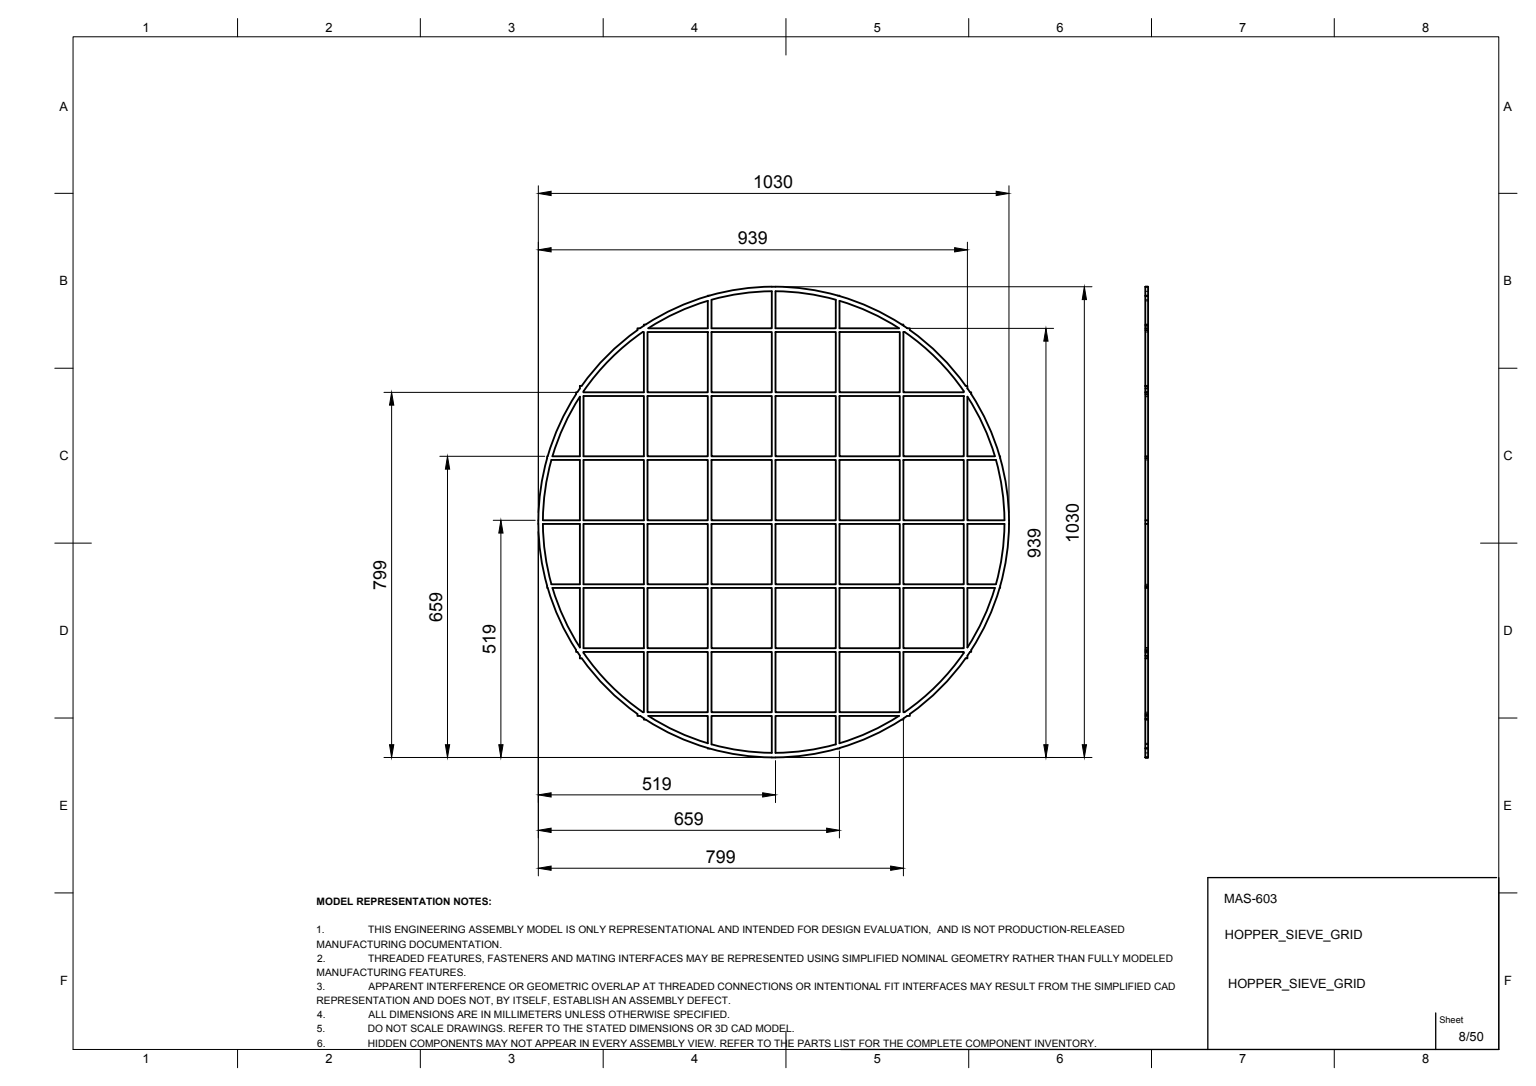
ISO-10303-21;
HEADER;
FILE_DESCRIPTION((''),'2;1');
FILE_NAME('HOPPER_SIEVE_GRID.step','2026-10-01T22:06:14-07:00',(''),(''),'','','');
FILE_SCHEMA (('AUTOMOTIVE_DESIGN { 1 0 10303 214 3 1 1 }'));
ENDSEC;
DATA;
#10=MECHANICAL_DESIGN_GEOMETRIC_PRESENTATION_REPRESENTATION('',(#984),#50440);
#894=SHAPE_REPRESENTATION_RELATIONSHIP('SRR','None',#50624,#939) ;
#939=ADVANCED_BREP_SHAPE_REPRESENTATION('',(#1040),#50393) ;
#984=STYLED_ITEM('',(#50885),#1040) ;
#1040=MANIFOLD_SOLID_BREP('HOPPER_SIEVE_GRID',#28632) ;
#1130=FACE_BOUND('',#4023,.T.) ;
#1131=FACE_BOUND('',#4024,.T.) ;
#1132=FACE_BOUND('',#4025,.T.) ;
#1133=FACE_BOUND('',#4026,.T.) ;
#1134=FACE_BOUND('',#4027,.T.) ;
#1135=FACE_BOUND('',#4028,.T.) ;
#1136=FACE_BOUND('',#4029,.T.) ;
#1137=FACE_BOUND('',#4030,.T.) ;
#1138=FACE_BOUND('',#4031,.T.) ;
#1139=FACE_BOUND('',#4032,.T.) ;
#1140=FACE_BOUND('',#4033,.T.) ;
#1141=FACE_BOUND('',#4034,.T.) ;
#1142=FACE_BOUND('',#4035,.T.) ;
#1143=FACE_BOUND('',#4036,.T.) ;
#1144=FACE_BOUND('',#4037,.T.) ;
#1145=FACE_BOUND('',#4038,.T.) ;
#1146=FACE_BOUND('',#4039,.T.) ;
#1147=FACE_BOUND('',#4040,.T.) ;
#1148=FACE_BOUND('',#4041,.T.) ;
#1149=FACE_BOUND('',#4042,.T.) ;
#1150=FACE_BOUND('',#4043,.T.) ;
#1151=FACE_BOUND('',#4044,.T.) ;
#1152=FACE_BOUND('',#4045,.T.) ;
#1153=FACE_BOUND('',#4046,.T.) ;
#1154=FACE_BOUND('',#4047,.T.) ;
#1155=FACE_BOUND('',#4048,.T.) ;
#1156=FACE_BOUND('',#4049,.T.) ;
#1157=FACE_BOUND('',#4050,.T.) ;
#1158=FACE_BOUND('',#4051,.T.) ;
#1159=FACE_BOUND('',#4052,.T.) ;
#1160=FACE_BOUND('',#4053,.T.) ;
#1161=FACE_BOUND('',#4054,.T.) ;
#1162=FACE_BOUND('',#4055,.T.) ;
#1163=FACE_BOUND('',#4056,.T.) ;
#1164=FACE_BOUND('',#4057,.T.) ;
#1165=FACE_BOUND('',#4058,.T.) ;
#1166=FACE_BOUND('',#4059,.T.) ;
#1167=FACE_BOUND('',#4060,.T.) ;
#1168=FACE_BOUND('',#4061,.T.) ;
#1169=FACE_BOUND('',#4062,.T.) ;
#1170=FACE_BOUND('',#4063,.T.) ;
#1171=FACE_BOUND('',#4064,.T.) ;
#1172=FACE_BOUND('',#4065,.T.) ;
#1173=FACE_BOUND('',#4066,.T.) ;
#1174=FACE_BOUND('',#4067,.T.) ;
#1175=FACE_BOUND('',#4068,.T.) ;
#1176=FACE_BOUND('',#4069,.T.) ;
#1177=FACE_BOUND('',#4070,.T.) ;
#1178=FACE_BOUND('',#4071,.T.) ;
#1179=FACE_BOUND('',#4072,.T.) ;
#1180=FACE_BOUND('',#4073,.T.) ;
#1181=FACE_BOUND('',#4074,.T.) ;
#1182=FACE_BOUND('',#4077,.T.) ;
#1183=FACE_BOUND('',#4078,.T.) ;
#1184=FACE_BOUND('',#4079,.T.) ;
#1185=FACE_BOUND('',#4080,.T.) ;
#1186=FACE_BOUND('',#4081,.T.) ;
#1187=FACE_BOUND('',#4082,.T.) ;
#1188=FACE_BOUND('',#4083,.T.) ;
#1189=FACE_BOUND('',#4084,.T.) ;
#1190=FACE_BOUND('',#4085,.T.) ;
#1191=FACE_BOUND('',#4086,.T.) ;
#1192=FACE_BOUND('',#4087,.T.) ;
#1193=FACE_BOUND('',#4088,.T.) ;
#1194=FACE_BOUND('',#4089,.T.) ;
#1195=FACE_BOUND('',#4090,.T.) ;
#1196=FACE_BOUND('',#4091,.T.) ;
#1197=FACE_BOUND('',#4092,.T.) ;
#1198=FACE_BOUND('',#4093,.T.) ;
#1199=FACE_BOUND('',#4094,.T.) ;
#1200=FACE_BOUND('',#4095,.T.) ;
#1201=FACE_BOUND('',#4096,.T.) ;
#1202=FACE_BOUND('',#4097,.T.) ;
#1203=FACE_BOUND('',#4098,.T.) ;
#1204=FACE_BOUND('',#4099,.T.) ;
#1205=FACE_BOUND('',#4100,.T.) ;
#1206=FACE_BOUND('',#4101,.T.) ;
#1207=FACE_BOUND('',#4102,.T.) ;
#1208=FACE_BOUND('',#4103,.T.) ;
#1209=FACE_BOUND('',#4104,.T.) ;
#1210=FACE_BOUND('',#4105,.T.) ;
#1211=FACE_BOUND('',#4106,.T.) ;
#1212=FACE_BOUND('',#4107,.T.) ;
#1213=FACE_BOUND('',#4108,.T.) ;
#1214=FACE_BOUND('',#4109,.T.) ;
#1215=FACE_BOUND('',#4110,.T.) ;
#1216=FACE_BOUND('',#4111,.T.) ;
#1217=FACE_BOUND('',#4112,.T.) ;
#1218=FACE_BOUND('',#4113,.T.) ;
#1219=FACE_BOUND('',#4114,.T.) ;
#1220=FACE_BOUND('',#4115,.T.) ;
#1221=FACE_BOUND('',#4116,.T.) ;
#1222=FACE_BOUND('',#4117,.T.) ;
#1223=FACE_BOUND('',#4118,.T.) ;
#1224=FACE_BOUND('',#4119,.T.) ;
#1225=FACE_BOUND('',#4120,.T.) ;
#1226=FACE_BOUND('',#4121,.T.) ;
#1227=FACE_BOUND('',#4122,.T.) ;
#1228=FACE_BOUND('',#4123,.T.) ;
#1229=FACE_BOUND('',#4124,.T.) ;
#1230=FACE_BOUND('',#4125,.T.) ;
#1231=FACE_BOUND('',#4126,.T.) ;
#1232=FACE_BOUND('',#4127,.T.) ;
#1233=FACE_BOUND('',#4128,.T.) ;
#1483=PLANE('',#29340) ;
#1484=PLANE('',#29341) ;
#1485=PLANE('',#29342) ;
#1486=PLANE('',#29343) ;
#1487=PLANE('',#29344) ;
#1488=PLANE('',#29345) ;
#1489=PLANE('',#29346) ;
#1490=PLANE('',#29347) ;
#1491=PLANE('',#29348) ;
#1492=PLANE('',#29349) ;
#1493=PLANE('',#29350) ;
#1494=PLANE('',#29351) ;
#1495=PLANE('',#29352) ;
#1496=PLANE('',#29353) ;
#1497=PLANE('',#29363) ;
#1498=PLANE('',#29364) ;
#1499=PLANE('',#29365) ;
#1500=PLANE('',#29366) ;
#1501=PLANE('',#29367) ;
#1502=PLANE('',#29368) ;
#1503=PLANE('',#29369) ;
#1504=PLANE('',#29370) ;
#1505=PLANE('',#29371) ;
#1506=PLANE('',#29419) ;
#1507=PLANE('',#29466) ;
#1508=PLANE('',#29467) ;
#1509=PLANE('',#29468) ;
#1510=PLANE('',#29469) ;
#1511=PLANE('',#29470) ;
#1512=PLANE('',#29471) ;
#1513=PLANE('',#29472) ;
#1514=PLANE('',#29473) ;
#1515=PLANE('',#29474) ;
#1516=PLANE('',#29475) ;
#1517=PLANE('',#29476) ;
#1518=PLANE('',#29477) ;
#1519=PLANE('',#29478) ;
#1520=PLANE('',#29479) ;
#1521=PLANE('',#29480) ;
#1522=PLANE('',#29481) ;
#1523=PLANE('',#29482) ;
#1524=PLANE('',#29485) ;
#1525=PLANE('',#29486) ;
#1526=PLANE('',#29487) ;
#1527=PLANE('',#29488) ;
#1528=PLANE('',#29489) ;
#1529=PLANE('',#29493) ;
#1530=PLANE('',#29494) ;
#1531=PLANE('',#29495) ;
#1532=PLANE('',#29496) ;
#1533=PLANE('',#29497) ;
#1534=PLANE('',#29498) ;
#1535=PLANE('',#29499) ;
#1536=PLANE('',#29500) ;
#1537=PLANE('',#29501) ;
#1538=PLANE('',#29502) ;
#1539=PLANE('',#29503) ;
#1540=PLANE('',#29504) ;
#1541=PLANE('',#29505) ;
#1542=PLANE('',#29506) ;
#1543=PLANE('',#29507) ;
#1544=PLANE('',#29508) ;
#1545=PLANE('',#29509) ;
#1546=PLANE('',#29511) ;
#1547=PLANE('',#29512) ;
#1548=PLANE('',#29513) ;
#1549=PLANE('',#29514) ;
#1550=PLANE('',#29515) ;
#1551=PLANE('',#29516) ;
#1552=PLANE('',#29517) ;
#1553=PLANE('',#29518) ;
#1554=PLANE('',#29520) ;
#1555=PLANE('',#29521) ;
#1556=PLANE('',#29522) ;
#1557=PLANE('',#29523) ;
#1558=PLANE('',#29524) ;
#1559=PLANE('',#29525) ;
#1560=PLANE('',#29526) ;
#1561=PLANE('',#29527) ;
#1562=PLANE('',#29528) ;
#1563=PLANE('',#29529) ;
#1564=PLANE('',#29530) ;
#1565=PLANE('',#29531) ;
#1566=PLANE('',#29532) ;
#1567=PLANE('',#29533) ;
#1568=PLANE('',#29534) ;
#1569=PLANE('',#29535) ;
#1570=PLANE('',#29536) ;
#1571=PLANE('',#29537) ;
#1572=PLANE('',#29538) ;
#1573=PLANE('',#29541) ;
#1574=PLANE('',#29544) ;
#1575=PLANE('',#29545) ;
#1576=PLANE('',#29546) ;
#1577=PLANE('',#29547) ;
#1578=PLANE('',#29548) ;
#1579=PLANE('',#29549) ;
#1580=PLANE('',#29550) ;
#1581=PLANE('',#29551) ;
#1582=PLANE('',#29552) ;
#1583=PLANE('',#29553) ;
#1584=PLANE('',#29554) ;
#1585=PLANE('',#29555) ;
#1586=PLANE('',#29556) ;
#1587=PLANE('',#29557) ;
#1588=PLANE('',#29558) ;
#1589=PLANE('',#29559) ;
#1590=PLANE('',#29560) ;
#1591=PLANE('',#29561) ;
#1592=PLANE('',#29562) ;
#1593=PLANE('',#29563) ;
#1594=PLANE('',#29564) ;
#1595=PLANE('',#29565) ;
#1596=PLANE('',#29570) ;
#1597=PLANE('',#29571) ;
#1598=PLANE('',#29572) ;
#1599=PLANE('',#29573) ;
#1600=PLANE('',#29574) ;
#1601=PLANE('',#29575) ;
#1602=PLANE('',#29576) ;
#1603=PLANE('',#29577) ;
#1604=PLANE('',#29578) ;
#1605=PLANE('',#29579) ;
#1606=PLANE('',#29580) ;
#1607=PLANE('',#29581) ;
#1608=PLANE('',#29582) ;
#1609=PLANE('',#29583) ;
#1610=PLANE('',#29584) ;
#1611=PLANE('',#29585) ;
#1612=PLANE('',#29586) ;
#1613=PLANE('',#29587) ;
#1614=PLANE('',#29588) ;
#1615=PLANE('',#29589) ;
#1616=PLANE('',#29590) ;
#1617=PLANE('',#29591) ;
#1618=PLANE('',#29592) ;
#1619=PLANE('',#29593) ;
#1620=PLANE('',#29597) ;
#1621=PLANE('',#29598) ;
#1622=PLANE('',#29599) ;
#1623=PLANE('',#29600) ;
#1624=PLANE('',#29601) ;
#1625=PLANE('',#29602) ;
#1626=PLANE('',#29605) ;
#1627=PLANE('',#29606) ;
#1628=PLANE('',#29607) ;
#1629=PLANE('',#29608) ;
#1630=PLANE('',#29609) ;
#1631=PLANE('',#29610) ;
#1632=PLANE('',#29611) ;
#1633=PLANE('',#29612) ;
#1634=PLANE('',#29613) ;
#1635=PLANE('',#29614) ;
#1636=PLANE('',#29615) ;
#1637=PLANE('',#29616) ;
#1638=PLANE('',#29617) ;
#1639=PLANE('',#29618) ;
#1640=PLANE('',#29619) ;
#1641=PLANE('',#29620) ;
#1642=PLANE('',#29621) ;
#1643=PLANE('',#29622) ;
#1644=PLANE('',#29625) ;
#1645=PLANE('',#29626) ;
#1646=PLANE('',#29630) ;
#1647=PLANE('',#29631) ;
#1648=PLANE('',#29632) ;
#1649=PLANE('',#29633) ;
#1650=PLANE('',#29634) ;
#1651=PLANE('',#29635) ;
#1652=PLANE('',#29636) ;
#1653=PLANE('',#29637) ;
#1654=PLANE('',#29638) ;
#1655=PLANE('',#29639) ;
#1656=PLANE('',#29640) ;
#1657=PLANE('',#29641) ;
#1658=PLANE('',#29642) ;
#1659=PLANE('',#29643) ;
#1660=PLANE('',#29644) ;
#1661=PLANE('',#29645) ;
#1662=PLANE('',#29646) ;
#1663=PLANE('',#29647) ;
#1664=PLANE('',#29648) ;
#1665=PLANE('',#29649) ;
#1666=PLANE('',#29650) ;
#1667=PLANE('',#29651) ;
#1668=PLANE('',#29653) ;
#1669=PLANE('',#29654) ;
#1670=PLANE('',#29658) ;
#1671=PLANE('',#29659) ;
#1672=PLANE('',#29660) ;
#1673=PLANE('',#29661) ;
#1674=PLANE('',#29662) ;
#1675=PLANE('',#29663) ;
#1676=PLANE('',#29664) ;
#1677=PLANE('',#29665) ;
#1678=PLANE('',#29666) ;
#1679=PLANE('',#29667) ;
#1680=PLANE('',#29668) ;
#1681=PLANE('',#29669) ;
#1682=PLANE('',#29670) ;
#1683=PLANE('',#29671) ;
#1684=PLANE('',#29672) ;
#1685=PLANE('',#29673) ;
#1686=PLANE('',#29675) ;
#1687=PLANE('',#29676) ;
#1688=PLANE('',#29679) ;
#1689=PLANE('',#29680) ;
#1690=PLANE('',#29681) ;
#1691=PLANE('',#29682) ;
#1692=PLANE('',#29683) ;
#1693=PLANE('',#29684) ;
#1694=PLANE('',#29685) ;
#1695=PLANE('',#29686) ;
#1696=PLANE('',#29687) ;
#1697=PLANE('',#29688) ;
#1698=PLANE('',#29689) ;
#1699=PLANE('',#29693) ;
#1700=PLANE('',#29694) ;
#1701=PLANE('',#29697) ;
#1702=PLANE('',#29698) ;
#1703=PLANE('',#29699) ;
#1704=PLANE('',#29700) ;
#1705=PLANE('',#29701) ;
#1706=PLANE('',#29702) ;
#1707=PLANE('',#29703) ;
#1708=PLANE('',#29704) ;
#1709=PLANE('',#29705) ;
#1710=PLANE('',#29707) ;
#1711=PLANE('',#29709) ;
#1712=PLANE('',#29710) ;
#1713=PLANE('',#29711) ;
#1714=PLANE('',#29712) ;
#1715=PLANE('',#29713) ;
#1716=PLANE('',#29714) ;
#1717=PLANE('',#29715) ;
#1718=PLANE('',#29717) ;
#1719=PLANE('',#29718) ;
#1720=PLANE('',#29719) ;
#1721=PLANE('',#29720) ;
#1722=PLANE('',#29721) ;
#1723=PLANE('',#29724) ;
#1724=PLANE('',#29725) ;
#1725=PLANE('',#29726) ;
#1726=PLANE('',#29727) ;
#1727=PLANE('',#29728) ;
#1728=PLANE('',#29729) ;
#2425=FACE_OUTER_BOUND('',#3997,.T.) ;
#2426=FACE_OUTER_BOUND('',#3998,.T.) ;
#2427=FACE_OUTER_BOUND('',#3999,.T.) ;
#2428=FACE_OUTER_BOUND('',#4000,.T.) ;
#2429=FACE_OUTER_BOUND('',#4001,.T.) ;
#2430=FACE_OUTER_BOUND('',#4002,.T.) ;
#2431=FACE_OUTER_BOUND('',#4003,.T.) ;
#2432=FACE_OUTER_BOUND('',#4004,.T.) ;
#2433=FACE_OUTER_BOUND('',#4005,.T.) ;
#2434=FACE_OUTER_BOUND('',#4006,.T.) ;
#2435=FACE_OUTER_BOUND('',#4007,.T.) ;
#2436=FACE_OUTER_BOUND('',#4008,.T.) ;
#2437=FACE_OUTER_BOUND('',#4009,.T.) ;
#2438=FACE_OUTER_BOUND('',#4010,.T.) ;
#2439=FACE_OUTER_BOUND('',#4011,.T.) ;
#2440=FACE_OUTER_BOUND('',#4012,.T.) ;
#2441=FACE_OUTER_BOUND('',#4013,.T.) ;
#2442=FACE_OUTER_BOUND('',#4014,.T.) ;
#2443=FACE_OUTER_BOUND('',#4015,.T.) ;
#2444=FACE_OUTER_BOUND('',#4016,.T.) ;
#2445=FACE_OUTER_BOUND('',#4017,.T.) ;
#2446=FACE_OUTER_BOUND('',#4018,.T.) ;
#2447=FACE_OUTER_BOUND('',#4019,.T.) ;
#2448=FACE_OUTER_BOUND('',#4020,.T.) ;
#2449=FACE_OUTER_BOUND('',#4021,.T.) ;
#2450=FACE_OUTER_BOUND('',#4022,.T.) ;
#2451=FACE_OUTER_BOUND('',#4075,.T.) ;
#2452=FACE_OUTER_BOUND('',#4076,.T.) ;
#2453=FACE_OUTER_BOUND('',#4129,.T.) ;
#2454=FACE_OUTER_BOUND('',#4130,.T.) ;
#2455=FACE_OUTER_BOUND('',#4131,.T.) ;
#2456=FACE_OUTER_BOUND('',#4132,.T.) ;
#2457=FACE_OUTER_BOUND('',#4133,.T.) ;
#2458=FACE_OUTER_BOUND('',#4134,.T.) ;
#2459=FACE_OUTER_BOUND('',#4135,.T.) ;
#2460=FACE_OUTER_BOUND('',#4136,.T.) ;
#2461=FACE_OUTER_BOUND('',#4137,.T.) ;
#2462=FACE_OUTER_BOUND('',#4138,.T.) ;
#2463=FACE_OUTER_BOUND('',#4139,.T.) ;
#2464=FACE_OUTER_BOUND('',#4140,.T.) ;
#2465=FACE_OUTER_BOUND('',#4141,.T.) ;
#2466=FACE_OUTER_BOUND('',#4142,.T.) ;
#2467=FACE_OUTER_BOUND('',#4143,.T.) ;
#2468=FACE_OUTER_BOUND('',#4144,.T.) ;
#2469=FACE_OUTER_BOUND('',#4145,.T.) ;
#2470=FACE_OUTER_BOUND('',#4146,.T.) ;
#2471=FACE_OUTER_BOUND('',#4147,.T.) ;
#2472=FACE_OUTER_BOUND('',#4148,.T.) ;
#2473=FACE_OUTER_BOUND('',#4149,.T.) ;
#2474=FACE_OUTER_BOUND('',#4150,.T.) ;
#2475=FACE_OUTER_BOUND('',#4151,.T.) ;
#2476=FACE_OUTER_BOUND('',#4152,.T.) ;
#2477=FACE_OUTER_BOUND('',#4153,.T.) ;
#2478=FACE_OUTER_BOUND('',#4154,.T.) ;
#2479=FACE_OUTER_BOUND('',#4155,.T.) ;
#2480=FACE_OUTER_BOUND('',#4156,.T.) ;
#2481=FACE_OUTER_BOUND('',#4157,.T.) ;
#2482=FACE_OUTER_BOUND('',#4158,.T.) ;
#2483=FACE_OUTER_BOUND('',#4159,.T.) ;
#2484=FACE_OUTER_BOUND('',#4160,.T.) ;
#2485=FACE_OUTER_BOUND('',#4161,.T.) ;
#2486=FACE_OUTER_BOUND('',#4162,.T.) ;
#2487=FACE_OUTER_BOUND('',#4163,.T.) ;
#2488=FACE_OUTER_BOUND('',#4164,.T.) ;
#2489=FACE_OUTER_BOUND('',#4165,.T.) ;
#2490=FACE_OUTER_BOUND('',#4166,.T.) ;
#2491=FACE_OUTER_BOUND('',#4167,.T.) ;
#2492=FACE_OUTER_BOUND('',#4168,.T.) ;
#2493=FACE_OUTER_BOUND('',#4169,.T.) ;
#2494=FACE_OUTER_BOUND('',#4170,.T.) ;
#2495=FACE_OUTER_BOUND('',#4171,.T.) ;
#2496=FACE_OUTER_BOUND('',#4172,.T.) ;
#2497=FACE_OUTER_BOUND('',#4173,.T.) ;
#2498=FACE_OUTER_BOUND('',#4174,.T.) ;
#2499=FACE_OUTER_BOUND('',#4175,.T.) ;
#2500=FACE_OUTER_BOUND('',#4176,.T.) ;
#2501=FACE_OUTER_BOUND('',#4177,.T.) ;
#2502=FACE_OUTER_BOUND('',#4178,.T.) ;
#2503=FACE_OUTER_BOUND('',#4179,.T.) ;
#2504=FACE_OUTER_BOUND('',#4180,.T.) ;
#2505=FACE_OUTER_BOUND('',#4181,.T.) ;
#2506=FACE_OUTER_BOUND('',#4182,.T.) ;
#2507=FACE_OUTER_BOUND('',#4183,.T.) ;
#2508=FACE_OUTER_BOUND('',#4184,.T.) ;
#2509=FACE_OUTER_BOUND('',#4185,.T.) ;
#2510=FACE_OUTER_BOUND('',#4186,.T.) ;
#2511=FACE_OUTER_BOUND('',#4187,.T.) ;
#2512=FACE_OUTER_BOUND('',#4188,.T.) ;
#2513=FACE_OUTER_BOUND('',#4189,.T.) ;
#2514=FACE_OUTER_BOUND('',#4190,.T.) ;
#2515=FACE_OUTER_BOUND('',#4191,.T.) ;
#2516=FACE_OUTER_BOUND('',#4192,.T.) ;
#2517=FACE_OUTER_BOUND('',#4193,.T.) ;
#2518=FACE_OUTER_BOUND('',#4194,.T.) ;
#2519=FACE_OUTER_BOUND('',#4195,.T.) ;
#2520=FACE_OUTER_BOUND('',#4196,.T.) ;
#2521=FACE_OUTER_BOUND('',#4197,.T.) ;
#2522=FACE_OUTER_BOUND('',#4198,.T.) ;
#2523=FACE_OUTER_BOUND('',#4199,.T.) ;
#2524=FACE_OUTER_BOUND('',#4200,.T.) ;
#2525=FACE_OUTER_BOUND('',#4201,.T.) ;
#2526=FACE_OUTER_BOUND('',#4202,.T.) ;
#2527=FACE_OUTER_BOUND('',#4203,.T.) ;
#2528=FACE_OUTER_BOUND('',#4204,.T.) ;
#2529=FACE_OUTER_BOUND('',#4205,.T.) ;
#2530=FACE_OUTER_BOUND('',#4206,.T.) ;
#2531=FACE_OUTER_BOUND('',#4207,.T.) ;
#2532=FACE_OUTER_BOUND('',#4208,.T.) ;
#2533=FACE_OUTER_BOUND('',#4209,.T.) ;
#2534=FACE_OUTER_BOUND('',#4210,.T.) ;
#2535=FACE_OUTER_BOUND('',#4211,.T.) ;
#2536=FACE_OUTER_BOUND('',#4212,.T.) ;
#2537=FACE_OUTER_BOUND('',#4213,.T.) ;
#2538=FACE_OUTER_BOUND('',#4214,.T.) ;
#2539=FACE_OUTER_BOUND('',#4215,.T.) ;
#2540=FACE_OUTER_BOUND('',#4216,.T.) ;
#2541=FACE_OUTER_BOUND('',#4217,.T.) ;
#2542=FACE_OUTER_BOUND('',#4218,.T.) ;
#2543=FACE_OUTER_BOUND('',#4219,.T.) ;
#2544=FACE_OUTER_BOUND('',#4220,.T.) ;
#2545=FACE_OUTER_BOUND('',#4221,.T.) ;
#2546=FACE_OUTER_BOUND('',#4222,.T.) ;
#2547=FACE_OUTER_BOUND('',#4223,.T.) ;
#2548=FACE_OUTER_BOUND('',#4224,.T.) ;
#2549=FACE_OUTER_BOUND('',#4225,.T.) ;
#2550=FACE_OUTER_BOUND('',#4226,.T.) ;
#2551=FACE_OUTER_BOUND('',#4227,.T.) ;
#2552=FACE_OUTER_BOUND('',#4228,.T.) ;
#2553=FACE_OUTER_BOUND('',#4229,.T.) ;
#2554=FACE_OUTER_BOUND('',#4230,.T.) ;
#2555=FACE_OUTER_BOUND('',#4231,.T.) ;
#2556=FACE_OUTER_BOUND('',#4232,.T.) ;
#2557=FACE_OUTER_BOUND('',#4233,.T.) ;
#2558=FACE_OUTER_BOUND('',#4234,.T.) ;
#2559=FACE_OUTER_BOUND('',#4235,.T.) ;
#2560=FACE_OUTER_BOUND('',#4236,.T.) ;
#2561=FACE_OUTER_BOUND('',#4237,.T.) ;
#2562=FACE_OUTER_BOUND('',#4238,.T.) ;
#2563=FACE_OUTER_BOUND('',#4239,.T.) ;
#2564=FACE_OUTER_BOUND('',#4240,.T.) ;
#2565=FACE_OUTER_BOUND('',#4241,.T.) ;
#2566=FACE_OUTER_BOUND('',#4242,.T.) ;
#2567=FACE_OUTER_BOUND('',#4243,.T.) ;
#2568=FACE_OUTER_BOUND('',#4244,.T.) ;
#2569=FACE_OUTER_BOUND('',#4245,.T.) ;
#2570=FACE_OUTER_BOUND('',#4246,.T.) ;
#2571=FACE_OUTER_BOUND('',#4247,.T.) ;
#2572=FACE_OUTER_BOUND('',#4248,.T.) ;
#2573=FACE_OUTER_BOUND('',#4249,.T.) ;
#2574=FACE_OUTER_BOUND('',#4250,.T.) ;
#2575=FACE_OUTER_BOUND('',#4251,.T.) ;
#2576=FACE_OUTER_BOUND('',#4252,.T.) ;
#2577=FACE_OUTER_BOUND('',#4253,.T.) ;
#2578=FACE_OUTER_BOUND('',#4254,.T.) ;
#2579=FACE_OUTER_BOUND('',#4255,.T.) ;
#2580=FACE_OUTER_BOUND('',#4256,.T.) ;
#2581=FACE_OUTER_BOUND('',#4257,.T.) ;
#2582=FACE_OUTER_BOUND('',#4258,.T.) ;
#2583=FACE_OUTER_BOUND('',#4259,.T.) ;
#2584=FACE_OUTER_BOUND('',#4260,.T.) ;
#2585=FACE_OUTER_BOUND('',#4261,.T.) ;
#2586=FACE_OUTER_BOUND('',#4262,.T.) ;
#2587=FACE_OUTER_BOUND('',#4263,.T.) ;
#2588=FACE_OUTER_BOUND('',#4264,.T.) ;
#2589=FACE_OUTER_BOUND('',#4265,.T.) ;
#2590=FACE_OUTER_BOUND('',#4266,.T.) ;
#2591=FACE_OUTER_BOUND('',#4267,.T.) ;
#2592=FACE_OUTER_BOUND('',#4268,.T.) ;
#2593=FACE_OUTER_BOUND('',#4269,.T.) ;
#2594=FACE_OUTER_BOUND('',#4270,.T.) ;
#2595=FACE_OUTER_BOUND('',#4271,.T.) ;
#2596=FACE_OUTER_BOUND('',#4272,.T.) ;
#2597=FACE_OUTER_BOUND('',#4273,.T.) ;
#2598=FACE_OUTER_BOUND('',#4274,.T.) ;
#2599=FACE_OUTER_BOUND('',#4275,.T.) ;
#2600=FACE_OUTER_BOUND('',#4276,.T.) ;
#2601=FACE_OUTER_BOUND('',#4277,.T.) ;
#2602=FACE_OUTER_BOUND('',#4278,.T.) ;
#2603=FACE_OUTER_BOUND('',#4279,.T.) ;
#2604=FACE_OUTER_BOUND('',#4280,.T.) ;
#2605=FACE_OUTER_BOUND('',#4281,.T.) ;
#2606=FACE_OUTER_BOUND('',#4282,.T.) ;
#2607=FACE_OUTER_BOUND('',#4283,.T.) ;
#2608=FACE_OUTER_BOUND('',#4284,.T.) ;
#2609=FACE_OUTER_BOUND('',#4285,.T.) ;
#2610=FACE_OUTER_BOUND('',#4286,.T.) ;
#2611=FACE_OUTER_BOUND('',#4287,.T.) ;
#2612=FACE_OUTER_BOUND('',#4288,.T.) ;
#2613=FACE_OUTER_BOUND('',#4289,.T.) ;
#2614=FACE_OUTER_BOUND('',#4290,.T.) ;
#2615=FACE_OUTER_BOUND('',#4291,.T.) ;
#2616=FACE_OUTER_BOUND('',#4292,.T.) ;
#2617=FACE_OUTER_BOUND('',#4293,.T.) ;
#2618=FACE_OUTER_BOUND('',#4294,.T.) ;
#2619=FACE_OUTER_BOUND('',#4295,.T.) ;
#2620=FACE_OUTER_BOUND('',#4296,.T.) ;
#2621=FACE_OUTER_BOUND('',#4297,.T.) ;
#2622=FACE_OUTER_BOUND('',#4298,.T.) ;
#2623=FACE_OUTER_BOUND('',#4299,.T.) ;
#2624=FACE_OUTER_BOUND('',#4300,.T.) ;
#2625=FACE_OUTER_BOUND('',#4301,.T.) ;
#2626=FACE_OUTER_BOUND('',#4302,.T.) ;
#2627=FACE_OUTER_BOUND('',#4303,.T.) ;
#2628=FACE_OUTER_BOUND('',#4304,.T.) ;
#2629=FACE_OUTER_BOUND('',#4305,.T.) ;
#2630=FACE_OUTER_BOUND('',#4306,.T.) ;
#2631=FACE_OUTER_BOUND('',#4307,.T.) ;
#2632=FACE_OUTER_BOUND('',#4308,.T.) ;
#2633=FACE_OUTER_BOUND('',#4309,.T.) ;
#2634=FACE_OUTER_BOUND('',#4310,.T.) ;
#2635=FACE_OUTER_BOUND('',#4311,.T.) ;
#2636=FACE_OUTER_BOUND('',#4312,.T.) ;
#2637=FACE_OUTER_BOUND('',#4313,.T.) ;
#2638=FACE_OUTER_BOUND('',#4314,.T.) ;
#2639=FACE_OUTER_BOUND('',#4315,.T.) ;
#2640=FACE_OUTER_BOUND('',#4316,.T.) ;
#2641=FACE_OUTER_BOUND('',#4317,.T.) ;
#2642=FACE_OUTER_BOUND('',#4318,.T.) ;
#2643=FACE_OUTER_BOUND('',#4319,.T.) ;
#2644=FACE_OUTER_BOUND('',#4320,.T.) ;
#2645=FACE_OUTER_BOUND('',#4321,.T.) ;
#2646=FACE_OUTER_BOUND('',#4322,.T.) ;
#2647=FACE_OUTER_BOUND('',#4323,.T.) ;
#2648=FACE_OUTER_BOUND('',#4324,.T.) ;
#2649=FACE_OUTER_BOUND('',#4325,.T.) ;
#2650=FACE_OUTER_BOUND('',#4326,.T.) ;
#2651=FACE_OUTER_BOUND('',#4327,.T.) ;
#2652=FACE_OUTER_BOUND('',#4328,.T.) ;
#2653=FACE_OUTER_BOUND('',#4329,.T.) ;
#2654=FACE_OUTER_BOUND('',#4330,.T.) ;
#2655=FACE_OUTER_BOUND('',#4331,.T.) ;
#2656=FACE_OUTER_BOUND('',#4332,.T.) ;
#2657=FACE_OUTER_BOUND('',#4333,.T.) ;
#2658=FACE_OUTER_BOUND('',#4334,.T.) ;
#2659=FACE_OUTER_BOUND('',#4335,.T.) ;
#2660=FACE_OUTER_BOUND('',#4336,.T.) ;
#2661=FACE_OUTER_BOUND('',#4337,.T.) ;
#2662=FACE_OUTER_BOUND('',#4338,.T.) ;
#2663=FACE_OUTER_BOUND('',#4339,.T.) ;
#2664=FACE_OUTER_BOUND('',#4340,.T.) ;
#2665=FACE_OUTER_BOUND('',#4341,.T.) ;
#2666=FACE_OUTER_BOUND('',#4342,.T.) ;
#2667=FACE_OUTER_BOUND('',#4343,.T.) ;
#2668=FACE_OUTER_BOUND('',#4344,.T.) ;
#2669=FACE_OUTER_BOUND('',#4345,.T.) ;
#2670=FACE_OUTER_BOUND('',#4346,.T.) ;
#2671=FACE_OUTER_BOUND('',#4347,.T.) ;
#2672=FACE_OUTER_BOUND('',#4348,.T.) ;
#2673=FACE_OUTER_BOUND('',#4349,.T.) ;
#2674=FACE_OUTER_BOUND('',#4350,.T.) ;
#2675=FACE_OUTER_BOUND('',#4351,.T.) ;
#2676=FACE_OUTER_BOUND('',#4352,.T.) ;
#2677=FACE_OUTER_BOUND('',#4353,.T.) ;
#2678=FACE_OUTER_BOUND('',#4354,.T.) ;
#2679=FACE_OUTER_BOUND('',#4355,.T.) ;
#2680=FACE_OUTER_BOUND('',#4356,.T.) ;
#2681=FACE_OUTER_BOUND('',#4357,.T.) ;
#2682=FACE_OUTER_BOUND('',#4358,.T.) ;
#2683=FACE_OUTER_BOUND('',#4359,.T.) ;
#2684=FACE_OUTER_BOUND('',#4360,.T.) ;
#2685=FACE_OUTER_BOUND('',#4361,.T.) ;
#2686=FACE_OUTER_BOUND('',#4362,.T.) ;
#2687=FACE_OUTER_BOUND('',#4363,.T.) ;
#2688=FACE_OUTER_BOUND('',#4364,.T.) ;
#2689=FACE_OUTER_BOUND('',#4365,.T.) ;
#2690=FACE_OUTER_BOUND('',#4366,.T.) ;
#2691=FACE_OUTER_BOUND('',#4367,.T.) ;
#2692=FACE_OUTER_BOUND('',#4368,.T.) ;
#2693=FACE_OUTER_BOUND('',#4369,.T.) ;
#2694=FACE_OUTER_BOUND('',#4370,.T.) ;
#2695=FACE_OUTER_BOUND('',#4371,.T.) ;
#2696=FACE_OUTER_BOUND('',#4372,.T.) ;
#2697=FACE_OUTER_BOUND('',#4373,.T.) ;
#2698=FACE_OUTER_BOUND('',#4374,.T.) ;
#2699=FACE_OUTER_BOUND('',#4375,.T.) ;
#2700=FACE_OUTER_BOUND('',#4376,.T.) ;
#2701=FACE_OUTER_BOUND('',#4377,.T.) ;
#2702=FACE_OUTER_BOUND('',#4378,.T.) ;
#2703=FACE_OUTER_BOUND('',#4379,.T.) ;
#2704=FACE_OUTER_BOUND('',#4380,.T.) ;
#2705=FACE_OUTER_BOUND('',#4381,.T.) ;
#2706=FACE_OUTER_BOUND('',#4382,.T.) ;
#2707=FACE_OUTER_BOUND('',#4383,.T.) ;
#2708=FACE_OUTER_BOUND('',#4384,.T.) ;
#2709=FACE_OUTER_BOUND('',#4385,.T.) ;
#2710=FACE_OUTER_BOUND('',#4386,.T.) ;
#2711=FACE_OUTER_BOUND('',#4387,.T.) ;
#2712=FACE_OUTER_BOUND('',#4388,.T.) ;
#2713=FACE_OUTER_BOUND('',#4389,.T.) ;
#2714=FACE_OUTER_BOUND('',#4390,.T.) ;
#2715=FACE_OUTER_BOUND('',#4391,.T.) ;
#2716=FACE_OUTER_BOUND('',#4392,.T.) ;
#2717=FACE_OUTER_BOUND('',#4393,.T.) ;
#2718=FACE_OUTER_BOUND('',#4394,.T.) ;
#3997=EDGE_LOOP('',(#19001,#19002,#19003,#19004)) ;
#3998=EDGE_LOOP('',(#19005,#19006,#19007,#19008)) ;
#3999=EDGE_LOOP('',(#19009,#19010,#19011,#19012)) ;
#4000=EDGE_LOOP('',(#19013,#19014,#19015,#19016)) ;
#4001=EDGE_LOOP('',(#19017,#19018,#19019,#19020)) ;
#4002=EDGE_LOOP('',(#19021,#19022,#19023,#19024)) ;
#4003=EDGE_LOOP('',(#19025,#19026,#19027,#19028)) ;
#4004=EDGE_LOOP('',(#19029,#19030,#19031,#19032)) ;
#4005=EDGE_LOOP('',(#19033,#19034,#19035,#19036)) ;
#4006=EDGE_LOOP('',(#19037,#19038,#19039,#19040)) ;
#4007=EDGE_LOOP('',(#19041,#19042,#19043,#19044)) ;
#4008=EDGE_LOOP('',(#19045,#19046,#19047,#19048)) ;
#4009=EDGE_LOOP('',(#19049,#19050,#19051,#19052)) ;
#4010=EDGE_LOOP('',(#19053,#19054,#19055,#19056)) ;
#4011=EDGE_LOOP('',(#19057,#19058,#19059,#19060)) ;
#4012=EDGE_LOOP('',(#19061,#19062,#19063,#19064)) ;
#4013=EDGE_LOOP('',(#19065,#19066,#19067,#19068)) ;
#4014=EDGE_LOOP('',(#19069,#19070,#19071,#19072)) ;
#4015=EDGE_LOOP('',(#19073,#19074,#19075,#19076)) ;
#4016=EDGE_LOOP('',(#19077,#19078,#19079,#19080)) ;
#4017=EDGE_LOOP('',(#19081,#19082,#19083,#19084)) ;
#4018=EDGE_LOOP('',(#19085,#19086,#19087,#19088)) ;
#4019=EDGE_LOOP('',(#19089,#19090,#19091,#19092)) ;
#4020=EDGE_LOOP('',(#19093,#19094,#19095,#19096)) ;
#4021=EDGE_LOOP('',(#19097,#19098,#19099,#19100)) ;
#4022=EDGE_LOOP('',(#19101,#19102,#19103,#19104,#19105,#19106,#19107,#19108,
#19109,#19110,#19111,#19112,#19113,#19114,#19115,#19116,#19117,#19118,#19119,
#19120,#19121,#19122,#19123,#19124,#19125,#19126,#19127,#19128,#19129,#19130,
#19131,#19132,#19133,#19134,#19135,#19136,#19137,#19138,#19139,#19140,#19141,
#19142,#19143,#19144,#19145,#19146,#19147,#19148,#19149,#19150,#19151,#19152,
#19153,#19154,#19155,#19156,#19157,#19158,#19159,#19160,#19161,#19162,#19163,
#19164,#19165,#19166,#19167,#19168,#19169,#19170,#19171,#19172,#19173,#19174,
#19175,#19176,#19177,#19178,#19179,#19180,#19181,#19182,#19183,#19184,#19185,
#19186,#19187,#19188)) ;
#4023=EDGE_LOOP('',(#19189,#19190,#19191)) ;
#4024=EDGE_LOOP('',(#19192,#19193,#19194,#19195)) ;
#4025=EDGE_LOOP('',(#19196,#19197,#19198,#19199)) ;
#4026=EDGE_LOOP('',(#19200,#19201,#19202)) ;
#4027=EDGE_LOOP('',(#19203,#19204,#19205,#19206)) ;
#4028=EDGE_LOOP('',(#19207,#19208,#19209,#19210)) ;
#4029=EDGE_LOOP('',(#19211,#19212,#19213,#19214)) ;
#4030=EDGE_LOOP('',(#19215,#19216,#19217,#19218)) ;
#4031=EDGE_LOOP('',(#19219,#19220,#19221,#19222,#19223)) ;
#4032=EDGE_LOOP('',(#19224,#19225,#19226)) ;
#4033=EDGE_LOOP('',(#19227,#19228,#19229,#19230)) ;
#4034=EDGE_LOOP('',(#19231,#19232,#19233,#19234)) ;
#4035=EDGE_LOOP('',(#19235,#19236,#19237,#19238)) ;
#4036=EDGE_LOOP('',(#19239,#19240,#19241,#19242)) ;
#4037=EDGE_LOOP('',(#19243,#19244,#19245,#19246)) ;
#4038=EDGE_LOOP('',(#19247,#19248,#19249,#19250)) ;
#4039=EDGE_LOOP('',(#19251,#19252,#19253,#19254,#19255)) ;
#4040=EDGE_LOOP('',(#19256,#19257,#19258)) ;
#4041=EDGE_LOOP('',(#19259,#19260,#19261,#19262)) ;
#4042=EDGE_LOOP('',(#19263,#19264,#19265,#19266)) ;
#4043=EDGE_LOOP('',(#19267,#19268,#19269,#19270)) ;
#4044=EDGE_LOOP('',(#19271,#19272,#19273,#19274)) ;
#4045=EDGE_LOOP('',(#19275,#19276,#19277,#19278)) ;
#4046=EDGE_LOOP('',(#19279,#19280,#19281,#19282)) ;
#4047=EDGE_LOOP('',(#19283,#19284,#19285,#19286)) ;
#4048=EDGE_LOOP('',(#19287,#19288,#19289,#19290)) ;
#4049=EDGE_LOOP('',(#19291,#19292,#19293,#19294)) ;
#4050=EDGE_LOOP('',(#19295,#19296,#19297)) ;
#4051=EDGE_LOOP('',(#19298,#19299,#19300,#19301,#19302)) ;
#4052=EDGE_LOOP('',(#19303,#19304,#19305)) ;
#4053=EDGE_LOOP('',(#19306,#19307,#19308,#19309)) ;
#4054=EDGE_LOOP('',(#19310,#19311,#19312)) ;
#4055=EDGE_LOOP('',(#19313,#19314,#19315,#19316)) ;
#4056=EDGE_LOOP('',(#19317,#19318,#19319,#19320)) ;
#4057=EDGE_LOOP('',(#19321,#19322,#19323,#19324)) ;
#4058=EDGE_LOOP('',(#19325,#19326,#19327,#19328)) ;
#4059=EDGE_LOOP('',(#19329,#19330,#19331,#19332)) ;
#4060=EDGE_LOOP('',(#19333,#19334,#19335,#19336)) ;
#4061=EDGE_LOOP('',(#19337,#19338,#19339,#19340)) ;
#4062=EDGE_LOOP('',(#19341,#19342,#19343)) ;
#4063=EDGE_LOOP('',(#19344,#19345,#19346,#19347)) ;
#4064=EDGE_LOOP('',(#19348,#19349,#19350,#19351)) ;
#4065=EDGE_LOOP('',(#19352,#19353,#19354,#19355)) ;
#4066=EDGE_LOOP('',(#19356,#19357,#19358,#19359)) ;
#4067=EDGE_LOOP('',(#19360,#19361,#19362,#19363)) ;
#4068=EDGE_LOOP('',(#19364,#19365,#19366,#19367)) ;
#4069=EDGE_LOOP('',(#19368,#19369,#19370,#19371)) ;
#4070=EDGE_LOOP('',(#19372,#19373,#19374,#19375)) ;
#4071=EDGE_LOOP('',(#19376,#19377,#19378,#19379)) ;
#4072=EDGE_LOOP('',(#19380,#19381,#19382,#19383)) ;
#4073=EDGE_LOOP('',(#19384,#19385,#19386,#19387)) ;
#4074=EDGE_LOOP('',(#19388,#19389,#19390,#19391,#19392)) ;
#4075=EDGE_LOOP('',(#19393,#19394,#19395,#19396)) ;
#4076=EDGE_LOOP('',(#19397,#19398,#19399,#19400,#19401,#19402,#19403,#19404,
#19405,#19406,#19407,#19408,#19409,#19410,#19411,#19412,#19413,#19414,#19415,
#19416,#19417,#19418,#19419,#19420,#19421,#19422,#19423,#19424,#19425,#19426,
#19427,#19428,#19429,#19430,#19431,#19432,#19433,#19434,#19435,#19436,#19437,
#19438,#19439,#19440,#19441,#19442,#19443,#19444,#19445,#19446,#19447,#19448,
#19449,#19450,#19451,#19452,#19453,#19454,#19455,#19456,#19457,#19458,#19459,
#19460,#19461,#19462,#19463,#19464,#19465,#19466,#19467,#19468,#19469,#19470,
#19471,#19472,#19473,#19474,#19475,#19476,#19477,#19478,#19479,#19480,#19481,
#19482,#19483,#19484)) ;
#4077=EDGE_LOOP('',(#19485,#19486,#19487,#19488)) ;
#4078=EDGE_LOOP('',(#19489,#19490,#19491,#19492)) ;
#4079=EDGE_LOOP('',(#19493,#19494,#19495,#19496)) ;
#4080=EDGE_LOOP('',(#19497,#19498,#19499,#19500)) ;
#4081=EDGE_LOOP('',(#19501,#19502,#19503,#19504,#19505)) ;
#4082=EDGE_LOOP('',(#19506,#19507,#19508,#19509)) ;
#4083=EDGE_LOOP('',(#19510,#19511,#19512,#19513)) ;
#4084=EDGE_LOOP('',(#19514,#19515,#19516)) ;
#4085=EDGE_LOOP('',(#19517,#19518,#19519,#19520,#19521)) ;
#4086=EDGE_LOOP('',(#19522,#19523,#19524)) ;
#4087=EDGE_LOOP('',(#19525,#19526,#19527,#19528,#19529)) ;
#4088=EDGE_LOOP('',(#19530,#19531,#19532,#19533)) ;
#4089=EDGE_LOOP('',(#19534,#19535,#19536,#19537)) ;
#4090=EDGE_LOOP('',(#19538,#19539,#19540,#19541)) ;
#4091=EDGE_LOOP('',(#19542,#19543,#19544,#19545)) ;
#4092=EDGE_LOOP('',(#19546,#19547,#19548)) ;
#4093=EDGE_LOOP('',(#19549,#19550,#19551,#19552)) ;
#4094=EDGE_LOOP('',(#19553,#19554,#19555,#19556)) ;
#4095=EDGE_LOOP('',(#19557,#19558,#19559,#19560)) ;
#4096=EDGE_LOOP('',(#19561,#19562,#19563,#19564)) ;
#4097=EDGE_LOOP('',(#19565,#19566,#19567,#19568)) ;
#4098=EDGE_LOOP('',(#19569,#19570,#19571,#19572)) ;
#4099=EDGE_LOOP('',(#19573,#19574,#19575,#19576)) ;
#4100=EDGE_LOOP('',(#19577,#19578,#19579,#19580)) ;
#4101=EDGE_LOOP('',(#19581,#19582,#19583,#19584,#19585)) ;
#4102=EDGE_LOOP('',(#19586,#19587,#19588)) ;
#4103=EDGE_LOOP('',(#19589,#19590,#19591,#19592)) ;
#4104=EDGE_LOOP('',(#19593,#19594,#19595)) ;
#4105=EDGE_LOOP('',(#19596,#19597,#19598,#19599)) ;
#4106=EDGE_LOOP('',(#19600,#19601,#19602,#19603)) ;
#4107=EDGE_LOOP('',(#19604,#19605,#19606,#19607)) ;
#4108=EDGE_LOOP('',(#19608,#19609,#19610,#19611)) ;
#4109=EDGE_LOOP('',(#19612,#19613,#19614,#19615)) ;
#4110=EDGE_LOOP('',(#19616,#19617,#19618,#19619)) ;
#4111=EDGE_LOOP('',(#19620,#19621,#19622,#19623)) ;
#4112=EDGE_LOOP('',(#19624,#19625,#19626,#19627)) ;
#4113=EDGE_LOOP('',(#19628,#19629,#19630,#19631)) ;
#4114=EDGE_LOOP('',(#19632,#19633,#19634)) ;
#4115=EDGE_LOOP('',(#19635,#19636,#19637,#19638)) ;
#4116=EDGE_LOOP('',(#19639,#19640,#19641,#19642)) ;
#4117=EDGE_LOOP('',(#19643,#19644,#19645,#19646)) ;
#4118=EDGE_LOOP('',(#19647,#19648,#19649,#19650)) ;
#4119=EDGE_LOOP('',(#19651,#19652,#19653,#19654)) ;
#4120=EDGE_LOOP('',(#19655,#19656,#19657,#19658)) ;
#4121=EDGE_LOOP('',(#19659,#19660,#19661,#19662)) ;
#4122=EDGE_LOOP('',(#19663,#19664,#19665,#19666)) ;
#4123=EDGE_LOOP('',(#19667,#19668,#19669,#19670)) ;
#4124=EDGE_LOOP('',(#19671,#19672,#19673)) ;
#4125=EDGE_LOOP('',(#19674,#19675,#19676)) ;
#4126=EDGE_LOOP('',(#19677,#19678,#19679,#19680)) ;
#4127=EDGE_LOOP('',(#19681,#19682,#19683,#19684)) ;
#4128=EDGE_LOOP('',(#19685,#19686,#19687,#19688)) ;
#4129=EDGE_LOOP('',(#19689,#19690,#19691,#19692)) ;
#4130=EDGE_LOOP('',(#19693,#19694,#19695,#19696)) ;
#4131=EDGE_LOOP('',(#19697,#19698,#19699,#19700)) ;
#4132=EDGE_LOOP('',(#19701,#19702,#19703,#19704)) ;
#4133=EDGE_LOOP('',(#19705,#19706,#19707,#19708)) ;
#4134=EDGE_LOOP('',(#19709,#19710,#19711,#19712)) ;
#4135=EDGE_LOOP('',(#19713,#19714,#19715,#19716)) ;
#4136=EDGE_LOOP('',(#19717,#19718,#19719,#19720)) ;
#4137=EDGE_LOOP('',(#19721,#19722,#19723,#19724)) ;
#4138=EDGE_LOOP('',(#19725,#19726,#19727,#19728)) ;
#4139=EDGE_LOOP('',(#19729,#19730,#19731,#19732)) ;
#4140=EDGE_LOOP('',(#19733,#19734,#19735,#19736)) ;
#4141=EDGE_LOOP('',(#19737,#19738,#19739,#19740)) ;
#4142=EDGE_LOOP('',(#19741,#19742,#19743,#19744)) ;
#4143=EDGE_LOOP('',(#19745,#19746,#19747,#19748)) ;
#4144=EDGE_LOOP('',(#19749,#19750,#19751,#19752)) ;
#4145=EDGE_LOOP('',(#19753,#19754,#19755,#19756)) ;
#4146=EDGE_LOOP('',(#19757,#19758,#19759,#19760)) ;
#4147=EDGE_LOOP('',(#19761,#19762,#19763,#19764)) ;
#4148=EDGE_LOOP('',(#19765,#19766,#19767,#19768)) ;
#4149=EDGE_LOOP('',(#19769,#19770,#19771,#19772)) ;
#4150=EDGE_LOOP('',(#19773,#19774,#19775,#19776)) ;
#4151=EDGE_LOOP('',(#19777,#19778,#19779,#19780)) ;
#4152=EDGE_LOOP('',(#19781,#19782,#19783,#19784)) ;
#4153=EDGE_LOOP('',(#19785,#19786,#19787,#19788)) ;
#4154=EDGE_LOOP('',(#19789,#19790,#19791,#19792)) ;
#4155=EDGE_LOOP('',(#19793,#19794,#19795,#19796)) ;
#4156=EDGE_LOOP('',(#19797,#19798,#19799,#19800)) ;
#4157=EDGE_LOOP('',(#19801,#19802,#19803,#19804)) ;
#4158=EDGE_LOOP('',(#19805,#19806,#19807,#19808)) ;
#4159=EDGE_LOOP('',(#19809,#19810,#19811,#19812)) ;
#4160=EDGE_LOOP('',(#19813,#19814,#19815,#19816)) ;
#4161=EDGE_LOOP('',(#19817,#19818,#19819,#19820)) ;
#4162=EDGE_LOOP('',(#19821,#19822,#19823,#19824)) ;
#4163=EDGE_LOOP('',(#19825,#19826,#19827,#19828)) ;
#4164=EDGE_LOOP('',(#19829,#19830,#19831,#19832)) ;
#4165=EDGE_LOOP('',(#19833,#19834,#19835,#19836)) ;
#4166=EDGE_LOOP('',(#19837,#19838,#19839,#19840)) ;
#4167=EDGE_LOOP('',(#19841,#19842,#19843,#19844)) ;
#4168=EDGE_LOOP('',(#19845,#19846,#19847,#19848)) ;
#4169=EDGE_LOOP('',(#19849,#19850,#19851,#19852)) ;
#4170=EDGE_LOOP('',(#19853,#19854,#19855,#19856)) ;
#4171=EDGE_LOOP('',(#19857,#19858,#19859,#19860)) ;
#4172=EDGE_LOOP('',(#19861,#19862,#19863,#19864)) ;
#4173=EDGE_LOOP('',(#19865,#19866,#19867,#19868)) ;
#4174=EDGE_LOOP('',(#19869,#19870,#19871,#19872)) ;
#4175=EDGE_LOOP('',(#19873,#19874,#19875,#19876)) ;
#4176=EDGE_LOOP('',(#19877,#19878,#19879,#19880)) ;
#4177=EDGE_LOOP('',(#19881,#19882,#19883,#19884)) ;
#4178=EDGE_LOOP('',(#19885,#19886,#19887,#19888)) ;
#4179=EDGE_LOOP('',(#19889,#19890,#19891,#19892)) ;
#4180=EDGE_LOOP('',(#19893,#19894,#19895,#19896)) ;
#4181=EDGE_LOOP('',(#19897,#19898,#19899,#19900)) ;
#4182=EDGE_LOOP('',(#19901,#19902,#19903,#19904)) ;
#4183=EDGE_LOOP('',(#19905,#19906,#19907,#19908)) ;
#4184=EDGE_LOOP('',(#19909,#19910,#19911,#19912)) ;
#4185=EDGE_LOOP('',(#19913,#19914,#19915,#19916)) ;
#4186=EDGE_LOOP('',(#19917,#19918,#19919,#19920)) ;
#4187=EDGE_LOOP('',(#19921,#19922,#19923,#19924)) ;
#4188=EDGE_LOOP('',(#19925,#19926,#19927,#19928)) ;
#4189=EDGE_LOOP('',(#19929,#19930,#19931,#19932)) ;
#4190=EDGE_LOOP('',(#19933,#19934,#19935,#19936)) ;
#4191=EDGE_LOOP('',(#19937,#19938,#19939,#19940)) ;
#4192=EDGE_LOOP('',(#19941,#19942,#19943,#19944)) ;
#4193=EDGE_LOOP('',(#19945,#19946,#19947,#19948)) ;
#4194=EDGE_LOOP('',(#19949,#19950,#19951,#19952)) ;
#4195=EDGE_LOOP('',(#19953,#19954,#19955,#19956)) ;
#4196=EDGE_LOOP('',(#19957,#19958,#19959,#19960)) ;
#4197=EDGE_LOOP('',(#19961,#19962,#19963,#19964)) ;
#4198=EDGE_LOOP('',(#19965,#19966,#19967,#19968)) ;
#4199=EDGE_LOOP('',(#19969,#19970,#19971,#19972)) ;
#4200=EDGE_LOOP('',(#19973,#19974,#19975,#19976)) ;
#4201=EDGE_LOOP('',(#19977,#19978,#19979,#19980)) ;
#4202=EDGE_LOOP('',(#19981,#19982,#19983,#19984)) ;
#4203=EDGE_LOOP('',(#19985,#19986,#19987,#19988)) ;
#4204=EDGE_LOOP('',(#19989,#19990,#19991,#19992)) ;
#4205=EDGE_LOOP('',(#19993,#19994,#19995,#19996)) ;
#4206=EDGE_LOOP('',(#19997,#19998,#19999,#20000)) ;
#4207=EDGE_LOOP('',(#20001,#20002,#20003,#20004)) ;
#4208=EDGE_LOOP('',(#20005,#20006,#20007,#20008)) ;
#4209=EDGE_LOOP('',(#20009,#20010,#20011,#20012)) ;
#4210=EDGE_LOOP('',(#20013,#20014,#20015,#20016)) ;
#4211=EDGE_LOOP('',(#20017,#20018,#20019,#20020)) ;
#4212=EDGE_LOOP('',(#20021,#20022,#20023,#20024)) ;
#4213=EDGE_LOOP('',(#20025,#20026,#20027,#20028)) ;
#4214=EDGE_LOOP('',(#20029,#20030,#20031,#20032)) ;
#4215=EDGE_LOOP('',(#20033,#20034,#20035,#20036)) ;
#4216=EDGE_LOOP('',(#20037,#20038,#20039,#20040)) ;
#4217=EDGE_LOOP('',(#20041,#20042,#20043,#20044)) ;
#4218=EDGE_LOOP('',(#20045,#20046,#20047,#20048)) ;
#4219=EDGE_LOOP('',(#20049,#20050,#20051,#20052)) ;
#4220=EDGE_LOOP('',(#20053,#20054,#20055,#20056)) ;
#4221=EDGE_LOOP('',(#20057,#20058,#20059,#20060)) ;
#4222=EDGE_LOOP('',(#20061,#20062,#20063,#20064)) ;
#4223=EDGE_LOOP('',(#20065,#20066,#20067,#20068)) ;
#4224=EDGE_LOOP('',(#20069,#20070,#20071,#20072)) ;
#4225=EDGE_LOOP('',(#20073,#20074,#20075,#20076)) ;
#4226=EDGE_LOOP('',(#20077,#20078,#20079,#20080)) ;
#4227=EDGE_LOOP('',(#20081,#20082,#20083,#20084)) ;
#4228=EDGE_LOOP('',(#20085,#20086,#20087,#20088)) ;
#4229=EDGE_LOOP('',(#20089,#20090,#20091,#20092)) ;
#4230=EDGE_LOOP('',(#20093,#20094,#20095,#20096)) ;
#4231=EDGE_LOOP('',(#20097,#20098,#20099,#20100)) ;
#4232=EDGE_LOOP('',(#20101,#20102,#20103,#20104)) ;
#4233=EDGE_LOOP('',(#20105,#20106,#20107,#20108)) ;
#4234=EDGE_LOOP('',(#20109,#20110,#20111,#20112)) ;
#4235=EDGE_LOOP('',(#20113,#20114,#20115,#20116)) ;
#4236=EDGE_LOOP('',(#20117,#20118,#20119,#20120)) ;
#4237=EDGE_LOOP('',(#20121,#20122,#20123,#20124)) ;
#4238=EDGE_LOOP('',(#20125,#20126,#20127,#20128)) ;
#4239=EDGE_LOOP('',(#20129,#20130,#20131,#20132)) ;
#4240=EDGE_LOOP('',(#20133,#20134,#20135,#20136)) ;
#4241=EDGE_LOOP('',(#20137,#20138,#20139,#20140)) ;
#4242=EDGE_LOOP('',(#20141,#20142,#20143,#20144)) ;
#4243=EDGE_LOOP('',(#20145,#20146,#20147,#20148)) ;
#4244=EDGE_LOOP('',(#20149,#20150,#20151,#20152)) ;
#4245=EDGE_LOOP('',(#20153,#20154,#20155,#20156)) ;
#4246=EDGE_LOOP('',(#20157,#20158,#20159,#20160)) ;
#4247=EDGE_LOOP('',(#20161,#20162,#20163,#20164)) ;
#4248=EDGE_LOOP('',(#20165,#20166,#20167,#20168)) ;
#4249=EDGE_LOOP('',(#20169,#20170,#20171,#20172)) ;
#4250=EDGE_LOOP('',(#20173,#20174,#20175,#20176)) ;
#4251=EDGE_LOOP('',(#20177,#20178,#20179,#20180)) ;
#4252=EDGE_LOOP('',(#20181,#20182,#20183,#20184)) ;
#4253=EDGE_LOOP('',(#20185,#20186,#20187,#20188)) ;
#4254=EDGE_LOOP('',(#20189,#20190,#20191,#20192)) ;
#4255=EDGE_LOOP('',(#20193,#20194,#20195,#20196)) ;
#4256=EDGE_LOOP('',(#20197,#20198,#20199,#20200)) ;
#4257=EDGE_LOOP('',(#20201,#20202,#20203,#20204)) ;
#4258=EDGE_LOOP('',(#20205,#20206,#20207,#20208)) ;
#4259=EDGE_LOOP('',(#20209,#20210,#20211,#20212)) ;
#4260=EDGE_LOOP('',(#20213,#20214,#20215,#20216)) ;
#4261=EDGE_LOOP('',(#20217,#20218,#20219,#20220)) ;
#4262=EDGE_LOOP('',(#20221,#20222,#20223,#20224)) ;
#4263=EDGE_LOOP('',(#20225,#20226,#20227,#20228)) ;
#4264=EDGE_LOOP('',(#20229,#20230,#20231,#20232)) ;
#4265=EDGE_LOOP('',(#20233,#20234,#20235,#20236)) ;
#4266=EDGE_LOOP('',(#20237,#20238,#20239,#20240)) ;
#4267=EDGE_LOOP('',(#20241,#20242,#20243,#20244)) ;
#4268=EDGE_LOOP('',(#20245,#20246,#20247,#20248)) ;
#4269=EDGE_LOOP('',(#20249,#20250,#20251,#20252)) ;
#4270=EDGE_LOOP('',(#20253,#20254,#20255,#20256)) ;
#4271=EDGE_LOOP('',(#20257,#20258,#20259,#20260)) ;
#4272=EDGE_LOOP('',(#20261,#20262,#20263,#20264)) ;
#4273=EDGE_LOOP('',(#20265,#20266,#20267,#20268)) ;
#4274=EDGE_LOOP('',(#20269,#20270,#20271,#20272)) ;
#4275=EDGE_LOOP('',(#20273,#20274,#20275,#20276)) ;
#4276=EDGE_LOOP('',(#20277,#20278,#20279,#20280)) ;
#4277=EDGE_LOOP('',(#20281,#20282,#20283,#20284)) ;
#4278=EDGE_LOOP('',(#20285,#20286,#20287,#20288)) ;
#4279=EDGE_LOOP('',(#20289,#20290,#20291,#20292)) ;
#4280=EDGE_LOOP('',(#20293,#20294,#20295,#20296)) ;
#4281=EDGE_LOOP('',(#20297,#20298,#20299,#20300)) ;
#4282=EDGE_LOOP('',(#20301,#20302,#20303,#20304)) ;
#4283=EDGE_LOOP('',(#20305,#20306,#20307,#20308)) ;
#4284=EDGE_LOOP('',(#20309,#20310,#20311,#20312)) ;
#4285=EDGE_LOOP('',(#20313,#20314,#20315,#20316)) ;
#4286=EDGE_LOOP('',(#20317,#20318,#20319,#20320)) ;
#4287=EDGE_LOOP('',(#20321,#20322,#20323,#20324)) ;
#4288=EDGE_LOOP('',(#20325,#20326,#20327,#20328)) ;
#4289=EDGE_LOOP('',(#20329,#20330,#20331,#20332)) ;
#4290=EDGE_LOOP('',(#20333,#20334,#20335,#20336)) ;
#4291=EDGE_LOOP('',(#20337,#20338,#20339,#20340)) ;
#4292=EDGE_LOOP('',(#20341,#20342,#20343,#20344)) ;
#4293=EDGE_LOOP('',(#20345,#20346,#20347,#20348)) ;
#4294=EDGE_LOOP('',(#20349,#20350,#20351,#20352)) ;
#4295=EDGE_LOOP('',(#20353,#20354,#20355,#20356)) ;
#4296=EDGE_LOOP('',(#20357,#20358,#20359,#20360)) ;
#4297=EDGE_LOOP('',(#20361,#20362,#20363,#20364)) ;
#4298=EDGE_LOOP('',(#20365,#20366,#20367,#20368)) ;
#4299=EDGE_LOOP('',(#20369,#20370,#20371,#20372)) ;
#4300=EDGE_LOOP('',(#20373,#20374,#20375,#20376)) ;
#4301=EDGE_LOOP('',(#20377,#20378,#20379,#20380)) ;
#4302=EDGE_LOOP('',(#20381,#20382,#20383,#20384)) ;
#4303=EDGE_LOOP('',(#20385,#20386,#20387,#20388)) ;
#4304=EDGE_LOOP('',(#20389,#20390,#20391,#20392)) ;
#4305=EDGE_LOOP('',(#20393,#20394,#20395,#20396)) ;
#4306=EDGE_LOOP('',(#20397,#20398,#20399,#20400)) ;
#4307=EDGE_LOOP('',(#20401,#20402,#20403,#20404)) ;
#4308=EDGE_LOOP('',(#20405,#20406,#20407,#20408)) ;
#4309=EDGE_LOOP('',(#20409,#20410,#20411,#20412)) ;
#4310=EDGE_LOOP('',(#20413,#20414,#20415,#20416)) ;
#4311=EDGE_LOOP('',(#20417,#20418,#20419,#20420)) ;
#4312=EDGE_LOOP('',(#20421,#20422,#20423,#20424)) ;
#4313=EDGE_LOOP('',(#20425,#20426,#20427,#20428)) ;
#4314=EDGE_LOOP('',(#20429,#20430,#20431,#20432)) ;
#4315=EDGE_LOOP('',(#20433,#20434,#20435,#20436)) ;
#4316=EDGE_LOOP('',(#20437,#20438,#20439,#20440)) ;
#4317=EDGE_LOOP('',(#20441,#20442,#20443,#20444)) ;
#4318=EDGE_LOOP('',(#20445,#20446,#20447,#20448)) ;
#4319=EDGE_LOOP('',(#20449,#20450,#20451,#20452)) ;
#4320=EDGE_LOOP('',(#20453,#20454,#20455,#20456)) ;
#4321=EDGE_LOOP('',(#20457,#20458,#20459,#20460)) ;
#4322=EDGE_LOOP('',(#20461,#20462,#20463,#20464)) ;
#4323=EDGE_LOOP('',(#20465,#20466,#20467,#20468)) ;
#4324=EDGE_LOOP('',(#20469,#20470,#20471,#20472)) ;
#4325=EDGE_LOOP('',(#20473,#20474,#20475,#20476)) ;
#4326=EDGE_LOOP('',(#20477,#20478,#20479,#20480)) ;
#4327=EDGE_LOOP('',(#20481,#20482,#20483,#20484)) ;
#4328=EDGE_LOOP('',(#20485,#20486,#20487,#20488)) ;
#4329=EDGE_LOOP('',(#20489,#20490,#20491,#20492)) ;
#4330=EDGE_LOOP('',(#20493,#20494,#20495,#20496)) ;
#4331=EDGE_LOOP('',(#20497,#20498,#20499,#20500)) ;
#4332=EDGE_LOOP('',(#20501,#20502,#20503,#20504)) ;
#4333=EDGE_LOOP('',(#20505,#20506,#20507,#20508)) ;
#4334=EDGE_LOOP('',(#20509,#20510,#20511,#20512)) ;
#4335=EDGE_LOOP('',(#20513,#20514,#20515,#20516)) ;
#4336=EDGE_LOOP('',(#20517,#20518,#20519,#20520)) ;
#4337=EDGE_LOOP('',(#20521,#20522,#20523,#20524)) ;
#4338=EDGE_LOOP('',(#20525,#20526,#20527,#20528)) ;
#4339=EDGE_LOOP('',(#20529,#20530,#20531,#20532)) ;
#4340=EDGE_LOOP('',(#20533,#20534,#20535,#20536)) ;
#4341=EDGE_LOOP('',(#20537,#20538,#20539,#20540)) ;
#4342=EDGE_LOOP('',(#20541,#20542,#20543,#20544)) ;
#4343=EDGE_LOOP('',(#20545,#20546,#20547,#20548)) ;
#4344=EDGE_LOOP('',(#20549,#20550,#20551,#20552)) ;
#4345=EDGE_LOOP('',(#20553,#20554,#20555,#20556)) ;
#4346=EDGE_LOOP('',(#20557,#20558,#20559,#20560)) ;
#4347=EDGE_LOOP('',(#20561,#20562,#20563,#20564)) ;
#4348=EDGE_LOOP('',(#20565,#20566,#20567,#20568)) ;
#4349=EDGE_LOOP('',(#20569,#20570,#20571,#20572)) ;
#4350=EDGE_LOOP('',(#20573,#20574,#20575,#20576)) ;
#4351=EDGE_LOOP('',(#20577,#20578,#20579,#20580)) ;
#4352=EDGE_LOOP('',(#20581,#20582,#20583,#20584)) ;
#4353=EDGE_LOOP('',(#20585,#20586,#20587,#20588)) ;
#4354=EDGE_LOOP('',(#20589,#20590,#20591,#20592)) ;
#4355=EDGE_LOOP('',(#20593,#20594,#20595,#20596)) ;
#4356=EDGE_LOOP('',(#20597,#20598,#20599,#20600)) ;
#4357=EDGE_LOOP('',(#20601,#20602,#20603,#20604)) ;
#4358=EDGE_LOOP('',(#20605,#20606,#20607,#20608)) ;
#4359=EDGE_LOOP('',(#20609,#20610,#20611,#20612)) ;
#4360=EDGE_LOOP('',(#20613,#20614,#20615,#20616)) ;
#4361=EDGE_LOOP('',(#20617,#20618,#20619,#20620)) ;
#4362=EDGE_LOOP('',(#20621,#20622,#20623,#20624)) ;
#4363=EDGE_LOOP('',(#20625,#20626,#20627,#20628)) ;
#4364=EDGE_LOOP('',(#20629,#20630,#20631,#20632)) ;
#4365=EDGE_LOOP('',(#20633,#20634,#20635,#20636)) ;
#4366=EDGE_LOOP('',(#20637,#20638,#20639,#20640)) ;
#4367=EDGE_LOOP('',(#20641,#20642,#20643,#20644)) ;
#4368=EDGE_LOOP('',(#20645,#20646,#20647,#20648)) ;
#4369=EDGE_LOOP('',(#20649,#20650,#20651,#20652)) ;
#4370=EDGE_LOOP('',(#20653,#20654,#20655,#20656)) ;
#4371=EDGE_LOOP('',(#20657,#20658,#20659,#20660)) ;
#4372=EDGE_LOOP('',(#20661,#20662,#20663,#20664)) ;
#4373=EDGE_LOOP('',(#20665,#20666,#20667,#20668)) ;
#4374=EDGE_LOOP('',(#20669,#20670,#20671,#20672)) ;
#4375=EDGE_LOOP('',(#20673,#20674,#20675,#20676)) ;
#4376=EDGE_LOOP('',(#20677,#20678,#20679,#20680)) ;
#4377=EDGE_LOOP('',(#20681,#20682,#20683,#20684)) ;
#4378=EDGE_LOOP('',(#20685,#20686,#20687,#20688)) ;
#4379=EDGE_LOOP('',(#20689,#20690,#20691,#20692)) ;
#4380=EDGE_LOOP('',(#20693,#20694,#20695,#20696)) ;
#4381=EDGE_LOOP('',(#20697,#20698,#20699,#20700)) ;
#4382=EDGE_LOOP('',(#20701,#20702,#20703,#20704)) ;
#4383=EDGE_LOOP('',(#20705,#20706,#20707,#20708)) ;
#4384=EDGE_LOOP('',(#20709,#20710,#20711,#20712)) ;
#4385=EDGE_LOOP('',(#20713,#20714,#20715,#20716)) ;
#4386=EDGE_LOOP('',(#20717,#20718,#20719,#20720)) ;
#4387=EDGE_LOOP('',(#20721,#20722,#20723,#20724)) ;
#4388=EDGE_LOOP('',(#20725,#20726,#20727,#20728)) ;
#4389=EDGE_LOOP('',(#20729,#20730,#20731,#20732)) ;
#4390=EDGE_LOOP('',(#20733,#20734,#20735,#20736)) ;
#4391=EDGE_LOOP('',(#20737,#20738,#20739,#20740)) ;
#4392=EDGE_LOOP('',(#20741,#20742,#20743,#20744)) ;
#4393=EDGE_LOOP('',(#20745,#20746,#20747,#20748)) ;
#4394=EDGE_LOOP('',(#20749,#20750,#20751,#20752)) ;
#5895=LINE('',#41690,#8367) ;
#5896=LINE('',#41692,#8368) ;
#5897=LINE('',#41694,#8369) ;
#5898=LINE('',#41695,#8370) ;
#5899=LINE('',#41699,#8371) ;
#5900=LINE('',#41701,#8372) ;
#5901=LINE('',#41703,#8373) ;
#5902=LINE('',#41704,#8374) ;
#5903=LINE('',#41708,#8375) ;
#5904=LINE('',#41710,#8376) ;
#5905=LINE('',#41712,#8377) ;
#5906=LINE('',#41713,#8378) ;
#5907=LINE('',#41717,#8379) ;
#5908=LINE('',#41719,#8380) ;
#5909=LINE('',#41721,#8381) ;
#5910=LINE('',#41722,#8382) ;
#5911=LINE('',#41726,#8383) ;
#5912=LINE('',#41728,#8384) ;
#5913=LINE('',#41730,#8385) ;
#5914=LINE('',#41731,#8386) ;
#5915=LINE('',#41735,#8387) ;
#5916=LINE('',#41737,#8388) ;
#5917=LINE('',#41739,#8389) ;
#5918=LINE('',#41740,#8390) ;
#5919=LINE('',#41744,#8391) ;
#5920=LINE('',#41746,#8392) ;
#5921=LINE('',#41748,#8393) ;
#5922=LINE('',#41749,#8394) ;
#5923=LINE('',#41753,#8395) ;
#5924=LINE('',#41755,#8396) ;
#5925=LINE('',#41757,#8397) ;
#5926=LINE('',#41758,#8398) ;
#5927=LINE('',#41762,#8399) ;
#5928=LINE('',#41764,#8400) ;
#5929=LINE('',#41766,#8401) ;
#5930=LINE('',#41767,#8402) ;
#5931=LINE('',#41771,#8403) ;
#5932=LINE('',#41773,#8404) ;
#5933=LINE('',#41775,#8405) ;
#5934=LINE('',#41776,#8406) ;
#5935=LINE('',#41780,#8407) ;
#5936=LINE('',#41782,#8408) ;
#5937=LINE('',#41784,#8409) ;
#5938=LINE('',#41785,#8410) ;
#5939=LINE('',#41789,#8411) ;
#5940=LINE('',#41791,#8412) ;
#5941=LINE('',#41793,#8413) ;
#5942=LINE('',#41794,#8414) ;
#5943=LINE('',#41798,#8415) ;
#5944=LINE('',#41799,#8416) ;
#5945=LINE('',#41800,#8417) ;
#5946=LINE('',#41804,#8418) ;
#5947=LINE('',#41805,#8419) ;
#5948=LINE('',#41806,#8420) ;
#5949=LINE('',#41811,#8421) ;
#5950=LINE('',#41817,#8422) ;
#5951=LINE('',#41823,#8423) ;
#5952=LINE('',#41827,#8424) ;
#5953=LINE('',#41829,#8425) ;
#5954=LINE('',#41830,#8426) ;
#5955=LINE('',#41833,#8427) ;
#5956=LINE('',#41835,#8428) ;
#5957=LINE('',#41836,#8429) ;
#5958=LINE('',#41839,#8430) ;
#5959=LINE('',#41841,#8431) ;
#5960=LINE('',#41842,#8432) ;
#5961=LINE('',#41845,#8433) ;
#5962=LINE('',#41847,#8434) ;
#5963=LINE('',#41848,#8435) ;
#5964=LINE('',#41851,#8436) ;
#5965=LINE('',#41853,#8437) ;
#5966=LINE('',#41854,#8438) ;
#5967=LINE('',#41857,#8439) ;
#5968=LINE('',#41859,#8440) ;
#5969=LINE('',#41860,#8441) ;
#5970=LINE('',#41863,#8442) ;
#5971=LINE('',#41865,#8443) ;
#5972=LINE('',#41866,#8444) ;
#5973=LINE('',#41869,#8445) ;
#5974=LINE('',#41871,#8446) ;
#5975=LINE('',#41872,#8447) ;
#5976=LINE('',#41875,#8448) ;
#5977=LINE('',#41877,#8449) ;
#5978=LINE('',#41881,#8450) ;
#5979=LINE('',#41883,#8451) ;
#5980=LINE('',#41887,#8452) ;
#5981=LINE('',#41889,#8453) ;
#5982=LINE('',#41893,#8454) ;
#5983=LINE('',#41895,#8455) ;
#5984=LINE('',#41897,#8456) ;
#5985=LINE('',#41901,#8457) ;
#5986=LINE('',#41903,#8458) ;
#5987=LINE('',#41907,#8459) ;
#5988=LINE('',#41909,#8460) ;
#5989=LINE('',#41913,#8461) ;
#5990=LINE('',#41915,#8462) ;
#5991=LINE('',#41919,#8463) ;
#5992=LINE('',#41921,#8464) ;
#5993=LINE('',#41925,#8465) ;
#5994=LINE('',#41927,#8466) ;
#5995=LINE('',#41931,#8467) ;
#5996=LINE('',#41933,#8468) ;
#5997=LINE('',#41937,#8469) ;
#5998=LINE('',#41939,#8470) ;
#5999=LINE('',#41941,#8471) ;
#6000=LINE('',#41945,#8472) ;
#6001=LINE('',#41947,#8473) ;
#6002=LINE('',#41951,#8474) ;
#6003=LINE('',#41953,#8475) ;
#6004=LINE('',#41957,#8476) ;
#6005=LINE('',#41959,#8477) ;
#6006=LINE('',#41963,#8478) ;
#6007=LINE('',#41965,#8479) ;
#6008=LINE('',#41969,#8480) ;
#6009=LINE('',#41971,#8481) ;
#6010=LINE('',#41975,#8482) ;
#6011=LINE('',#41977,#8483) ;
#6012=LINE('',#41981,#8484) ;
#6013=LINE('',#41983,#8485) ;
#6014=LINE('',#41985,#8486) ;
#6015=LINE('',#41989,#8487) ;
#6016=LINE('',#41991,#8488) ;
#6017=LINE('',#41995,#8489) ;
#6018=LINE('',#41997,#8490) ;
#6019=LINE('',#42001,#8491) ;
#6020=LINE('',#42003,#8492) ;
#6021=LINE('',#42008,#8493) ;
#6022=LINE('',#42010,#8494) ;
#6023=LINE('',#42014,#8495) ;
#6024=LINE('',#42016,#8496) ;
#6025=LINE('',#42020,#8497) ;
#6026=LINE('',#42022,#8498) ;
#6027=LINE('',#42024,#8499) ;
#6028=LINE('',#42028,#8500) ;
#6029=LINE('',#42030,#8501) ;
#6030=LINE('',#42034,#8502) ;
#6031=LINE('',#42035,#8503) ;
#6032=LINE('',#42036,#8504) ;
#6033=LINE('',#42039,#8505) ;
#6034=LINE('',#42042,#8506) ;
#6035=LINE('',#42045,#8507) ;
#6036=LINE('',#42046,#8508) ;
#6037=LINE('',#42048,#8509) ;
#6038=LINE('',#42049,#8510) ;
#6039=LINE('',#42051,#8511) ;
#6040=LINE('',#42052,#8512) ;
#6041=LINE('',#42054,#8513) ;
#6042=LINE('',#42055,#8514) ;
#6043=LINE('',#42057,#8515) ;
#6044=LINE('',#42059,#8516) ;
#6045=LINE('',#42063,#8517) ;
#6046=LINE('',#42066,#8518) ;
#6047=LINE('',#42069,#8519) ;
#6048=LINE('',#42071,#8520) ;
#6049=LINE('',#42073,#8521) ;
#6050=LINE('',#42074,#8522) ;
#6051=LINE('',#42077,#8523) ;
#6052=LINE('',#42079,#8524) ;
#6053=LINE('',#42081,#8525) ;
#6054=LINE('',#42082,#8526) ;
#6055=LINE('',#42085,#8527) ;
#6056=LINE('',#42087,#8528) ;
#6057=LINE('',#42089,#8529) ;
#6058=LINE('',#42090,#8530) ;
#6059=LINE('',#42093,#8531) ;
#6060=LINE('',#42095,#8532) ;
#6061=LINE('',#42097,#8533) ;
#6062=LINE('',#42098,#8534) ;
#6063=LINE('',#42101,#8535) ;
#6064=LINE('',#42103,#8536) ;
#6065=LINE('',#42106,#8537) ;
#6066=LINE('',#42109,#8538) ;
#6067=LINE('',#42111,#8539) ;
#6068=LINE('',#42114,#8540) ;
#6069=LINE('',#42117,#8541) ;
#6070=LINE('',#42119,#8542) ;
#6071=LINE('',#42121,#8543) ;
#6072=LINE('',#42124,#8544) ;
#6073=LINE('',#42127,#8545) ;
#6074=LINE('',#42130,#8546) ;
#6075=LINE('',#42135,#8547) ;
#6076=LINE('',#42137,#8548) ;
#6077=LINE('',#42138,#8549) ;
#6078=LINE('',#42141,#8550) ;
#6079=LINE('',#42143,#8551) ;
#6080=LINE('',#42145,#8552) ;
#6081=LINE('',#42146,#8553) ;
#6082=LINE('',#42149,#8554) ;
#6083=LINE('',#42151,#8555) ;
#6084=LINE('',#42153,#8556) ;
#6085=LINE('',#42154,#8557) ;
#6086=LINE('',#42157,#8558) ;
#6087=LINE('',#42159,#8559) ;
#6088=LINE('',#42161,#8560) ;
#6089=LINE('',#42162,#8561) ;
#6090=LINE('',#42165,#8562) ;
#6091=LINE('',#42167,#8563) ;
#6092=LINE('',#42169,#8564) ;
#6093=LINE('',#42170,#8565) ;
#6094=LINE('',#42173,#8566) ;
#6095=LINE('',#42175,#8567) ;
#6096=LINE('',#42177,#8568) ;
#6097=LINE('',#42178,#8569) ;
#6098=LINE('',#42181,#8570) ;
#6099=LINE('',#42183,#8571) ;
#6100=LINE('',#42186,#8572) ;
#6101=LINE('',#42189,#8573) ;
#6102=LINE('',#42191,#8574) ;
#6103=LINE('',#42193,#8575) ;
#6104=LINE('',#42194,#8576) ;
#6105=LINE('',#42197,#8577) ;
#6106=LINE('',#42199,#8578) ;
#6107=LINE('',#42201,#8579) ;
#6108=LINE('',#42202,#8580) ;
#6109=LINE('',#42205,#8581) ;
#6110=LINE('',#42208,#8582) ;
#6111=LINE('',#42211,#8583) ;
#6112=LINE('',#42213,#8584) ;
#6113=LINE('',#42217,#8585) ;
#6114=LINE('',#42218,#8586) ;
#6115=LINE('',#42221,#8587) ;
#6116=LINE('',#42224,#8588) ;
#6117=LINE('',#42227,#8589) ;
#6118=LINE('',#42229,#8590) ;
#6119=LINE('',#42231,#8591) ;
#6120=LINE('',#42232,#8592) ;
#6121=LINE('',#42235,#8593) ;
#6122=LINE('',#42238,#8594) ;
#6123=LINE('',#42241,#8595) ;
#6124=LINE('',#42243,#8596) ;
#6125=LINE('',#42246,#8597) ;
#6126=LINE('',#42249,#8598) ;
#6127=LINE('',#42251,#8599) ;
#6128=LINE('',#42253,#8600) ;
#6129=LINE('',#42254,#8601) ;
#6130=LINE('',#42257,#8602) ;
#6131=LINE('',#42259,#8603) ;
#6132=LINE('',#42261,#8604) ;
#6133=LINE('',#42262,#8605) ;
#6134=LINE('',#42265,#8606) ;
#6135=LINE('',#42267,#8607) ;
#6136=LINE('',#42269,#8608) ;
#6137=LINE('',#42270,#8609) ;
#6138=LINE('',#42273,#8610) ;
#6139=LINE('',#42275,#8611) ;
#6140=LINE('',#42277,#8612) ;
#6141=LINE('',#42278,#8613) ;
#6142=LINE('',#42281,#8614) ;
#6143=LINE('',#42283,#8615) ;
#6144=LINE('',#42285,#8616) ;
#6145=LINE('',#42286,#8617) ;
#6146=LINE('',#42289,#8618) ;
#6147=LINE('',#42291,#8619) ;
#6148=LINE('',#42293,#8620) ;
#6149=LINE('',#42294,#8621) ;
#6150=LINE('',#42297,#8622) ;
#6151=LINE('',#42299,#8623) ;
#6152=LINE('',#42303,#8624) ;
#6153=LINE('',#42305,#8625) ;
#6154=LINE('',#42307,#8626) ;
#6155=LINE('',#42308,#8627) ;
#6156=LINE('',#42313,#8628) ;
#6157=LINE('',#42315,#8629) ;
#6158=LINE('',#42316,#8630) ;
#6159=LINE('',#42319,#8631) ;
#6160=LINE('',#42321,#8632) ;
#6161=LINE('',#42323,#8633) ;
#6162=LINE('',#42324,#8634) ;
#6163=LINE('',#42327,#8635) ;
#6164=LINE('',#42329,#8636) ;
#6165=LINE('',#42331,#8637) ;
#6166=LINE('',#42332,#8638) ;
#6167=LINE('',#42335,#8639) ;
#6168=LINE('',#42337,#8640) ;
#6169=LINE('',#42339,#8641) ;
#6170=LINE('',#42340,#8642) ;
#6171=LINE('',#42343,#8643) ;
#6172=LINE('',#42345,#8644) ;
#6173=LINE('',#42347,#8645) ;
#6174=LINE('',#42348,#8646) ;
#6175=LINE('',#42351,#8647) ;
#6176=LINE('',#42353,#8648) ;
#6177=LINE('',#42355,#8649) ;
#6178=LINE('',#42356,#8650) ;
#6179=LINE('',#42359,#8651) ;
#6180=LINE('',#42361,#8652) ;
#6181=LINE('',#42363,#8653) ;
#6182=LINE('',#42364,#8654) ;
#6183=LINE('',#42367,#8655) ;
#6184=LINE('',#42369,#8656) ;
#6185=LINE('',#42371,#8657) ;
#6186=LINE('',#42372,#8658) ;
#6187=LINE('',#42375,#8659) ;
#6188=LINE('',#42377,#8660) ;
#6189=LINE('',#42379,#8661) ;
#6190=LINE('',#42380,#8662) ;
#6191=LINE('',#42383,#8663) ;
#6192=LINE('',#42385,#8664) ;
#6193=LINE('',#42387,#8665) ;
#6194=LINE('',#42388,#8666) ;
#6195=LINE('',#42392,#8667) ;
#6196=LINE('',#42394,#8668) ;
#6197=LINE('',#42395,#8669) ;
#6198=LINE('',#42399,#8670) ;
#6199=LINE('',#42402,#8671) ;
#6200=LINE('',#42404,#8672) ;
#6201=LINE('',#42408,#8673) ;
#6202=LINE('',#42410,#8674) ;
#6203=LINE('',#42414,#8675) ;
#6204=LINE('',#42416,#8676) ;
#6205=LINE('',#42418,#8677) ;
#6206=LINE('',#42422,#8678) ;
#6207=LINE('',#42424,#8679) ;
#6208=LINE('',#42428,#8680) ;
#6209=LINE('',#42430,#8681) ;
#6210=LINE('',#42435,#8682) ;
#6211=LINE('',#42437,#8683) ;
#6212=LINE('',#42441,#8684) ;
#6213=LINE('',#42443,#8685) ;
#6214=LINE('',#42447,#8686) ;
#6215=LINE('',#42449,#8687) ;
#6216=LINE('',#42453,#8688) ;
#6217=LINE('',#42455,#8689) ;
#6218=LINE('',#42457,#8690) ;
#6219=LINE('',#42461,#8691) ;
#6220=LINE('',#42463,#8692) ;
#6221=LINE('',#42467,#8693) ;
#6222=LINE('',#42469,#8694) ;
#6223=LINE('',#42473,#8695) ;
#6224=LINE('',#42475,#8696) ;
#6225=LINE('',#42479,#8697) ;
#6226=LINE('',#42481,#8698) ;
#6227=LINE('',#42485,#8699) ;
#6228=LINE('',#42487,#8700) ;
#6229=LINE('',#42491,#8701) ;
#6230=LINE('',#42493,#8702) ;
#6231=LINE('',#42497,#8703) ;
#6232=LINE('',#42499,#8704) ;
#6233=LINE('',#42501,#8705) ;
#6234=LINE('',#42505,#8706) ;
#6235=LINE('',#42507,#8707) ;
#6236=LINE('',#42511,#8708) ;
#6237=LINE('',#42513,#8709) ;
#6238=LINE('',#42517,#8710) ;
#6239=LINE('',#42519,#8711) ;
#6240=LINE('',#42523,#8712) ;
#6241=LINE('',#42525,#8713) ;
#6242=LINE('',#42529,#8714) ;
#6243=LINE('',#42531,#8715) ;
#6244=LINE('',#42535,#8716) ;
#6245=LINE('',#42537,#8717) ;
#6246=LINE('',#42541,#8718) ;
#6247=LINE('',#42543,#8719) ;
#6248=LINE('',#42545,#8720) ;
#6249=LINE('',#42549,#8721) ;
#6250=LINE('',#42551,#8722) ;
#6251=LINE('',#42555,#8723) ;
#6252=LINE('',#42557,#8724) ;
#6253=LINE('',#42561,#8725) ;
#6254=LINE('',#42562,#8726) ;
#6255=LINE('',#42564,#8727) ;
#6256=LINE('',#42565,#8728) ;
#6257=LINE('',#42567,#8729) ;
#6258=LINE('',#42568,#8730) ;
#6259=LINE('',#42570,#8731) ;
#6260=LINE('',#42571,#8732) ;
#6261=LINE('',#42573,#8733) ;
#6262=LINE('',#42574,#8734) ;
#6263=LINE('',#42578,#8735) ;
#6264=LINE('',#42579,#8736) ;
#6265=LINE('',#42581,#8737) ;
#6266=LINE('',#42584,#8738) ;
#6267=LINE('',#42588,#8739) ;
#6268=LINE('',#42590,#8740) ;
#6269=LINE('',#42591,#8741) ;
#6270=LINE('',#42592,#8742) ;
#6271=LINE('',#42595,#8743) ;
#6272=LINE('',#42599,#8744) ;
#6273=LINE('',#42601,#8745) ;
#6274=LINE('',#42602,#8746) ;
#6275=LINE('',#42605,#8747) ;
#6276=LINE('',#42607,#8748) ;
#6277=LINE('',#42609,#8749) ;
#6278=LINE('',#42610,#8750) ;
#6279=LINE('',#42613,#8751) ;
#6280=LINE('',#42615,#8752) ;
#6281=LINE('',#42617,#8753) ;
#6282=LINE('',#42618,#8754) ;
#6283=LINE('',#42621,#8755) ;
#6284=LINE('',#42623,#8756) ;
#6285=LINE('',#42625,#8757) ;
#6286=LINE('',#42626,#8758) ;
#6287=LINE('',#42629,#8759) ;
#6288=LINE('',#42631,#8760) ;
#6289=LINE('',#42633,#8761) ;
#6290=LINE('',#42634,#8762) ;
#6291=LINE('',#42637,#8763) ;
#6292=LINE('',#42640,#8764) ;
#6293=LINE('',#42643,#8765) ;
#6294=LINE('',#42645,#8766) ;
#6295=LINE('',#42647,#8767) ;
#6296=LINE('',#42648,#8768) ;
#6297=LINE('',#42651,#8769) ;
#6298=LINE('',#42653,#8770) ;
#6299=LINE('',#42655,#8771) ;
#6300=LINE('',#42656,#8772) ;
#6301=LINE('',#42659,#8773) ;
#6302=LINE('',#42661,#8774) ;
#6303=LINE('',#42663,#8775) ;
#6304=LINE('',#42664,#8776) ;
#6305=LINE('',#42667,#8777) ;
#6306=LINE('',#42669,#8778) ;
#6307=LINE('',#42671,#8779) ;
#6308=LINE('',#42672,#8780) ;
#6309=LINE('',#42675,#8781) ;
#6310=LINE('',#42677,#8782) ;
#6311=LINE('',#42679,#8783) ;
#6312=LINE('',#42680,#8784) ;
#6313=LINE('',#42683,#8785) ;
#6314=LINE('',#42685,#8786) ;
#6315=LINE('',#42687,#8787) ;
#6316=LINE('',#42688,#8788) ;
#6317=LINE('',#42691,#8789) ;
#6318=LINE('',#42693,#8790) ;
#6319=LINE('',#42695,#8791) ;
#6320=LINE('',#42699,#8792) ;
#6321=LINE('',#42703,#8793) ;
#6322=LINE('',#42704,#8794) ;
#6323=LINE('',#42707,#8795) ;
#6324=LINE('',#42709,#8796) ;
#6325=LINE('',#42713,#8797) ;
#6326=LINE('',#42714,#8798) ;
#6327=LINE('',#42717,#8799) ;
#6328=LINE('',#42720,#8800) ;
#6329=LINE('',#42723,#8801) ;
#6330=LINE('',#42725,#8802) ;
#6331=LINE('',#42727,#8803) ;
#6332=LINE('',#42728,#8804) ;
#6333=LINE('',#42731,#8805) ;
#6334=LINE('',#42734,#8806) ;
#6335=LINE('',#42737,#8807) ;
#6336=LINE('',#42739,#8808) ;
#6337=LINE('',#42741,#8809) ;
#6338=LINE('',#42742,#8810) ;
#6339=LINE('',#42745,#8811) ;
#6340=LINE('',#42747,#8812) ;
#6341=LINE('',#42749,#8813) ;
#6342=LINE('',#42750,#8814) ;
#6343=LINE('',#42753,#8815) ;
#6344=LINE('',#42755,#8816) ;
#6345=LINE('',#42757,#8817) ;
#6346=LINE('',#42758,#8818) ;
#6347=LINE('',#42761,#8819) ;
#6348=LINE('',#42763,#8820) ;
#6349=LINE('',#42765,#8821) ;
#6350=LINE('',#42766,#8822) ;
#6351=LINE('',#42769,#8823) ;
#6352=LINE('',#42773,#8824) ;
#6353=LINE('',#42774,#8825) ;
#6354=LINE('',#42777,#8826) ;
#6355=LINE('',#42779,#8827) ;
#6356=LINE('',#42781,#8828) ;
#6357=LINE('',#42785,#8829) ;
#6358=LINE('',#42787,#8830) ;
#6359=LINE('',#42789,#8831) ;
#6360=LINE('',#42790,#8832) ;
#6361=LINE('',#42793,#8833) ;
#6362=LINE('',#42795,#8834) ;
#6363=LINE('',#42797,#8835) ;
#6364=LINE('',#42798,#8836) ;
#6365=LINE('',#42801,#8837) ;
#6366=LINE('',#42803,#8838) ;
#6367=LINE('',#42805,#8839) ;
#6368=LINE('',#42806,#8840) ;
#6369=LINE('',#42811,#8841) ;
#6370=LINE('',#42812,#8842) ;
#6371=LINE('',#42815,#8843) ;
#6372=LINE('',#42817,#8844) ;
#6373=LINE('',#42819,#8845) ;
#6374=LINE('',#42820,#8846) ;
#6375=LINE('',#42823,#8847) ;
#6376=LINE('',#42825,#8848) ;
#6377=LINE('',#42827,#8849) ;
#6378=LINE('',#42828,#8850) ;
#6379=LINE('',#42831,#8851) ;
#6380=LINE('',#42833,#8852) ;
#6381=LINE('',#42835,#8853) ;
#6382=LINE('',#42836,#8854) ;
#6383=LINE('',#42839,#8855) ;
#6384=LINE('',#42841,#8856) ;
#6385=LINE('',#42843,#8857) ;
#6386=LINE('',#42844,#8858) ;
#6387=LINE('',#42847,#8859) ;
#6388=LINE('',#42849,#8860) ;
#6389=LINE('',#42851,#8861) ;
#6390=LINE('',#42852,#8862) ;
#6391=LINE('',#42855,#8863) ;
#6392=LINE('',#42857,#8864) ;
#6393=LINE('',#42859,#8865) ;
#6394=LINE('',#42860,#8866) ;
#6395=LINE('',#42863,#8867) ;
#6396=LINE('',#42865,#8868) ;
#6397=LINE('',#42867,#8869) ;
#6398=LINE('',#42868,#8870) ;
#6399=LINE('',#42871,#8871) ;
#6400=LINE('',#42873,#8872) ;
#6401=LINE('',#42875,#8873) ;
#6402=LINE('',#42876,#8874) ;
#6403=LINE('',#42879,#8875) ;
#6404=LINE('',#42881,#8876) ;
#6405=LINE('',#42883,#8877) ;
#6406=LINE('',#42884,#8878) ;
#6407=LINE('',#42887,#8879) ;
#6408=LINE('',#42890,#8880) ;
#6409=LINE('',#42893,#8881) ;
#6410=LINE('',#42896,#8882) ;
#6411=LINE('',#42899,#8883) ;
#6412=LINE('',#42903,#8884) ;
#6413=LINE('',#42904,#8885) ;
#6414=LINE('',#42907,#8886) ;
#6415=LINE('',#42911,#8887) ;
#6416=LINE('',#42912,#8888) ;
#6417=LINE('',#42915,#8889) ;
#6418=LINE('',#42917,#8890) ;
#6419=LINE('',#42919,#8891) ;
#6420=LINE('',#42920,#8892) ;
#6421=LINE('',#42922,#8893) ;
#6422=LINE('',#42924,#8894) ;
#6423=LINE('',#42926,#8895) ;
#6424=LINE('',#42928,#8896) ;
#6425=LINE('',#42929,#8897) ;
#6426=LINE('',#42931,#8898) ;
#6427=LINE('',#42932,#8899) ;
#6428=LINE('',#42934,#8900) ;
#6429=LINE('',#42935,#8901) ;
#6430=LINE('',#42937,#8902) ;
#6431=LINE('',#42938,#8903) ;
#6432=LINE('',#42940,#8904) ;
#6433=LINE('',#42941,#8905) ;
#6434=LINE('',#42943,#8906) ;
#6435=LINE('',#42944,#8907) ;
#6436=LINE('',#42946,#8908) ;
#6437=LINE('',#42947,#8909) ;
#6438=LINE('',#42949,#8910) ;
#6439=LINE('',#42950,#8911) ;
#6440=LINE('',#42952,#8912) ;
#6441=LINE('',#42953,#8913) ;
#6442=LINE('',#42955,#8914) ;
#6443=LINE('',#42956,#8915) ;
#6444=LINE('',#42958,#8916) ;
#6445=LINE('',#42960,#8917) ;
#6446=LINE('',#42962,#8918) ;
#6447=LINE('',#42963,#8919) ;
#6448=LINE('',#42965,#8920) ;
#6449=LINE('',#42967,#8921) ;
#6450=LINE('',#42969,#8922) ;
#6451=LINE('',#42972,#8923) ;
#6452=LINE('',#42974,#8924) ;
#6453=LINE('',#42976,#8925) ;
#6454=LINE('',#42978,#8926) ;
#6455=LINE('',#42980,#8927) ;
#6456=LINE('',#42982,#8928) ;
#6457=LINE('',#42984,#8929) ;
#6458=LINE('',#42986,#8930) ;
#6459=LINE('',#42988,#8931) ;
#6460=LINE('',#42990,#8932) ;
#6461=LINE('',#42991,#8933) ;
#6462=LINE('',#42993,#8934) ;
#6463=LINE('',#42995,#8935) ;
#6464=LINE('',#42997,#8936) ;
#6465=LINE('',#42998,#8937) ;
#6466=LINE('',#43000,#8938) ;
#6467=LINE('',#43002,#8939) ;
#6468=LINE('',#43004,#8940) ;
#6469=LINE('',#43007,#8941) ;
#6470=LINE('',#43008,#8942) ;
#6471=LINE('',#43010,#8943) ;
#6472=LINE('',#43011,#8944) ;
#6473=LINE('',#43013,#8945) ;
#6474=LINE('',#43014,#8946) ;
#6475=LINE('',#43016,#8947) ;
#6476=LINE('',#43017,#8948) ;
#6477=LINE('',#43019,#8949) ;
#6478=LINE('',#43020,#8950) ;
#6479=LINE('',#43022,#8951) ;
#6480=LINE('',#43024,#8952) ;
#6481=LINE('',#43027,#8953) ;
#6482=LINE('',#43029,#8954) ;
#6483=LINE('',#43032,#8955) ;
#6484=LINE('',#43035,#8956) ;
#6485=LINE('',#43038,#8957) ;
#6486=LINE('',#43041,#8958) ;
#6487=LINE('',#43043,#8959) ;
#6488=LINE('',#43045,#8960) ;
#6489=LINE('',#43047,#8961) ;
#6490=LINE('',#43048,#8962) ;
#6491=LINE('',#43050,#8963) ;
#6492=LINE('',#43051,#8964) ;
#6493=LINE('',#43053,#8965) ;
#6494=LINE('',#43055,#8966) ;
#6495=LINE('',#43057,#8967) ;
#6496=LINE('',#43060,#8968) ;
#6497=LINE('',#43062,#8969) ;
#6498=LINE('',#43063,#8970) ;
#6499=LINE('',#43065,#8971) ;
#6500=LINE('',#43066,#8972) ;
#6501=LINE('',#43068,#8973) ;
#6502=LINE('',#43070,#8974) ;
#6503=LINE('',#43071,#8975) ;
#6504=LINE('',#43073,#8976) ;
#6505=LINE('',#43074,#8977) ;
#6506=LINE('',#43076,#8978) ;
#6507=LINE('',#43079,#8979) ;
#6508=LINE('',#43081,#8980) ;
#6509=LINE('',#43084,#8981) ;
#6510=LINE('',#43087,#8982) ;
#6511=LINE('',#43089,#8983) ;
#6512=LINE('',#43091,#8984) ;
#6513=LINE('',#43093,#8985) ;
#6514=LINE('',#43096,#8986) ;
#6515=LINE('',#43099,#8987) ;
#6516=LINE('',#43101,#8988) ;
#6517=LINE('',#43102,#8989) ;
#6518=LINE('',#43104,#8990) ;
#6519=LINE('',#43106,#8991) ;
#6520=LINE('',#43107,#8992) ;
#6521=LINE('',#43109,#8993) ;
#6522=LINE('',#43111,#8994) ;
#6523=LINE('',#43113,#8995) ;
#6524=LINE('',#43115,#8996) ;
#6525=LINE('',#43118,#8997) ;
#6526=LINE('',#43119,#8998) ;
#6527=LINE('',#43121,#8999) ;
#6528=LINE('',#43122,#9000) ;
#6529=LINE('',#43124,#9001) ;
#6530=LINE('',#43125,#9002) ;
#6531=LINE('',#43127,#9003) ;
#6532=LINE('',#43128,#9004) ;
#6533=LINE('',#43130,#9005) ;
#6534=LINE('',#43131,#9006) ;
#6535=LINE('',#43133,#9007) ;
#6536=LINE('',#43135,#9008) ;
#6537=LINE('',#43139,#9009) ;
#6538=LINE('',#43141,#9010) ;
#6539=LINE('',#43144,#9011) ;
#6540=LINE('',#43146,#9012) ;
#6541=LINE('',#43149,#9013) ;
#6542=LINE('',#43152,#9014) ;
#6543=LINE('',#43155,#9015) ;
#6544=LINE('',#43158,#9016) ;
#6545=LINE('',#43160,#9017) ;
#6546=LINE('',#43161,#9018) ;
#6547=LINE('',#43163,#9019) ;
#6548=LINE('',#43164,#9020) ;
#6549=LINE('',#43166,#9021) ;
#6550=LINE('',#43167,#9022) ;
#6551=LINE('',#43169,#9023) ;
#6552=LINE('',#43170,#9024) ;
#6553=LINE('',#43172,#9025) ;
#6554=LINE('',#43174,#9026) ;
#6555=LINE('',#43175,#9027) ;
#6556=LINE('',#43177,#9028) ;
#6557=LINE('',#43179,#9029) ;
#6558=LINE('',#43180,#9030) ;
#6559=LINE('',#43182,#9031) ;
#6560=LINE('',#43184,#9032) ;
#6561=LINE('',#43186,#9033) ;
#6562=LINE('',#43189,#9034) ;
#6563=LINE('',#43192,#9035) ;
#6564=LINE('',#43194,#9036) ;
#6565=LINE('',#43197,#9037) ;
#6566=LINE('',#43199,#9038) ;
#6567=LINE('',#43202,#9039) ;
#6568=LINE('',#43205,#9040) ;
#6569=LINE('',#43208,#9041) ;
#6570=LINE('',#43210,#9042) ;
#6571=LINE('',#43212,#9043) ;
#6572=LINE('',#43214,#9044) ;
#6573=LINE('',#43216,#9045) ;
#6574=LINE('',#43218,#9046) ;
#6575=LINE('',#43220,#9047) ;
#6576=LINE('',#43221,#9048) ;
#6577=LINE('',#43223,#9049) ;
#6578=LINE('',#43226,#9050) ;
#6579=LINE('',#43228,#9051) ;
#6580=LINE('',#43229,#9052) ;
#6581=LINE('',#43231,#9053) ;
#6582=LINE('',#43232,#9054) ;
#6583=LINE('',#43234,#9055) ;
#6584=LINE('',#43235,#9056) ;
#6585=LINE('',#43237,#9057) ;
#6586=LINE('',#43238,#9058) ;
#6587=LINE('',#43240,#9059) ;
#6588=LINE('',#43241,#9060) ;
#6589=LINE('',#43243,#9061) ;
#6590=LINE('',#43244,#9062) ;
#6591=LINE('',#43248,#9063) ;
#6592=LINE('',#43250,#9064) ;
#6593=LINE('',#43254,#9065) ;
#6594=LINE('',#43257,#9066) ;
#6595=LINE('',#43260,#9067) ;
#6596=LINE('',#43262,#9068) ;
#6597=LINE('',#43265,#9069) ;
#6598=LINE('',#43268,#9070) ;
#6599=LINE('',#43270,#9071) ;
#6600=LINE('',#43272,#9072) ;
#6601=LINE('',#43274,#9073) ;
#6602=LINE('',#43276,#9074) ;
#6603=LINE('',#43278,#9075) ;
#6604=LINE('',#43281,#9076) ;
#6605=LINE('',#43282,#9077) ;
#6606=LINE('',#43284,#9078) ;
#6607=LINE('',#43285,#9079) ;
#6608=LINE('',#43287,#9080) ;
#6609=LINE('',#43288,#9081) ;
#6610=LINE('',#43290,#9082) ;
#6611=LINE('',#43291,#9083) ;
#6612=LINE('',#43293,#9084) ;
#6613=LINE('',#43294,#9085) ;
#6614=LINE('',#43298,#9086) ;
#6615=LINE('',#43303,#9087) ;
#6616=LINE('',#43305,#9088) ;
#6617=LINE('',#43308,#9089) ;
#6618=LINE('',#43310,#9090) ;
#6619=LINE('',#43313,#9091) ;
#6620=LINE('',#43315,#9092) ;
#6621=LINE('',#43317,#9093) ;
#6622=LINE('',#43318,#9094) ;
#6623=LINE('',#43320,#9095) ;
#6624=LINE('',#43321,#9096) ;
#6625=LINE('',#43323,#9097) ;
#6626=LINE('',#43324,#9098) ;
#6627=LINE('',#43326,#9099) ;
#6628=LINE('',#43328,#9100) ;
#6629=LINE('',#43329,#9101) ;
#6630=LINE('',#43332,#9102) ;
#6631=LINE('',#43334,#9103) ;
#6632=LINE('',#43337,#9104) ;
#6633=LINE('',#43341,#9105) ;
#6634=LINE('',#43344,#9106) ;
#6635=LINE('',#43346,#9107) ;
#6636=LINE('',#43348,#9108) ;
#6637=LINE('',#43351,#9109) ;
#6638=LINE('',#43353,#9110) ;
#6639=LINE('',#43355,#9111) ;
#6640=LINE('',#43358,#9112) ;
#6641=LINE('',#43360,#9113) ;
#6642=LINE('',#43362,#9114) ;
#6643=LINE('',#43363,#9115) ;
#6644=LINE('',#43365,#9116) ;
#6645=LINE('',#43366,#9117) ;
#6646=LINE('',#43368,#9118) ;
#6647=LINE('',#43369,#9119) ;
#6648=LINE('',#43371,#9120) ;
#6649=LINE('',#43373,#9121) ;
#6650=LINE('',#43376,#9122) ;
#6651=LINE('',#43379,#9123) ;
#6652=LINE('',#43383,#9124) ;
#6653=LINE('',#43385,#9125) ;
#6654=LINE('',#43388,#9126) ;
#6655=LINE('',#43391,#9127) ;
#6656=LINE('',#43392,#9128) ;
#6657=LINE('',#43395,#9129) ;
#6658=LINE('',#43396,#9130) ;
#6659=LINE('',#43399,#9131) ;
#6660=LINE('',#43402,#9132) ;
#6661=LINE('',#43405,#9133) ;
#6662=LINE('',#43407,#9134) ;
#6663=LINE('',#43409,#9135) ;
#6664=LINE('',#43411,#9136) ;
#6665=LINE('',#43413,#9137) ;
#6666=LINE('',#43415,#9138) ;
#6667=LINE('',#43418,#9139) ;
#6668=LINE('',#43421,#9140) ;
#6669=LINE('',#43423,#9141) ;
#6670=LINE('',#43427,#9142) ;
#6671=LINE('',#43429,#9143) ;
#6672=LINE('',#43431,#9144) ;
#6673=LINE('',#43435,#9145) ;
#6674=LINE('',#43437,#9146) ;
#8367=VECTOR('',#32802,1.) ;
#8368=VECTOR('',#32803,1.) ;
#8369=VECTOR('',#32804,1.) ;
#8370=VECTOR('',#32805,1.) ;
#8371=VECTOR('',#32808,1.) ;
#8372=VECTOR('',#32809,1.) ;
#8373=VECTOR('',#32810,1.) ;
#8374=VECTOR('',#32811,1.) ;
#8375=VECTOR('',#32814,1.) ;
#8376=VECTOR('',#32815,1.) ;
#8377=VECTOR('',#32816,1.) ;
#8378=VECTOR('',#32817,1.) ;
#8379=VECTOR('',#32820,1.) ;
#8380=VECTOR('',#32821,1.) ;
#8381=VECTOR('',#32822,1.) ;
#8382=VECTOR('',#32823,1.) ;
#8383=VECTOR('',#32826,1.) ;
#8384=VECTOR('',#32827,1.) ;
#8385=VECTOR('',#32828,1.) ;
#8386=VECTOR('',#32829,1.) ;
#8387=VECTOR('',#32832,1.) ;
#8388=VECTOR('',#32833,1.) ;
#8389=VECTOR('',#32834,1.) ;
#8390=VECTOR('',#32835,1.) ;
#8391=VECTOR('',#32838,1.) ;
#8392=VECTOR('',#32839,1.) ;
#8393=VECTOR('',#32840,1.) ;
#8394=VECTOR('',#32841,1.) ;
#8395=VECTOR('',#32844,1.) ;
#8396=VECTOR('',#32845,1.) ;
#8397=VECTOR('',#32846,1.) ;
#8398=VECTOR('',#32847,1.) ;
#8399=VECTOR('',#32850,1.) ;
#8400=VECTOR('',#32851,1.) ;
#8401=VECTOR('',#32852,1.) ;
#8402=VECTOR('',#32853,1.) ;
#8403=VECTOR('',#32856,1.) ;
#8404=VECTOR('',#32857,1.) ;
#8405=VECTOR('',#32858,1.) ;
#8406=VECTOR('',#32859,1.) ;
#8407=VECTOR('',#32862,1.) ;
#8408=VECTOR('',#32863,1.) ;
#8409=VECTOR('',#32864,1.) ;
#8410=VECTOR('',#32865,1.) ;
#8411=VECTOR('',#32868,1.) ;
#8412=VECTOR('',#32869,1.) ;
#8413=VECTOR('',#32870,1.) ;
#8414=VECTOR('',#32871,1.) ;
#8415=VECTOR('',#32874,1.) ;
#8416=VECTOR('',#32875,1.) ;
#8417=VECTOR('',#32876,1.) ;
#8418=VECTOR('',#32879,1.) ;
#8419=VECTOR('',#32880,1.) ;
#8420=VECTOR('',#32881,1.) ;
#8421=VECTOR('',#32886,1.) ;
#8422=VECTOR('',#32893,1.) ;
#8423=VECTOR('',#32900,1.) ;
#8424=VECTOR('',#32905,1.) ;
#8425=VECTOR('',#32906,1.) ;
#8426=VECTOR('',#32907,1.) ;
#8427=VECTOR('',#32910,1.) ;
#8428=VECTOR('',#32911,1.) ;
#8429=VECTOR('',#32912,1.) ;
#8430=VECTOR('',#32915,1.) ;
#8431=VECTOR('',#32916,1.) ;
#8432=VECTOR('',#32917,1.) ;
#8433=VECTOR('',#32920,1.) ;
#8434=VECTOR('',#32921,1.) ;
#8435=VECTOR('',#32922,1.) ;
#8436=VECTOR('',#32925,1.) ;
#8437=VECTOR('',#32926,1.) ;
#8438=VECTOR('',#32927,1.) ;
#8439=VECTOR('',#32930,1.) ;
#8440=VECTOR('',#32931,1.) ;
#8441=VECTOR('',#32932,1.) ;
#8442=VECTOR('',#32935,1.) ;
#8443=VECTOR('',#32936,1.) ;
#8444=VECTOR('',#32937,1.) ;
#8445=VECTOR('',#32940,1.) ;
#8446=VECTOR('',#32941,1.) ;
#8447=VECTOR('',#32942,1.) ;
#8448=VECTOR('',#32945,1.) ;
#8449=VECTOR('',#32946,1.) ;
#8450=VECTOR('',#32949,1.) ;
#8451=VECTOR('',#32950,1.) ;
#8452=VECTOR('',#32953,1.) ;
#8453=VECTOR('',#32954,1.) ;
#8454=VECTOR('',#32957,1.) ;
#8455=VECTOR('',#32958,1.) ;
#8456=VECTOR('',#32959,1.) ;
#8457=VECTOR('',#32962,1.) ;
#8458=VECTOR('',#32963,1.) ;
#8459=VECTOR('',#32966,1.) ;
#8460=VECTOR('',#32967,1.) ;
#8461=VECTOR('',#32970,1.) ;
#8462=VECTOR('',#32971,1.) ;
#8463=VECTOR('',#32974,1.) ;
#8464=VECTOR('',#32975,1.) ;
#8465=VECTOR('',#32978,1.) ;
#8466=VECTOR('',#32979,1.) ;
#8467=VECTOR('',#32982,1.) ;
#8468=VECTOR('',#32983,1.) ;
#8469=VECTOR('',#32986,1.) ;
#8470=VECTOR('',#32987,1.) ;
#8471=VECTOR('',#32988,1.) ;
#8472=VECTOR('',#32991,1.) ;
#8473=VECTOR('',#32992,1.) ;
#8474=VECTOR('',#32995,1.) ;
#8475=VECTOR('',#32996,1.) ;
#8476=VECTOR('',#32999,1.) ;
#8477=VECTOR('',#33000,1.) ;
#8478=VECTOR('',#33003,1.) ;
#8479=VECTOR('',#33004,1.) ;
#8480=VECTOR('',#33007,1.) ;
#8481=VECTOR('',#33008,1.) ;
#8482=VECTOR('',#33011,1.) ;
#8483=VECTOR('',#33012,1.) ;
#8484=VECTOR('',#33015,1.) ;
#8485=VECTOR('',#33016,1.) ;
#8486=VECTOR('',#33017,1.) ;
#8487=VECTOR('',#33020,1.) ;
#8488=VECTOR('',#33021,1.) ;
#8489=VECTOR('',#33024,1.) ;
#8490=VECTOR('',#33025,1.) ;
#8491=VECTOR('',#33028,1.) ;
#8492=VECTOR('',#33029,1.) ;
#8493=VECTOR('',#33034,1.) ;
#8494=VECTOR('',#33035,1.) ;
#8495=VECTOR('',#33038,1.) ;
#8496=VECTOR('',#33039,1.) ;
#8497=VECTOR('',#33042,1.) ;
#8498=VECTOR('',#33043,1.) ;
#8499=VECTOR('',#33044,1.) ;
#8500=VECTOR('',#33047,1.) ;
#8501=VECTOR('',#33048,1.) ;
#8502=VECTOR('',#33051,1.) ;
#8503=VECTOR('',#33052,1.) ;
#8504=VECTOR('',#33053,1.) ;
#8505=VECTOR('',#33056,1.) ;
#8506=VECTOR('',#33059,1.) ;
#8507=VECTOR('',#33062,1.) ;
#8508=VECTOR('',#33063,1.) ;
#8509=VECTOR('',#33064,1.) ;
#8510=VECTOR('',#33065,1.) ;
#8511=VECTOR('',#33066,1.) ;
#8512=VECTOR('',#33067,1.) ;
#8513=VECTOR('',#33068,1.) ;
#8514=VECTOR('',#33069,1.) ;
#8515=VECTOR('',#33070,1.) ;
#8516=VECTOR('',#33071,1.) ;
#8517=VECTOR('',#33074,1.) ;
#8518=VECTOR('',#33077,1.) ;
#8519=VECTOR('',#33078,1.) ;
#8520=VECTOR('',#33079,1.) ;
#8521=VECTOR('',#33080,1.) ;
#8522=VECTOR('',#33081,1.) ;
#8523=VECTOR('',#33082,1.) ;
#8524=VECTOR('',#33083,1.) ;
#8525=VECTOR('',#33084,1.) ;
#8526=VECTOR('',#33085,1.) ;
#8527=VECTOR('',#33086,1.) ;
#8528=VECTOR('',#33087,1.) ;
#8529=VECTOR('',#33088,1.) ;
#8530=VECTOR('',#33089,1.) ;
#8531=VECTOR('',#33090,1.) ;
#8532=VECTOR('',#33091,1.) ;
#8533=VECTOR('',#33092,1.) ;
#8534=VECTOR('',#33093,1.) ;
#8535=VECTOR('',#33094,1.) ;
#8536=VECTOR('',#33095,1.) ;
#8537=VECTOR('',#33098,1.) ;
#8538=VECTOR('',#33099,1.) ;
#8539=VECTOR('',#33100,1.) ;
#8540=VECTOR('',#33103,1.) ;
#8541=VECTOR('',#33104,1.) ;
#8542=VECTOR('',#33105,1.) ;
#8543=VECTOR('',#33106,1.) ;
#8544=VECTOR('',#33109,1.) ;
#8545=VECTOR('',#33110,1.) ;
#8546=VECTOR('',#33113,1.) ;
#8547=VECTOR('',#33116,1.) ;
#8548=VECTOR('',#33117,1.) ;
#8549=VECTOR('',#33118,1.) ;
#8550=VECTOR('',#33119,1.) ;
#8551=VECTOR('',#33120,1.) ;
#8552=VECTOR('',#33121,1.) ;
#8553=VECTOR('',#33122,1.) ;
#8554=VECTOR('',#33123,1.) ;
#8555=VECTOR('',#33124,1.) ;
#8556=VECTOR('',#33125,1.) ;
#8557=VECTOR('',#33126,1.) ;
#8558=VECTOR('',#33127,1.) ;
#8559=VECTOR('',#33128,1.) ;
#8560=VECTOR('',#33129,1.) ;
#8561=VECTOR('',#33130,1.) ;
#8562=VECTOR('',#33131,1.) ;
#8563=VECTOR('',#33132,1.) ;
#8564=VECTOR('',#33133,1.) ;
#8565=VECTOR('',#33134,1.) ;
#8566=VECTOR('',#33135,1.) ;
#8567=VECTOR('',#33136,1.) ;
#8568=VECTOR('',#33137,1.) ;
#8569=VECTOR('',#33138,1.) ;
#8570=VECTOR('',#33139,1.) ;
#8571=VECTOR('',#33140,1.) ;
#8572=VECTOR('',#33143,1.) ;
#8573=VECTOR('',#33144,1.) ;
#8574=VECTOR('',#33145,1.) ;
#8575=VECTOR('',#33146,1.) ;
#8576=VECTOR('',#33147,1.) ;
#8577=VECTOR('',#33148,1.) ;
#8578=VECTOR('',#33149,1.) ;
#8579=VECTOR('',#33150,1.) ;
#8580=VECTOR('',#33151,1.) ;
#8581=VECTOR('',#33152,1.) ;
#8582=VECTOR('',#33155,1.) ;
#8583=VECTOR('',#33156,1.) ;
#8584=VECTOR('',#33157,1.) ;
#8585=VECTOR('',#33160,1.) ;
#8586=VECTOR('',#33161,1.) ;
#8587=VECTOR('',#33162,1.) ;
#8588=VECTOR('',#33165,1.) ;
#8589=VECTOR('',#33166,1.) ;
#8590=VECTOR('',#33167,1.) ;
#8591=VECTOR('',#33168,1.) ;
#8592=VECTOR('',#33169,1.) ;
#8593=VECTOR('',#33170,1.) ;
#8594=VECTOR('',#33173,1.) ;
#8595=VECTOR('',#33174,1.) ;
#8596=VECTOR('',#33175,1.) ;
#8597=VECTOR('',#33178,1.) ;
#8598=VECTOR('',#33179,1.) ;
#8599=VECTOR('',#33180,1.) ;
#8600=VECTOR('',#33181,1.) ;
#8601=VECTOR('',#33182,1.) ;
#8602=VECTOR('',#33183,1.) ;
#8603=VECTOR('',#33184,1.) ;
#8604=VECTOR('',#33185,1.) ;
#8605=VECTOR('',#33186,1.) ;
#8606=VECTOR('',#33187,1.) ;
#8607=VECTOR('',#33188,1.) ;
#8608=VECTOR('',#33189,1.) ;
#8609=VECTOR('',#33190,1.) ;
#8610=VECTOR('',#33191,1.) ;
#8611=VECTOR('',#33192,1.) ;
#8612=VECTOR('',#33193,1.) ;
#8613=VECTOR('',#33194,1.) ;
#8614=VECTOR('',#33195,1.) ;
#8615=VECTOR('',#33196,1.) ;
#8616=VECTOR('',#33197,1.) ;
#8617=VECTOR('',#33198,1.) ;
#8618=VECTOR('',#33199,1.) ;
#8619=VECTOR('',#33200,1.) ;
#8620=VECTOR('',#33201,1.) ;
#8621=VECTOR('',#33202,1.) ;
#8622=VECTOR('',#33203,1.) ;
#8623=VECTOR('',#33204,1.) ;
#8624=VECTOR('',#33207,1.) ;
#8625=VECTOR('',#33208,1.) ;
#8626=VECTOR('',#33209,1.) ;
#8627=VECTOR('',#33210,1.) ;
#8628=VECTOR('',#33213,1.) ;
#8629=VECTOR('',#33214,1.) ;
#8630=VECTOR('',#33215,1.) ;
#8631=VECTOR('',#33216,1.) ;
#8632=VECTOR('',#33217,1.) ;
#8633=VECTOR('',#33218,1.) ;
#8634=VECTOR('',#33219,1.) ;
#8635=VECTOR('',#33220,1.) ;
#8636=VECTOR('',#33221,1.) ;
#8637=VECTOR('',#33222,1.) ;
#8638=VECTOR('',#33223,1.) ;
#8639=VECTOR('',#33224,1.) ;
#8640=VECTOR('',#33225,1.) ;
#8641=VECTOR('',#33226,1.) ;
#8642=VECTOR('',#33227,1.) ;
#8643=VECTOR('',#33228,1.) ;
#8644=VECTOR('',#33229,1.) ;
#8645=VECTOR('',#33230,1.) ;
#8646=VECTOR('',#33231,1.) ;
#8647=VECTOR('',#33232,1.) ;
#8648=VECTOR('',#33233,1.) ;
#8649=VECTOR('',#33234,1.) ;
#8650=VECTOR('',#33235,1.) ;
#8651=VECTOR('',#33236,1.) ;
#8652=VECTOR('',#33237,1.) ;
#8653=VECTOR('',#33238,1.) ;
#8654=VECTOR('',#33239,1.) ;
#8655=VECTOR('',#33240,1.) ;
#8656=VECTOR('',#33241,1.) ;
#8657=VECTOR('',#33242,1.) ;
#8658=VECTOR('',#33243,1.) ;
#8659=VECTOR('',#33244,1.) ;
#8660=VECTOR('',#33245,1.) ;
#8661=VECTOR('',#33246,1.) ;
#8662=VECTOR('',#33247,1.) ;
#8663=VECTOR('',#33248,1.) ;
#8664=VECTOR('',#33249,1.) ;
#8665=VECTOR('',#33250,1.) ;
#8666=VECTOR('',#33251,1.) ;
#8667=VECTOR('',#33254,1.) ;
#8668=VECTOR('',#33255,1.) ;
#8669=VECTOR('',#33256,1.) ;
#8670=VECTOR('',#33261,1.) ;
#8671=VECTOR('',#33264,1.) ;
#8672=VECTOR('',#33265,1.) ;
#8673=VECTOR('',#33268,1.) ;
#8674=VECTOR('',#33269,1.) ;
#8675=VECTOR('',#33272,1.) ;
#8676=VECTOR('',#33273,1.) ;
#8677=VECTOR('',#33274,1.) ;
#8678=VECTOR('',#33277,1.) ;
#8679=VECTOR('',#33278,1.) ;
#8680=VECTOR('',#33281,1.) ;
#8681=VECTOR('',#33282,1.) ;
#8682=VECTOR('',#33287,1.) ;
#8683=VECTOR('',#33288,1.) ;
#8684=VECTOR('',#33291,1.) ;
#8685=VECTOR('',#33292,1.) ;
#8686=VECTOR('',#33295,1.) ;
#8687=VECTOR('',#33296,1.) ;
#8688=VECTOR('',#33299,1.) ;
#8689=VECTOR('',#33300,1.) ;
#8690=VECTOR('',#33301,1.) ;
#8691=VECTOR('',#33304,1.) ;
#8692=VECTOR('',#33305,1.) ;
#8693=VECTOR('',#33308,1.) ;
#8694=VECTOR('',#33309,1.) ;
#8695=VECTOR('',#33312,1.) ;
#8696=VECTOR('',#33313,1.) ;
#8697=VECTOR('',#33316,1.) ;
#8698=VECTOR('',#33317,1.) ;
#8699=VECTOR('',#33320,1.) ;
#8700=VECTOR('',#33321,1.) ;
#8701=VECTOR('',#33324,1.) ;
#8702=VECTOR('',#33325,1.) ;
#8703=VECTOR('',#33328,1.) ;
#8704=VECTOR('',#33329,1.) ;
#8705=VECTOR('',#33330,1.) ;
#8706=VECTOR('',#33333,1.) ;
#8707=VECTOR('',#33334,1.) ;
#8708=VECTOR('',#33337,1.) ;
#8709=VECTOR('',#33338,1.) ;
#8710=VECTOR('',#33341,1.) ;
#8711=VECTOR('',#33342,1.) ;
#8712=VECTOR('',#33345,1.) ;
#8713=VECTOR('',#33346,1.) ;
#8714=VECTOR('',#33349,1.) ;
#8715=VECTOR('',#33350,1.) ;
#8716=VECTOR('',#33353,1.) ;
#8717=VECTOR('',#33354,1.) ;
#8718=VECTOR('',#33357,1.) ;
#8719=VECTOR('',#33358,1.) ;
#8720=VECTOR('',#33359,1.) ;
#8721=VECTOR('',#33362,1.) ;
#8722=VECTOR('',#33363,1.) ;
#8723=VECTOR('',#33366,1.) ;
#8724=VECTOR('',#33367,1.) ;
#8725=VECTOR('',#33370,1.) ;
#8726=VECTOR('',#33371,1.) ;
#8727=VECTOR('',#33372,1.) ;
#8728=VECTOR('',#33373,1.) ;
#8729=VECTOR('',#33374,1.) ;
#8730=VECTOR('',#33375,1.) ;
#8731=VECTOR('',#33376,1.) ;
#8732=VECTOR('',#33377,1.) ;
#8733=VECTOR('',#33378,1.) ;
#8734=VECTOR('',#33379,1.) ;
#8735=VECTOR('',#33382,1.) ;
#8736=VECTOR('',#33383,1.) ;
#8737=VECTOR('',#33384,1.) ;
#8738=VECTOR('',#33387,1.) ;
#8739=VECTOR('',#33392,1.) ;
#8740=VECTOR('',#33393,1.) ;
#8741=VECTOR('',#33394,1.) ;
#8742=VECTOR('',#33395,1.) ;
#8743=VECTOR('',#33396,1.) ;
#8744=VECTOR('',#33399,1.) ;
#8745=VECTOR('',#33400,1.) ;
#8746=VECTOR('',#33401,1.) ;
#8747=VECTOR('',#33402,1.) ;
#8748=VECTOR('',#33403,1.) ;
#8749=VECTOR('',#33404,1.) ;
#8750=VECTOR('',#33405,1.) ;
#8751=VECTOR('',#33406,1.) ;
#8752=VECTOR('',#33407,1.) ;
#8753=VECTOR('',#33408,1.) ;
#8754=VECTOR('',#33409,1.) ;
#8755=VECTOR('',#33410,1.) ;
#8756=VECTOR('',#33411,1.) ;
#8757=VECTOR('',#33412,1.) ;
#8758=VECTOR('',#33413,1.) ;
#8759=VECTOR('',#33414,1.) ;
#8760=VECTOR('',#33415,1.) ;
#8761=VECTOR('',#33416,1.) ;
#8762=VECTOR('',#33417,1.) ;
#8763=VECTOR('',#33418,1.) ;
#8764=VECTOR('',#33421,1.) ;
#8765=VECTOR('',#33422,1.) ;
#8766=VECTOR('',#33423,1.) ;
#8767=VECTOR('',#33424,1.) ;
#8768=VECTOR('',#33425,1.) ;
#8769=VECTOR('',#33426,1.) ;
#8770=VECTOR('',#33427,1.) ;
#8771=VECTOR('',#33428,1.) ;
#8772=VECTOR('',#33429,1.) ;
#8773=VECTOR('',#33430,1.) ;
#8774=VECTOR('',#33431,1.) ;
#8775=VECTOR('',#33432,1.) ;
#8776=VECTOR('',#33433,1.) ;
#8777=VECTOR('',#33434,1.) ;
#8778=VECTOR('',#33435,1.) ;
#8779=VECTOR('',#33436,1.) ;
#8780=VECTOR('',#33437,1.) ;
#8781=VECTOR('',#33438,1.) ;
#8782=VECTOR('',#33439,1.) ;
#8783=VECTOR('',#33440,1.) ;
#8784=VECTOR('',#33441,1.) ;
#8785=VECTOR('',#33442,1.) ;
#8786=VECTOR('',#33443,1.) ;
#8787=VECTOR('',#33444,1.) ;
#8788=VECTOR('',#33445,1.) ;
#8789=VECTOR('',#33446,1.) ;
#8790=VECTOR('',#33447,1.) ;
#8791=VECTOR('',#33448,1.) ;
#8792=VECTOR('',#33451,1.) ;
#8793=VECTOR('',#33454,1.) ;
#8794=VECTOR('',#33455,1.) ;
#8795=VECTOR('',#33456,1.) ;
#8796=VECTOR('',#33457,1.) ;
#8797=VECTOR('',#33460,1.) ;
#8798=VECTOR('',#33461,1.) ;
#8799=VECTOR('',#33462,1.) ;
#8800=VECTOR('',#33465,1.) ;
#8801=VECTOR('',#33466,1.) ;
#8802=VECTOR('',#33467,1.) ;
#8803=VECTOR('',#33468,1.) ;
#8804=VECTOR('',#33469,1.) ;
#8805=VECTOR('',#33470,1.) ;
#8806=VECTOR('',#33473,1.) ;
#8807=VECTOR('',#33474,1.) ;
#8808=VECTOR('',#33475,1.) ;
#8809=VECTOR('',#33476,1.) ;
#8810=VECTOR('',#33477,1.) ;
#8811=VECTOR('',#33478,1.) ;
#8812=VECTOR('',#33479,1.) ;
#8813=VECTOR('',#33480,1.) ;
#8814=VECTOR('',#33481,1.) ;
#8815=VECTOR('',#33482,1.) ;
#8816=VECTOR('',#33483,1.) ;
#8817=VECTOR('',#33484,1.) ;
#8818=VECTOR('',#33485,1.) ;
#8819=VECTOR('',#33486,1.) ;
#8820=VECTOR('',#33487,1.) ;
#8821=VECTOR('',#33488,1.) ;
#8822=VECTOR('',#33489,1.) ;
#8823=VECTOR('',#33490,1.) ;
#8824=VECTOR('',#33493,1.) ;
#8825=VECTOR('',#33494,1.) ;
#8826=VECTOR('',#33495,1.) ;
#8827=VECTOR('',#33496,1.) ;
#8828=VECTOR('',#33497,1.) ;
#8829=VECTOR('',#33500,1.) ;
#8830=VECTOR('',#33501,1.) ;
#8831=VECTOR('',#33502,1.) ;
#8832=VECTOR('',#33503,1.) ;
#8833=VECTOR('',#33504,1.) ;
#8834=VECTOR('',#33505,1.) ;
#8835=VECTOR('',#33506,1.) ;
#8836=VECTOR('',#33507,1.) ;
#8837=VECTOR('',#33508,1.) ;
#8838=VECTOR('',#33509,1.) ;
#8839=VECTOR('',#33510,1.) ;
#8840=VECTOR('',#33511,1.) ;
#8841=VECTOR('',#33514,1.) ;
#8842=VECTOR('',#33515,1.) ;
#8843=VECTOR('',#33516,1.) ;
#8844=VECTOR('',#33517,1.) ;
#8845=VECTOR('',#33518,1.) ;
#8846=VECTOR('',#33519,1.) ;
#8847=VECTOR('',#33520,1.) ;
#8848=VECTOR('',#33521,1.) ;
#8849=VECTOR('',#33522,1.) ;
#8850=VECTOR('',#33523,1.) ;
#8851=VECTOR('',#33524,1.) ;
#8852=VECTOR('',#33525,1.) ;
#8853=VECTOR('',#33526,1.) ;
#8854=VECTOR('',#33527,1.) ;
#8855=VECTOR('',#33528,1.) ;
#8856=VECTOR('',#33529,1.) ;
#8857=VECTOR('',#33530,1.) ;
#8858=VECTOR('',#33531,1.) ;
#8859=VECTOR('',#33532,1.) ;
#8860=VECTOR('',#33533,1.) ;
#8861=VECTOR('',#33534,1.) ;
#8862=VECTOR('',#33535,1.) ;
#8863=VECTOR('',#33536,1.) ;
#8864=VECTOR('',#33537,1.) ;
#8865=VECTOR('',#33538,1.) ;
#8866=VECTOR('',#33539,1.) ;
#8867=VECTOR('',#33540,1.) ;
#8868=VECTOR('',#33541,1.) ;
#8869=VECTOR('',#33542,1.) ;
#8870=VECTOR('',#33543,1.) ;
#8871=VECTOR('',#33544,1.) ;
#8872=VECTOR('',#33545,1.) ;
#8873=VECTOR('',#33546,1.) ;
#8874=VECTOR('',#33547,1.) ;
#8875=VECTOR('',#33548,1.) ;
#8876=VECTOR('',#33549,1.) ;
#8877=VECTOR('',#33550,1.) ;
#8878=VECTOR('',#33551,1.) ;
#8879=VECTOR('',#33552,1.) ;
#8880=VECTOR('',#33555,1.) ;
#8881=VECTOR('',#33556,1.) ;
#8882=VECTOR('',#33559,1.) ;
#8883=VECTOR('',#33560,1.) ;
#8884=VECTOR('',#33563,1.) ;
#8885=VECTOR('',#33564,1.) ;
#8886=VECTOR('',#33565,1.) ;
#8887=VECTOR('',#33568,1.) ;
#8888=VECTOR('',#33569,1.) ;
#8889=VECTOR('',#33570,1.) ;
#8890=VECTOR('',#33571,1.) ;
#8891=VECTOR('',#33572,1.) ;
#8892=VECTOR('',#33573,1.) ;
#8893=VECTOR('',#33576,1.) ;
#8894=VECTOR('',#33579,1.) ;
#8895=VECTOR('',#33582,1.) ;
#8896=VECTOR('',#33585,1.) ;
#8897=VECTOR('',#33586,1.) ;
#8898=VECTOR('',#33589,1.) ;
#8899=VECTOR('',#33590,1.) ;
#8900=VECTOR('',#33593,1.) ;
#8901=VECTOR('',#33594,1.) ;
#8902=VECTOR('',#33597,1.) ;
#8903=VECTOR('',#33598,1.) ;
#8904=VECTOR('',#33601,1.) ;
#8905=VECTOR('',#33602,1.) ;
#8906=VECTOR('',#33605,1.) ;
#8907=VECTOR('',#33606,1.) ;
#8908=VECTOR('',#33609,1.) ;
#8909=VECTOR('',#33610,1.) ;
#8910=VECTOR('',#33613,1.) ;
#8911=VECTOR('',#33614,1.) ;
#8912=VECTOR('',#33617,1.) ;
#8913=VECTOR('',#33618,1.) ;
#8914=VECTOR('',#33621,1.) ;
#8915=VECTOR('',#33622,1.) ;
#8916=VECTOR('',#33625,1.) ;
#8917=VECTOR('',#33628,1.) ;
#8918=VECTOR('',#33631,1.) ;
#8919=VECTOR('',#33632,1.) ;
#8920=VECTOR('',#33635,1.) ;
#8921=VECTOR('',#33638,1.) ;
#8922=VECTOR('',#33641,1.) ;
#8923=VECTOR('',#33646,1.) ;
#8924=VECTOR('',#33649,1.) ;
#8925=VECTOR('',#33652,1.) ;
#8926=VECTOR('',#33655,1.) ;
#8927=VECTOR('',#33658,1.) ;
#8928=VECTOR('',#33661,1.) ;
#8929=VECTOR('',#33664,1.) ;
#8930=VECTOR('',#33667,1.) ;
#8931=VECTOR('',#33670,1.) ;
#8932=VECTOR('',#33673,1.) ;
#8933=VECTOR('',#33674,1.) ;
#8934=VECTOR('',#33677,1.) ;
#8935=VECTOR('',#33680,1.) ;
#8936=VECTOR('',#33683,1.) ;
#8937=VECTOR('',#33684,1.) ;
#8938=VECTOR('',#33687,1.) ;
#8939=VECTOR('',#33690,1.) ;
#8940=VECTOR('',#33693,1.) ;
#8941=VECTOR('',#33698,1.) ;
#8942=VECTOR('',#33699,1.) ;
#8943=VECTOR('',#33702,1.) ;
#8944=VECTOR('',#33703,1.) ;
#8945=VECTOR('',#33706,1.) ;
#8946=VECTOR('',#33707,1.) ;
#8947=VECTOR('',#33710,1.) ;
#8948=VECTOR('',#33711,1.) ;
#8949=VECTOR('',#33714,1.) ;
#8950=VECTOR('',#33715,1.) ;
#8951=VECTOR('',#33718,1.) ;
#8952=VECTOR('',#33721,1.) ;
#8953=VECTOR('',#33726,1.) ;
#8954=VECTOR('',#33729,1.) ;
#8955=VECTOR('',#33734,1.) ;
#8956=VECTOR('',#33739,1.) ;
#8957=VECTOR('',#33744,1.) ;
#8958=VECTOR('',#33749,1.) ;
#8959=VECTOR('',#33752,1.) ;
#8960=VECTOR('',#33755,1.) ;
#8961=VECTOR('',#33758,1.) ;
#8962=VECTOR('',#33759,1.) ;
#8963=VECTOR('',#33762,1.) ;
#8964=VECTOR('',#33763,1.) ;
#8965=VECTOR('',#33766,1.) ;
#8966=VECTOR('',#33769,1.) ;
#8967=VECTOR('',#33772,1.) ;
#8968=VECTOR('',#33777,1.) ;
#8969=VECTOR('',#33780,1.) ;
#8970=VECTOR('',#33781,1.) ;
#8971=VECTOR('',#33784,1.) ;
#8972=VECTOR('',#33785,1.) ;
#8973=VECTOR('',#33788,1.) ;
#8974=VECTOR('',#33791,1.) ;
#8975=VECTOR('',#33792,1.) ;
#8976=VECTOR('',#33795,1.) ;
#8977=VECTOR('',#33796,1.) ;
#8978=VECTOR('',#33799,1.) ;
#8979=VECTOR('',#33804,1.) ;
#8980=VECTOR('',#33807,1.) ;
#8981=VECTOR('',#33812,1.) ;
#8982=VECTOR('',#33817,1.) ;
#8983=VECTOR('',#33820,1.) ;
#8984=VECTOR('',#33823,1.) ;
#8985=VECTOR('',#33826,1.) ;
#8986=VECTOR('',#33831,1.) ;
#8987=VECTOR('',#33836,1.) ;
#8988=VECTOR('',#33839,1.) ;
#8989=VECTOR('',#33840,1.) ;
#8990=VECTOR('',#33843,1.) ;
#8991=VECTOR('',#33846,1.) ;
#8992=VECTOR('',#33847,1.) ;
#8993=VECTOR('',#33850,1.) ;
#8994=VECTOR('',#33853,1.) ;
#8995=VECTOR('',#33856,1.) ;
#8996=VECTOR('',#33859,1.) ;
#8997=VECTOR('',#33864,1.) ;
#8998=VECTOR('',#33865,1.) ;
#8999=VECTOR('',#33868,1.) ;
#9000=VECTOR('',#33869,1.) ;
#9001=VECTOR('',#33872,1.) ;
#9002=VECTOR('',#33873,1.) ;
#9003=VECTOR('',#33876,1.) ;
#9004=VECTOR('',#33877,1.) ;
#9005=VECTOR('',#33880,1.) ;
#9006=VECTOR('',#33881,1.) ;
#9007=VECTOR('',#33884,1.) ;
#9008=VECTOR('',#33887,1.) ;
#9009=VECTOR('',#33894,1.) ;
#9010=VECTOR('',#33897,1.) ;
#9011=VECTOR('',#33902,1.) ;
#9012=VECTOR('',#33905,1.) ;
#9013=VECTOR('',#33910,1.) ;
#9014=VECTOR('',#33915,1.) ;
#9015=VECTOR('',#33920,1.) ;
#9016=VECTOR('',#33925,1.) ;
#9017=VECTOR('',#33928,1.) ;
#9018=VECTOR('',#33929,1.) ;
#9019=VECTOR('',#33932,1.) ;
#9020=VECTOR('',#33933,1.) ;
#9021=VECTOR('',#33936,1.) ;
#9022=VECTOR('',#33937,1.) ;
#9023=VECTOR('',#33940,1.) ;
#9024=VECTOR('',#33941,1.) ;
#9025=VECTOR('',#33944,1.) ;
#9026=VECTOR('',#33947,1.) ;
#9027=VECTOR('',#33948,1.) ;
#9028=VECTOR('',#33951,1.) ;
#9029=VECTOR('',#33954,1.) ;
#9030=VECTOR('',#33955,1.) ;
#9031=VECTOR('',#33958,1.) ;
#9032=VECTOR('',#33961,1.) ;
#9033=VECTOR('',#33964,1.) ;
#9034=VECTOR('',#33969,1.) ;
#9035=VECTOR('',#33974,1.) ;
#9036=VECTOR('',#33977,1.) ;
#9037=VECTOR('',#33982,1.) ;
#9038=VECTOR('',#33985,1.) ;
#9039=VECTOR('',#33990,1.) ;
#9040=VECTOR('',#33995,1.) ;
#9041=VECTOR('',#34000,1.) ;
#9042=VECTOR('',#34003,1.) ;
#9043=VECTOR('',#34006,1.) ;
#9044=VECTOR('',#34009,1.) ;
#9045=VECTOR('',#34012,1.) ;
#9046=VECTOR('',#34015,1.) ;
#9047=VECTOR('',#34018,1.) ;
#9048=VECTOR('',#34019,1.) ;
#9049=VECTOR('',#34022,1.) ;
#9050=VECTOR('',#34027,1.) ;
#9051=VECTOR('',#34030,1.) ;
#9052=VECTOR('',#34031,1.) ;
#9053=VECTOR('',#34034,1.) ;
#9054=VECTOR('',#34035,1.) ;
#9055=VECTOR('',#34038,1.) ;
#9056=VECTOR('',#34039,1.) ;
#9057=VECTOR('',#34042,1.) ;
#9058=VECTOR('',#34043,1.) ;
#9059=VECTOR('',#34046,1.) ;
#9060=VECTOR('',#34047,1.) ;
#9061=VECTOR('',#34050,1.) ;
#9062=VECTOR('',#34051,1.) ;
#9063=VECTOR('',#34058,1.) ;
#9064=VECTOR('',#34061,1.) ;
#9065=VECTOR('',#34068,1.) ;
#9066=VECTOR('',#34073,1.) ;
#9067=VECTOR('',#34078,1.) ;
#9068=VECTOR('',#34081,1.) ;
#9069=VECTOR('',#34086,1.) ;
#9070=VECTOR('',#34091,1.) ;
#9071=VECTOR('',#34094,1.) ;
#9072=VECTOR('',#34097,1.) ;
#9073=VECTOR('',#34100,1.) ;
#9074=VECTOR('',#34103,1.) ;
#9075=VECTOR('',#34106,1.) ;
#9076=VECTOR('',#34111,1.) ;
#9077=VECTOR('',#34112,1.) ;
#9078=VECTOR('',#34115,1.) ;
#9079=VECTOR('',#34116,1.) ;
#9080=VECTOR('',#34119,1.) ;
#9081=VECTOR('',#34120,1.) ;
#9082=VECTOR('',#34123,1.) ;
#9083=VECTOR('',#34124,1.) ;
#9084=VECTOR('',#34127,1.) ;
#9085=VECTOR('',#34128,1.) ;
#9086=VECTOR('',#34135,1.) ;
#9087=VECTOR('',#34144,1.) ;
#9088=VECTOR('',#34147,1.) ;
#9089=VECTOR('',#34152,1.) ;
#9090=VECTOR('',#34155,1.) ;
#9091=VECTOR('',#34160,1.) ;
#9092=VECTOR('',#34163,1.) ;
#9093=VECTOR('',#34166,1.) ;
#9094=VECTOR('',#34167,1.) ;
#9095=VECTOR('',#34170,1.) ;
#9096=VECTOR('',#34171,1.) ;
#9097=VECTOR('',#34174,1.) ;
#9098=VECTOR('',#34175,1.) ;
#9099=VECTOR('',#34178,1.) ;
#9100=VECTOR('',#34181,1.) ;
#9101=VECTOR('',#34182,1.) ;
#9102=VECTOR('',#34187,1.) ;
#9103=VECTOR('',#34190,1.) ;
#9104=VECTOR('',#34195,1.) ;
#9105=VECTOR('',#34202,1.) ;
#9106=VECTOR('',#34207,1.) ;
#9107=VECTOR('',#34210,1.) ;
#9108=VECTOR('',#34213,1.) ;
#9109=VECTOR('',#34218,1.) ;
#9110=VECTOR('',#34221,1.) ;
#9111=VECTOR('',#34224,1.) ;
#9112=VECTOR('',#34229,1.) ;
#9113=VECTOR('',#34232,1.) ;
#9114=VECTOR('',#34235,1.) ;
#9115=VECTOR('',#34236,1.) ;
#9116=VECTOR('',#34239,1.) ;
#9117=VECTOR('',#34240,1.) ;
#9118=VECTOR('',#34243,1.) ;
#9119=VECTOR('',#34244,1.) ;
#9120=VECTOR('',#34247,1.) ;
#9121=VECTOR('',#34250,1.) ;
#9122=VECTOR('',#34255,1.) ;
#9123=VECTOR('',#34260,1.) ;
#9124=VECTOR('',#34267,1.) ;
#9125=VECTOR('',#34270,1.) ;
#9126=VECTOR('',#34275,1.) ;
#9127=VECTOR('',#34280,1.) ;
#9128=VECTOR('',#34281,1.) ;
#9129=VECTOR('',#34286,1.) ;
#9130=VECTOR('',#34287,1.) ;
#9131=VECTOR('',#34292,1.) ;
#9132=VECTOR('',#34297,1.) ;
#9133=VECTOR('',#34302,1.) ;
#9134=VECTOR('',#34305,1.) ;
#9135=VECTOR('',#34308,1.) ;
#9136=VECTOR('',#34311,1.) ;
#9137=VECTOR('',#34314,1.) ;
#9138=VECTOR('',#34317,1.) ;
#9139=VECTOR('',#34322,1.) ;
#9140=VECTOR('',#34327,1.) ;
#9141=VECTOR('',#34330,1.) ;
#9142=VECTOR('',#34337,1.) ;
#9143=VECTOR('',#34340,1.) ;
#9144=VECTOR('',#34343,1.) ;
#9145=VECTOR('',#34350,1.) ;
#9146=VECTOR('',#34353,1.) ;
#10726=CIRCLE('',#29355,51.5) ;
#10727=CIRCLE('',#29356,51.5) ;
#10728=CIRCLE('',#29358,51.5) ;
#10729=CIRCLE('',#29359,51.5) ;
#10730=CIRCLE('',#29361,50.5) ;
#10731=CIRCLE('',#29362,50.5) ;
#10732=CIRCLE('',#29372,51.5) ;
#10733=CIRCLE('',#29373,51.5) ;
#10734=CIRCLE('',#29374,51.5) ;
#10735=CIRCLE('',#29375,51.5) ;
#10736=CIRCLE('',#29376,51.5) ;
#10737=CIRCLE('',#29377,51.5) ;
#10738=CIRCLE('',#29378,51.5) ;
#10739=CIRCLE('',#29379,51.5) ;
#10740=CIRCLE('',#29380,51.5) ;
#10741=CIRCLE('',#29381,51.5) ;
#10742=CIRCLE('',#29382,51.5) ;
#10743=CIRCLE('',#29383,51.5) ;
#10744=CIRCLE('',#29384,51.5) ;
#10745=CIRCLE('',#29385,51.5) ;
#10746=CIRCLE('',#29386,51.5) ;
#10747=CIRCLE('',#29387,51.5) ;
#10748=CIRCLE('',#29388,51.5) ;
#10749=CIRCLE('',#29389,51.5) ;
#10750=CIRCLE('',#29390,51.5) ;
#10751=CIRCLE('',#29391,51.5) ;
#10752=CIRCLE('',#29392,51.5) ;
#10753=CIRCLE('',#29393,51.5) ;
#10754=CIRCLE('',#29394,51.5) ;
#10755=CIRCLE('',#29395,51.5) ;
#10756=CIRCLE('',#29396,51.5) ;
#10757=CIRCLE('',#29397,51.5) ;
#10758=CIRCLE('',#29398,50.5) ;
#10759=CIRCLE('',#29399,50.5) ;
#10760=CIRCLE('',#29400,50.5) ;
#10761=CIRCLE('',#29401,50.5) ;
#10762=CIRCLE('',#29402,50.5) ;
#10763=CIRCLE('',#29403,50.5) ;
#10764=CIRCLE('',#29404,50.5) ;
#10765=CIRCLE('',#29405,50.5) ;
#10766=CIRCLE('',#29406,50.5) ;
#10767=CIRCLE('',#29407,50.5) ;
#10768=CIRCLE('',#29408,50.5) ;
#10769=CIRCLE('',#29409,50.5) ;
#10770=CIRCLE('',#29410,50.5) ;
#10771=CIRCLE('',#29411,50.5) ;
#10772=CIRCLE('',#29412,50.5) ;
#10773=CIRCLE('',#29413,50.5) ;
#10774=CIRCLE('',#29414,50.5) ;
#10775=CIRCLE('',#29415,50.5) ;
#10776=CIRCLE('',#29416,50.5) ;
#10777=CIRCLE('',#29418,50.5) ;
#10778=CIRCLE('',#29420,51.5) ;
#10779=CIRCLE('',#29421,51.5) ;
#10780=CIRCLE('',#29422,51.5) ;
#10781=CIRCLE('',#29423,51.5) ;
#10782=CIRCLE('',#29424,51.5) ;
#10783=CIRCLE('',#29425,51.5) ;
#10784=CIRCLE('',#29426,51.5) ;
#10785=CIRCLE('',#29427,51.5) ;
#10786=CIRCLE('',#29428,51.5) ;
#10787=CIRCLE('',#29429,51.5) ;
#10788=CIRCLE('',#29430,51.5) ;
#10789=CIRCLE('',#29431,51.5) ;
#10790=CIRCLE('',#29432,51.5) ;
#10791=CIRCLE('',#29433,51.5) ;
#10792=CIRCLE('',#29434,51.5) ;
#10793=CIRCLE('',#29435,51.5) ;
#10794=CIRCLE('',#29436,51.5) ;
#10795=CIRCLE('',#29437,51.5) ;
#10796=CIRCLE('',#29438,51.5) ;
#10797=CIRCLE('',#29439,51.5) ;
#10798=CIRCLE('',#29440,51.5) ;
#10799=CIRCLE('',#29441,51.5) ;
#10800=CIRCLE('',#29442,51.5) ;
#10801=CIRCLE('',#29443,51.5) ;
#10802=CIRCLE('',#29444,51.5) ;
#10803=CIRCLE('',#29445,51.5) ;
#10804=CIRCLE('',#29446,50.5) ;
#10805=CIRCLE('',#29447,50.5) ;
#10806=CIRCLE('',#29448,50.5) ;
#10807=CIRCLE('',#29449,50.5) ;
#10808=CIRCLE('',#29450,50.5) ;
#10809=CIRCLE('',#29451,50.5) ;
#10810=CIRCLE('',#29452,50.5) ;
#10811=CIRCLE('',#29453,50.5) ;
#10812=CIRCLE('',#29454,50.5) ;
#10813=CIRCLE('',#29455,50.5) ;
#10814=CIRCLE('',#29456,50.5) ;
#10815=CIRCLE('',#29457,50.5) ;
#10816=CIRCLE('',#29458,50.5) ;
#10817=CIRCLE('',#29459,50.5) ;
#10818=CIRCLE('',#29460,50.5) ;
#10819=CIRCLE('',#29461,50.5) ;
#10820=CIRCLE('',#29462,50.5) ;
#10821=CIRCLE('',#29463,50.5) ;
#11991=VERTEX_POINT('',#41688) ;
#11992=VERTEX_POINT('',#41689) ;
#11993=VERTEX_POINT('',#41691) ;
#11994=VERTEX_POINT('',#41693) ;
#11995=VERTEX_POINT('',#41697) ;
#11996=VERTEX_POINT('',#41698) ;
#11997=VERTEX_POINT('',#41700) ;
#11998=VERTEX_POINT('',#41702) ;
#11999=VERTEX_POINT('',#41706) ;
#12000=VERTEX_POINT('',#41707) ;
#12001=VERTEX_POINT('',#41709) ;
#12002=VERTEX_POINT('',#41711) ;
#12003=VERTEX_POINT('',#41715) ;
#12004=VERTEX_POINT('',#41716) ;
#12005=VERTEX_POINT('',#41718) ;
#12006=VERTEX_POINT('',#41720) ;
#12007=VERTEX_POINT('',#41724) ;
#12008=VERTEX_POINT('',#41725) ;
#12009=VERTEX_POINT('',#41727) ;
#12010=VERTEX_POINT('',#41729) ;
#12011=VERTEX_POINT('',#41733) ;
#12012=VERTEX_POINT('',#41734) ;
#12013=VERTEX_POINT('',#41736) ;
#12014=VERTEX_POINT('',#41738) ;
#12015=VERTEX_POINT('',#41742) ;
#12016=VERTEX_POINT('',#41743) ;
#12017=VERTEX_POINT('',#41745) ;
#12018=VERTEX_POINT('',#41747) ;
#12019=VERTEX_POINT('',#41751) ;
#12020=VERTEX_POINT('',#41752) ;
#12021=VERTEX_POINT('',#41754) ;
#12022=VERTEX_POINT('',#41756) ;
#12023=VERTEX_POINT('',#41760) ;
#12024=VERTEX_POINT('',#41761) ;
#12025=VERTEX_POINT('',#41763) ;
#12026=VERTEX_POINT('',#41765) ;
#12027=VERTEX_POINT('',#41769) ;
#12028=VERTEX_POINT('',#41770) ;
#12029=VERTEX_POINT('',#41772) ;
#12030=VERTEX_POINT('',#41774) ;
#12031=VERTEX_POINT('',#41778) ;
#12032=VERTEX_POINT('',#41779) ;
#12033=VERTEX_POINT('',#41781) ;
#12034=VERTEX_POINT('',#41783) ;
#12035=VERTEX_POINT('',#41787) ;
#12036=VERTEX_POINT('',#41788) ;
#12037=VERTEX_POINT('',#41790) ;
#12038=VERTEX_POINT('',#41792) ;
#12039=VERTEX_POINT('',#41796) ;
#12040=VERTEX_POINT('',#41797) ;
#12041=VERTEX_POINT('',#41802) ;
#12042=VERTEX_POINT('',#41803) ;
#12043=VERTEX_POINT('',#41808) ;
#12044=VERTEX_POINT('',#41810) ;
#12045=VERTEX_POINT('',#41814) ;
#12046=VERTEX_POINT('',#41816) ;
#12047=VERTEX_POINT('',#41820) ;
#12048=VERTEX_POINT('',#41822) ;
#12049=VERTEX_POINT('',#41826) ;
#12050=VERTEX_POINT('',#41828) ;
#12051=VERTEX_POINT('',#41832) ;
#12052=VERTEX_POINT('',#41834) ;
#12053=VERTEX_POINT('',#41838) ;
#12054=VERTEX_POINT('',#41840) ;
#12055=VERTEX_POINT('',#41844) ;
#12056=VERTEX_POINT('',#41846) ;
#12057=VERTEX_POINT('',#41850) ;
#12058=VERTEX_POINT('',#41852) ;
#12059=VERTEX_POINT('',#41856) ;
#12060=VERTEX_POINT('',#41858) ;
#12061=VERTEX_POINT('',#41862) ;
#12062=VERTEX_POINT('',#41864) ;
#12063=VERTEX_POINT('',#41868) ;
#12064=VERTEX_POINT('',#41870) ;
#12065=VERTEX_POINT('',#41874) ;
#12066=VERTEX_POINT('',#41876) ;
#12067=VERTEX_POINT('',#41878) ;
#12068=VERTEX_POINT('',#41880) ;
#12069=VERTEX_POINT('',#41882) ;
#12070=VERTEX_POINT('',#41884) ;
#12071=VERTEX_POINT('',#41886) ;
#12072=VERTEX_POINT('',#41888) ;
#12073=VERTEX_POINT('',#41890) ;
#12074=VERTEX_POINT('',#41892) ;
#12075=VERTEX_POINT('',#41894) ;
#12076=VERTEX_POINT('',#41896) ;
#12077=VERTEX_POINT('',#41898) ;
#12078=VERTEX_POINT('',#41900) ;
#12079=VERTEX_POINT('',#41902) ;
#12080=VERTEX_POINT('',#41904) ;
#12081=VERTEX_POINT('',#41906) ;
#12082=VERTEX_POINT('',#41908) ;
#12083=VERTEX_POINT('',#41910) ;
#12084=VERTEX_POINT('',#41912) ;
#12085=VERTEX_POINT('',#41914) ;
#12086=VERTEX_POINT('',#41916) ;
#12087=VERTEX_POINT('',#41918) ;
#12088=VERTEX_POINT('',#41920) ;
#12089=VERTEX_POINT('',#41922) ;
#12090=VERTEX_POINT('',#41924) ;
#12091=VERTEX_POINT('',#41926) ;
#12092=VERTEX_POINT('',#41928) ;
#12093=VERTEX_POINT('',#41930) ;
#12094=VERTEX_POINT('',#41932) ;
#12095=VERTEX_POINT('',#41934) ;
#12096=VERTEX_POINT('',#41936) ;
#12097=VERTEX_POINT('',#41938) ;
#12098=VERTEX_POINT('',#41940) ;
#12099=VERTEX_POINT('',#41942) ;
#12100=VERTEX_POINT('',#41944) ;
#12101=VERTEX_POINT('',#41946) ;
#12102=VERTEX_POINT('',#41948) ;
#12103=VERTEX_POINT('',#41950) ;
#12104=VERTEX_POINT('',#41952) ;
#12105=VERTEX_POINT('',#41954) ;
#12106=VERTEX_POINT('',#41956) ;
#12107=VERTEX_POINT('',#41958) ;
#12108=VERTEX_POINT('',#41960) ;
#12109=VERTEX_POINT('',#41962) ;
#12110=VERTEX_POINT('',#41964) ;
#12111=VERTEX_POINT('',#41966) ;
#12112=VERTEX_POINT('',#41968) ;
#12113=VERTEX_POINT('',#41970) ;
#12114=VERTEX_POINT('',#41972) ;
#12115=VERTEX_POINT('',#41974) ;
#12116=VERTEX_POINT('',#41976) ;
#12117=VERTEX_POINT('',#41978) ;
#12118=VERTEX_POINT('',#41980) ;
#12119=VERTEX_POINT('',#41982) ;
#12120=VERTEX_POINT('',#41984) ;
#12121=VERTEX_POINT('',#41986) ;
#12122=VERTEX_POINT('',#41988) ;
#12123=VERTEX_POINT('',#41990) ;
#12124=VERTEX_POINT('',#41992) ;
#12125=VERTEX_POINT('',#41994) ;
#12126=VERTEX_POINT('',#41996) ;
#12127=VERTEX_POINT('',#41998) ;
#12128=VERTEX_POINT('',#42000) ;
#12129=VERTEX_POINT('',#42002) ;
#12130=VERTEX_POINT('',#42005) ;
#12131=VERTEX_POINT('',#42007) ;
#12132=VERTEX_POINT('',#42009) ;
#12133=VERTEX_POINT('',#42011) ;
#12134=VERTEX_POINT('',#42013) ;
#12135=VERTEX_POINT('',#42015) ;
#12136=VERTEX_POINT('',#42017) ;
#12137=VERTEX_POINT('',#42019) ;
#12138=VERTEX_POINT('',#42021) ;
#12139=VERTEX_POINT('',#42023) ;
#12140=VERTEX_POINT('',#42025) ;
#12141=VERTEX_POINT('',#42027) ;
#12142=VERTEX_POINT('',#42029) ;
#12143=VERTEX_POINT('',#42031) ;
#12144=VERTEX_POINT('',#42033) ;
#12145=VERTEX_POINT('',#42037) ;
#12146=VERTEX_POINT('',#42040) ;
#12147=VERTEX_POINT('',#42044) ;
#12148=VERTEX_POINT('',#42047) ;
#12149=VERTEX_POINT('',#42050) ;
#12150=VERTEX_POINT('',#42053) ;
#12151=VERTEX_POINT('',#42056) ;
#12152=VERTEX_POINT('',#42058) ;
#12153=VERTEX_POINT('',#42061) ;
#12154=VERTEX_POINT('',#42062) ;
#12155=VERTEX_POINT('',#42064) ;
#12156=VERTEX_POINT('',#42067) ;
#12157=VERTEX_POINT('',#42068) ;
#12158=VERTEX_POINT('',#42070) ;
#12159=VERTEX_POINT('',#42072) ;
#12160=VERTEX_POINT('',#42075) ;
#12161=VERTEX_POINT('',#42076) ;
#12162=VERTEX_POINT('',#42078) ;
#12163=VERTEX_POINT('',#42080) ;
#12164=VERTEX_POINT('',#42083) ;
#12165=VERTEX_POINT('',#42084) ;
#12166=VERTEX_POINT('',#42086) ;
#12167=VERTEX_POINT('',#42088) ;
#12168=VERTEX_POINT('',#42091) ;
#12169=VERTEX_POINT('',#42092) ;
#12170=VERTEX_POINT('',#42094) ;
#12171=VERTEX_POINT('',#42096) ;
#12172=VERTEX_POINT('',#42099) ;
#12173=VERTEX_POINT('',#42100) ;
#12174=VERTEX_POINT('',#42102) ;
#12175=VERTEX_POINT('',#42104) ;
#12176=VERTEX_POINT('',#42107) ;
#12177=VERTEX_POINT('',#42108) ;
#12178=VERTEX_POINT('',#42110) ;
#12179=VERTEX_POINT('',#42112) ;
#12180=VERTEX_POINT('',#42115) ;
#12181=VERTEX_POINT('',#42116) ;
#12182=VERTEX_POINT('',#42118) ;
#12183=VERTEX_POINT('',#42120) ;
#12184=VERTEX_POINT('',#42122) ;
#12185=VERTEX_POINT('',#42125) ;
#12186=VERTEX_POINT('',#42126) ;
#12187=VERTEX_POINT('',#42128) ;
#12188=VERTEX_POINT('',#42131) ;
#12189=VERTEX_POINT('',#42132) ;
#12190=VERTEX_POINT('',#42134) ;
#12191=VERTEX_POINT('',#42136) ;
#12192=VERTEX_POINT('',#42139) ;
#12193=VERTEX_POINT('',#42140) ;
#12194=VERTEX_POINT('',#42142) ;
#12195=VERTEX_POINT('',#42144) ;
#12196=VERTEX_POINT('',#42147) ;
#12197=VERTEX_POINT('',#42148) ;
#12198=VERTEX_POINT('',#42150) ;
#12199=VERTEX_POINT('',#42152) ;
#12200=VERTEX_POINT('',#42155) ;
#12201=VERTEX_POINT('',#42156) ;
#12202=VERTEX_POINT('',#42158) ;
#12203=VERTEX_POINT('',#42160) ;
#12204=VERTEX_POINT('',#42163) ;
#12205=VERTEX_POINT('',#42164) ;
#12206=VERTEX_POINT('',#42166) ;
#12207=VERTEX_POINT('',#42168) ;
#12208=VERTEX_POINT('',#42171) ;
#12209=VERTEX_POINT('',#42172) ;
#12210=VERTEX_POINT('',#42174) ;
#12211=VERTEX_POINT('',#42176) ;
#12212=VERTEX_POINT('',#42179) ;
#12213=VERTEX_POINT('',#42180) ;
#12214=VERTEX_POINT('',#42182) ;
#12215=VERTEX_POINT('',#42184) ;
#12216=VERTEX_POINT('',#42187) ;
#12217=VERTEX_POINT('',#42188) ;
#12218=VERTEX_POINT('',#42190) ;
#12219=VERTEX_POINT('',#42192) ;
#12220=VERTEX_POINT('',#42195) ;
#12221=VERTEX_POINT('',#42196) ;
#12222=VERTEX_POINT('',#42198) ;
#12223=VERTEX_POINT('',#42200) ;
#12224=VERTEX_POINT('',#42203) ;
#12225=VERTEX_POINT('',#42204) ;
#12226=VERTEX_POINT('',#42206) ;
#12227=VERTEX_POINT('',#42209) ;
#12228=VERTEX_POINT('',#42210) ;
#12229=VERTEX_POINT('',#42212) ;
#12230=VERTEX_POINT('',#42214) ;
#12231=VERTEX_POINT('',#42216) ;
#12232=VERTEX_POINT('',#42219) ;
#12233=VERTEX_POINT('',#42220) ;
#12234=VERTEX_POINT('',#42222) ;
#12235=VERTEX_POINT('',#42225) ;
#12236=VERTEX_POINT('',#42226) ;
#12237=VERTEX_POINT('',#42228) ;
#12238=VERTEX_POINT('',#42230) ;
#12239=VERTEX_POINT('',#42233) ;
#12240=VERTEX_POINT('',#42234) ;
#12241=VERTEX_POINT('',#42236) ;
#12242=VERTEX_POINT('',#42239) ;
#12243=VERTEX_POINT('',#42240) ;
#12244=VERTEX_POINT('',#42242) ;
#12245=VERTEX_POINT('',#42244) ;
#12246=VERTEX_POINT('',#42247) ;
#12247=VERTEX_POINT('',#42248) ;
#12248=VERTEX_POINT('',#42250) ;
#12249=VERTEX_POINT('',#42252) ;
#12250=VERTEX_POINT('',#42255) ;
#12251=VERTEX_POINT('',#42256) ;
#12252=VERTEX_POINT('',#42258) ;
#12253=VERTEX_POINT('',#42260) ;
#12254=VERTEX_POINT('',#42263) ;
#12255=VERTEX_POINT('',#42264) ;
#12256=VERTEX_POINT('',#42266) ;
#12257=VERTEX_POINT('',#42268) ;
#12258=VERTEX_POINT('',#42271) ;
#12259=VERTEX_POINT('',#42272) ;
#12260=VERTEX_POINT('',#42274) ;
#12261=VERTEX_POINT('',#42276) ;
#12262=VERTEX_POINT('',#42279) ;
#12263=VERTEX_POINT('',#42280) ;
#12264=VERTEX_POINT('',#42282) ;
#12265=VERTEX_POINT('',#42284) ;
#12266=VERTEX_POINT('',#42287) ;
#12267=VERTEX_POINT('',#42288) ;
#12268=VERTEX_POINT('',#42290) ;
#12269=VERTEX_POINT('',#42292) ;
#12270=VERTEX_POINT('',#42295) ;
#12271=VERTEX_POINT('',#42296) ;
#12272=VERTEX_POINT('',#42298) ;
#12273=VERTEX_POINT('',#42301) ;
#12274=VERTEX_POINT('',#42302) ;
#12275=VERTEX_POINT('',#42304) ;
#12276=VERTEX_POINT('',#42306) ;
#12277=VERTEX_POINT('',#42309) ;
#12278=VERTEX_POINT('',#42310) ;
#12279=VERTEX_POINT('',#42312) ;
#12280=VERTEX_POINT('',#42314) ;
#12281=VERTEX_POINT('',#42317) ;
#12282=VERTEX_POINT('',#42318) ;
#12283=VERTEX_POINT('',#42320) ;
#12284=VERTEX_POINT('',#42322) ;
#12285=VERTEX_POINT('',#42325) ;
#12286=VERTEX_POINT('',#42326) ;
#12287=VERTEX_POINT('',#42328) ;
#12288=VERTEX_POINT('',#42330) ;
#12289=VERTEX_POINT('',#42333) ;
#12290=VERTEX_POINT('',#42334) ;
#12291=VERTEX_POINT('',#42336) ;
#12292=VERTEX_POINT('',#42338) ;
#12293=VERTEX_POINT('',#42341) ;
#12294=VERTEX_POINT('',#42342) ;
#12295=VERTEX_POINT('',#42344) ;
#12296=VERTEX_POINT('',#42346) ;
#12297=VERTEX_POINT('',#42349) ;
#12298=VERTEX_POINT('',#42350) ;
#12299=VERTEX_POINT('',#42352) ;
#12300=VERTEX_POINT('',#42354) ;
#12301=VERTEX_POINT('',#42357) ;
#12302=VERTEX_POINT('',#42358) ;
#12303=VERTEX_POINT('',#42360) ;
#12304=VERTEX_POINT('',#42362) ;
#12305=VERTEX_POINT('',#42365) ;
#12306=VERTEX_POINT('',#42366) ;
#12307=VERTEX_POINT('',#42368) ;
#12308=VERTEX_POINT('',#42370) ;
#12309=VERTEX_POINT('',#42373) ;
#12310=VERTEX_POINT('',#42374) ;
#12311=VERTEX_POINT('',#42376) ;
#12312=VERTEX_POINT('',#42378) ;
#12313=VERTEX_POINT('',#42381) ;
#12314=VERTEX_POINT('',#42382) ;
#12315=VERTEX_POINT('',#42384) ;
#12316=VERTEX_POINT('',#42386) ;
#12317=VERTEX_POINT('',#42389) ;
#12318=VERTEX_POINT('',#42391) ;
#12319=VERTEX_POINT('',#42393) ;
#12320=VERTEX_POINT('',#42397) ;
#12321=VERTEX_POINT('',#42401) ;
#12322=VERTEX_POINT('',#42403) ;
#12323=VERTEX_POINT('',#42405) ;
#12324=VERTEX_POINT('',#42407) ;
#12325=VERTEX_POINT('',#42409) ;
#12326=VERTEX_POINT('',#42411) ;
#12327=VERTEX_POINT('',#42413) ;
#12328=VERTEX_POINT('',#42415) ;
#12329=VERTEX_POINT('',#42417) ;
#12330=VERTEX_POINT('',#42419) ;
#12331=VERTEX_POINT('',#42421) ;
#12332=VERTEX_POINT('',#42423) ;
#12333=VERTEX_POINT('',#42425) ;
#12334=VERTEX_POINT('',#42427) ;
#12335=VERTEX_POINT('',#42429) ;
#12336=VERTEX_POINT('',#42432) ;
#12337=VERTEX_POINT('',#42434) ;
#12338=VERTEX_POINT('',#42436) ;
#12339=VERTEX_POINT('',#42438) ;
#12340=VERTEX_POINT('',#42440) ;
#12341=VERTEX_POINT('',#42442) ;
#12342=VERTEX_POINT('',#42444) ;
#12343=VERTEX_POINT('',#42446) ;
#12344=VERTEX_POINT('',#42448) ;
#12345=VERTEX_POINT('',#42450) ;
#12346=VERTEX_POINT('',#42452) ;
#12347=VERTEX_POINT('',#42454) ;
#12348=VERTEX_POINT('',#42456) ;
#12349=VERTEX_POINT('',#42458) ;
#12350=VERTEX_POINT('',#42460) ;
#12351=VERTEX_POINT('',#42462) ;
#12352=VERTEX_POINT('',#42464) ;
#12353=VERTEX_POINT('',#42466) ;
#12354=VERTEX_POINT('',#42468) ;
#12355=VERTEX_POINT('',#42470) ;
#12356=VERTEX_POINT('',#42472) ;
#12357=VERTEX_POINT('',#42474) ;
#12358=VERTEX_POINT('',#42476) ;
#12359=VERTEX_POINT('',#42478) ;
#12360=VERTEX_POINT('',#42480) ;
#12361=VERTEX_POINT('',#42482) ;
#12362=VERTEX_POINT('',#42484) ;
#12363=VERTEX_POINT('',#42486) ;
#12364=VERTEX_POINT('',#42488) ;
#12365=VERTEX_POINT('',#42490) ;
#12366=VERTEX_POINT('',#42492) ;
#12367=VERTEX_POINT('',#42494) ;
#12368=VERTEX_POINT('',#42496) ;
#12369=VERTEX_POINT('',#42498) ;
#12370=VERTEX_POINT('',#42500) ;
#12371=VERTEX_POINT('',#42502) ;
#12372=VERTEX_POINT('',#42504) ;
#12373=VERTEX_POINT('',#42506) ;
#12374=VERTEX_POINT('',#42508) ;
#12375=VERTEX_POINT('',#42510) ;
#12376=VERTEX_POINT('',#42512) ;
#12377=VERTEX_POINT('',#42514) ;
#12378=VERTEX_POINT('',#42516) ;
#12379=VERTEX_POINT('',#42518) ;
#12380=VERTEX_POINT('',#42520) ;
#12381=VERTEX_POINT('',#42522) ;
#12382=VERTEX_POINT('',#42524) ;
#12383=VERTEX_POINT('',#42526) ;
#12384=VERTEX_POINT('',#42528) ;
#12385=VERTEX_POINT('',#42530) ;
#12386=VERTEX_POINT('',#42532) ;
#12387=VERTEX_POINT('',#42534) ;
#12388=VERTEX_POINT('',#42536) ;
#12389=VERTEX_POINT('',#42538) ;
#12390=VERTEX_POINT('',#42540) ;
#12391=VERTEX_POINT('',#42542) ;
#12392=VERTEX_POINT('',#42544) ;
#12393=VERTEX_POINT('',#42546) ;
#12394=VERTEX_POINT('',#42548) ;
#12395=VERTEX_POINT('',#42550) ;
#12396=VERTEX_POINT('',#42552) ;
#12397=VERTEX_POINT('',#42554) ;
#12398=VERTEX_POINT('',#42556) ;
#12399=VERTEX_POINT('',#42558) ;
#12400=VERTEX_POINT('',#42560) ;
#12401=VERTEX_POINT('',#42563) ;
#12402=VERTEX_POINT('',#42566) ;
#12403=VERTEX_POINT('',#42569) ;
#12404=VERTEX_POINT('',#42572) ;
#12405=VERTEX_POINT('',#42575) ;
#12406=VERTEX_POINT('',#42577) ;
#12407=VERTEX_POINT('',#42580) ;
#12408=VERTEX_POINT('',#42583) ;
#12409=VERTEX_POINT('',#42587) ;
#12410=VERTEX_POINT('',#42589) ;
#12411=VERTEX_POINT('',#42593) ;
#12412=VERTEX_POINT('',#42594) ;
#12413=VERTEX_POINT('',#42596) ;
#12414=VERTEX_POINT('',#42598) ;
#12415=VERTEX_POINT('',#42600) ;
#12416=VERTEX_POINT('',#42603) ;
#12417=VERTEX_POINT('',#42604) ;
#12418=VERTEX_POINT('',#42606) ;
#12419=VERTEX_POINT('',#42608) ;
#12420=VERTEX_POINT('',#42611) ;
#12421=VERTEX_POINT('',#42612) ;
#12422=VERTEX_POINT('',#42614) ;
#12423=VERTEX_POINT('',#42616) ;
#12424=VERTEX_POINT('',#42619) ;
#12425=VERTEX_POINT('',#42620) ;
#12426=VERTEX_POINT('',#42622) ;
#12427=VERTEX_POINT('',#42624) ;
#12428=VERTEX_POINT('',#42627) ;
#12429=VERTEX_POINT('',#42628) ;
#12430=VERTEX_POINT('',#42630) ;
#12431=VERTEX_POINT('',#42632) ;
#12432=VERTEX_POINT('',#42635) ;
#12433=VERTEX_POINT('',#42636) ;
#12434=VERTEX_POINT('',#42638) ;
#12435=VERTEX_POINT('',#42641) ;
#12436=VERTEX_POINT('',#42642) ;
#12437=VERTEX_POINT('',#42644) ;
#12438=VERTEX_POINT('',#42646) ;
#12439=VERTEX_POINT('',#42649) ;
#12440=VERTEX_POINT('',#42650) ;
#12441=VERTEX_POINT('',#42652) ;
#12442=VERTEX_POINT('',#42654) ;
#12443=VERTEX_POINT('',#42657) ;
#12444=VERTEX_POINT('',#42658) ;
#12445=VERTEX_POINT('',#42660) ;
#12446=VERTEX_POINT('',#42662) ;
#12447=VERTEX_POINT('',#42665) ;
#12448=VERTEX_POINT('',#42666) ;
#12449=VERTEX_POINT('',#42668) ;
#12450=VERTEX_POINT('',#42670) ;
#12451=VERTEX_POINT('',#42673) ;
#12452=VERTEX_POINT('',#42674) ;
#12453=VERTEX_POINT('',#42676) ;
#12454=VERTEX_POINT('',#42678) ;
#12455=VERTEX_POINT('',#42681) ;
#12456=VERTEX_POINT('',#42682) ;
#12457=VERTEX_POINT('',#42684) ;
#12458=VERTEX_POINT('',#42686) ;
#12459=VERTEX_POINT('',#42689) ;
#12460=VERTEX_POINT('',#42690) ;
#12461=VERTEX_POINT('',#42692) ;
#12462=VERTEX_POINT('',#42694) ;
#12463=VERTEX_POINT('',#42697) ;
#12464=VERTEX_POINT('',#42698) ;
#12465=VERTEX_POINT('',#42700) ;
#12466=VERTEX_POINT('',#42702) ;
#12467=VERTEX_POINT('',#42705) ;
#12468=VERTEX_POINT('',#42706) ;
#12469=VERTEX_POINT('',#42708) ;
#12470=VERTEX_POINT('',#42710) ;
#12471=VERTEX_POINT('',#42712) ;
#12472=VERTEX_POINT('',#42715) ;
#12473=VERTEX_POINT('',#42716) ;
#12474=VERTEX_POINT('',#42718) ;
#12475=VERTEX_POINT('',#42721) ;
#12476=VERTEX_POINT('',#42722) ;
#12477=VERTEX_POINT('',#42724) ;
#12478=VERTEX_POINT('',#42726) ;
#12479=VERTEX_POINT('',#42729) ;
#12480=VERTEX_POINT('',#42730) ;
#12481=VERTEX_POINT('',#42732) ;
#12482=VERTEX_POINT('',#42735) ;
#12483=VERTEX_POINT('',#42736) ;
#12484=VERTEX_POINT('',#42738) ;
#12485=VERTEX_POINT('',#42740) ;
#12486=VERTEX_POINT('',#42743) ;
#12487=VERTEX_POINT('',#42744) ;
#12488=VERTEX_POINT('',#42746) ;
#12489=VERTEX_POINT('',#42748) ;
#12490=VERTEX_POINT('',#42751) ;
#12491=VERTEX_POINT('',#42752) ;
#12492=VERTEX_POINT('',#42754) ;
#12493=VERTEX_POINT('',#42756) ;
#12494=VERTEX_POINT('',#42759) ;
#12495=VERTEX_POINT('',#42760) ;
#12496=VERTEX_POINT('',#42762) ;
#12497=VERTEX_POINT('',#42764) ;
#12498=VERTEX_POINT('',#42767) ;
#12499=VERTEX_POINT('',#42768) ;
#12500=VERTEX_POINT('',#42770) ;
#12501=VERTEX_POINT('',#42772) ;
#12502=VERTEX_POINT('',#42775) ;
#12503=VERTEX_POINT('',#42776) ;
#12504=VERTEX_POINT('',#42778) ;
#12505=VERTEX_POINT('',#42780) ;
#12506=VERTEX_POINT('',#42783) ;
#12507=VERTEX_POINT('',#42784) ;
#12508=VERTEX_POINT('',#42786) ;
#12509=VERTEX_POINT('',#42788) ;
#12510=VERTEX_POINT('',#42791) ;
#12511=VERTEX_POINT('',#42792) ;
#12512=VERTEX_POINT('',#42794) ;
#12513=VERTEX_POINT('',#42796) ;
#12514=VERTEX_POINT('',#42799) ;
#12515=VERTEX_POINT('',#42800) ;
#12516=VERTEX_POINT('',#42802) ;
#12517=VERTEX_POINT('',#42804) ;
#12518=VERTEX_POINT('',#42807) ;
#12519=VERTEX_POINT('',#42808) ;
#12520=VERTEX_POINT('',#42810) ;
#12521=VERTEX_POINT('',#42813) ;
#12522=VERTEX_POINT('',#42814) ;
#12523=VERTEX_POINT('',#42816) ;
#12524=VERTEX_POINT('',#42818) ;
#12525=VERTEX_POINT('',#42821) ;
#12526=VERTEX_POINT('',#42822) ;
#12527=VERTEX_POINT('',#42824) ;
#12528=VERTEX_POINT('',#42826) ;
#12529=VERTEX_POINT('',#42829) ;
#12530=VERTEX_POINT('',#42830) ;
#12531=VERTEX_POINT('',#42832) ;
#12532=VERTEX_POINT('',#42834) ;
#12533=VERTEX_POINT('',#42837) ;
#12534=VERTEX_POINT('',#42838) ;
#12535=VERTEX_POINT('',#42840) ;
#12536=VERTEX_POINT('',#42842) ;
#12537=VERTEX_POINT('',#42845) ;
#12538=VERTEX_POINT('',#42846) ;
#12539=VERTEX_POINT('',#42848) ;
#12540=VERTEX_POINT('',#42850) ;
#12541=VERTEX_POINT('',#42853) ;
#12542=VERTEX_POINT('',#42854) ;
#12543=VERTEX_POINT('',#42856) ;
#12544=VERTEX_POINT('',#42858) ;
#12545=VERTEX_POINT('',#42861) ;
#12546=VERTEX_POINT('',#42862) ;
#12547=VERTEX_POINT('',#42864) ;
#12548=VERTEX_POINT('',#42866) ;
#12549=VERTEX_POINT('',#42869) ;
#12550=VERTEX_POINT('',#42870) ;
#12551=VERTEX_POINT('',#42872) ;
#12552=VERTEX_POINT('',#42874) ;
#12553=VERTEX_POINT('',#42877) ;
#12554=VERTEX_POINT('',#42878) ;
#12555=VERTEX_POINT('',#42880) ;
#12556=VERTEX_POINT('',#42882) ;
#12557=VERTEX_POINT('',#42885) ;
#12558=VERTEX_POINT('',#42886) ;
#12559=VERTEX_POINT('',#42888) ;
#12560=VERTEX_POINT('',#42891) ;
#12561=VERTEX_POINT('',#42892) ;
#12562=VERTEX_POINT('',#42894) ;
#12563=VERTEX_POINT('',#42897) ;
#12564=VERTEX_POINT('',#42898) ;
#12565=VERTEX_POINT('',#42900) ;
#12566=VERTEX_POINT('',#42902) ;
#12567=VERTEX_POINT('',#42905) ;
#12568=VERTEX_POINT('',#42906) ;
#12569=VERTEX_POINT('',#42908) ;
#12570=VERTEX_POINT('',#42910) ;
#12571=VERTEX_POINT('',#42913) ;
#12572=VERTEX_POINT('',#42914) ;
#12573=VERTEX_POINT('',#42916) ;
#12574=VERTEX_POINT('',#42918) ;
#14766=EDGE_CURVE('',#11991,#11992,#5895,.T.) ;
#14767=EDGE_CURVE('',#11993,#11991,#5896,.T.) ;
#14768=EDGE_CURVE('',#11994,#11993,#5897,.T.) ;
#14769=EDGE_CURVE('',#11992,#11994,#5898,.T.) ;
#14770=EDGE_CURVE('',#11995,#11996,#5899,.T.) ;
#14771=EDGE_CURVE('',#11997,#11995,#5900,.T.) ;
#14772=EDGE_CURVE('',#11998,#11997,#5901,.T.) ;
#14773=EDGE_CURVE('',#11996,#11998,#5902,.T.) ;
#14774=EDGE_CURVE('',#11999,#12000,#5903,.T.) ;
#14775=EDGE_CURVE('',#12001,#11999,#5904,.T.) ;
#14776=EDGE_CURVE('',#12002,#12001,#5905,.T.) ;
#14777=EDGE_CURVE('',#12000,#12002,#5906,.T.) ;
#14778=EDGE_CURVE('',#12003,#12004,#5907,.T.) ;
#14779=EDGE_CURVE('',#12005,#12003,#5908,.T.) ;
#14780=EDGE_CURVE('',#12006,#12005,#5909,.T.) ;
#14781=EDGE_CURVE('',#12004,#12006,#5910,.T.) ;
#14782=EDGE_CURVE('',#12007,#12008,#5911,.T.) ;
#14783=EDGE_CURVE('',#12009,#12007,#5912,.T.) ;
#14784=EDGE_CURVE('',#12010,#12009,#5913,.T.) ;
#14785=EDGE_CURVE('',#12008,#12010,#5914,.T.) ;
#14786=EDGE_CURVE('',#12011,#12012,#5915,.T.) ;
#14787=EDGE_CURVE('',#12013,#12011,#5916,.T.) ;
#14788=EDGE_CURVE('',#12014,#12013,#5917,.T.) ;
#14789=EDGE_CURVE('',#12012,#12014,#5918,.T.) ;
#14790=EDGE_CURVE('',#12015,#12016,#5919,.T.) ;
#14791=EDGE_CURVE('',#12017,#12015,#5920,.T.) ;
#14792=EDGE_CURVE('',#12018,#12017,#5921,.T.) ;
#14793=EDGE_CURVE('',#12016,#12018,#5922,.T.) ;
#14794=EDGE_CURVE('',#12019,#12020,#5923,.T.) ;
#14795=EDGE_CURVE('',#12021,#12019,#5924,.T.) ;
#14796=EDGE_CURVE('',#12021,#12022,#5925,.T.) ;
#14797=EDGE_CURVE('',#12020,#12022,#5926,.T.) ;
#14798=EDGE_CURVE('',#12023,#12024,#5927,.T.) ;
#14799=EDGE_CURVE('',#12025,#12023,#5928,.T.) ;
#14800=EDGE_CURVE('',#12026,#12025,#5929,.T.) ;
#14801=EDGE_CURVE('',#12024,#12026,#5930,.T.) ;
#14802=EDGE_CURVE('',#12027,#12028,#5931,.T.) ;
#14803=EDGE_CURVE('',#12029,#12027,#5932,.T.) ;
#14804=EDGE_CURVE('',#12030,#12029,#5933,.T.) ;
#14805=EDGE_CURVE('',#12028,#12030,#5934,.T.) ;
#14806=EDGE_CURVE('',#12031,#12032,#5935,.T.) ;
#14807=EDGE_CURVE('',#12033,#12031,#5936,.T.) ;
#14808=EDGE_CURVE('',#12034,#12033,#5937,.T.) ;
#14809=EDGE_CURVE('',#12032,#12034,#5938,.T.) ;
#14810=EDGE_CURVE('',#12035,#12036,#5939,.T.) ;
#14811=EDGE_CURVE('',#12037,#12035,#5940,.T.) ;
#14812=EDGE_CURVE('',#12038,#12037,#5941,.T.) ;
#14813=EDGE_CURVE('',#12036,#12038,#5942,.T.) ;
#14814=EDGE_CURVE('',#12039,#12040,#5943,.T.) ;
#14815=EDGE_CURVE('',#12022,#12039,#5944,.T.) ;
#14816=EDGE_CURVE('',#12040,#12021,#5945,.T.) ;
#14817=EDGE_CURVE('',#12041,#12042,#5946,.T.) ;
#14818=EDGE_CURVE('',#12018,#12041,#5947,.T.) ;
#14819=EDGE_CURVE('',#12042,#12017,#5948,.T.) ;
#14820=EDGE_CURVE('',#12043,#12016,#10726,.T.) ;
#14821=EDGE_CURVE('',#12043,#12044,#5949,.T.) ;
#14822=EDGE_CURVE('',#12015,#12044,#10727,.T.) ;
#14823=EDGE_CURVE('',#12045,#12042,#10728,.T.) ;
#14824=EDGE_CURVE('',#12045,#12046,#5950,.T.) ;
#14825=EDGE_CURVE('',#12041,#12046,#10729,.T.) ;
#14826=EDGE_CURVE('',#12047,#12036,#10730,.T.) ;
#14827=EDGE_CURVE('',#12047,#12048,#5951,.T.) ;
#14828=EDGE_CURVE('',#12035,#12048,#10731,.T.) ;
#14829=EDGE_CURVE('',#12049,#12013,#5952,.T.) ;
#14830=EDGE_CURVE('',#12049,#12050,#5953,.T.) ;
#14831=EDGE_CURVE('',#12014,#12050,#5954,.T.) ;
#14832=EDGE_CURVE('',#12051,#12032,#5955,.T.) ;
#14833=EDGE_CURVE('',#12052,#12051,#5956,.T.) ;
#14834=EDGE_CURVE('',#12031,#12052,#5957,.T.) ;
#14835=EDGE_CURVE('',#12053,#12009,#5958,.T.) ;
#14836=EDGE_CURVE('',#12053,#12054,#5959,.T.) ;
#14837=EDGE_CURVE('',#12010,#12054,#5960,.T.) ;
#14838=EDGE_CURVE('',#12055,#12028,#5961,.T.) ;
#14839=EDGE_CURVE('',#12056,#12055,#5962,.T.) ;
#14840=EDGE_CURVE('',#12027,#12056,#5963,.T.) ;
#14841=EDGE_CURVE('',#12057,#12005,#5964,.T.) ;
#14842=EDGE_CURVE('',#12057,#12058,#5965,.T.) ;
#14843=EDGE_CURVE('',#12006,#12058,#5966,.T.) ;
#14844=EDGE_CURVE('',#12059,#12024,#5967,.T.) ;
#14845=EDGE_CURVE('',#12060,#12059,#5968,.T.) ;
#14846=EDGE_CURVE('',#12023,#12060,#5969,.T.) ;
#14847=EDGE_CURVE('',#12061,#12001,#5970,.T.) ;
#14848=EDGE_CURVE('',#12061,#12062,#5971,.T.) ;
#14849=EDGE_CURVE('',#12002,#12062,#5972,.T.) ;
#14850=EDGE_CURVE('',#12063,#11997,#5973,.T.) ;
#14851=EDGE_CURVE('',#12063,#12064,#5974,.T.) ;
#14852=EDGE_CURVE('',#11998,#12064,#5975,.T.) ;
#14853=EDGE_CURVE('',#12046,#12065,#5976,.T.) ;
#14854=EDGE_CURVE('',#12065,#12066,#5977,.T.) ;
#14855=EDGE_CURVE('',#12066,#12067,#10732,.T.) ;
#14856=EDGE_CURVE('',#12067,#12068,#5978,.T.) ;
#14857=EDGE_CURVE('',#12068,#12069,#5979,.T.) ;
#14858=EDGE_CURVE('',#12069,#12070,#10733,.T.) ;
#14859=EDGE_CURVE('',#12070,#12071,#5980,.T.) ;
#14860=EDGE_CURVE('',#12071,#12072,#5981,.T.) ;
#14861=EDGE_CURVE('',#12072,#12073,#10734,.T.) ;
#14862=EDGE_CURVE('',#12073,#12074,#5982,.T.) ;
#14863=EDGE_CURVE('',#12074,#12075,#5983,.T.) ;
#14864=EDGE_CURVE('',#12075,#12076,#5984,.T.) ;
#14865=EDGE_CURVE('',#12076,#12077,#10735,.T.) ;
#14866=EDGE_CURVE('',#12077,#12078,#5985,.T.) ;
#14867=EDGE_CURVE('',#12078,#12079,#5986,.T.) ;
#14868=EDGE_CURVE('',#12079,#12080,#10736,.T.) ;
#14869=EDGE_CURVE('',#12080,#12081,#5987,.T.) ;
#14870=EDGE_CURVE('',#12081,#12082,#5988,.T.) ;
#14871=EDGE_CURVE('',#12082,#12083,#10737,.T.) ;
#14872=EDGE_CURVE('',#12083,#12084,#5989,.T.) ;
#14873=EDGE_CURVE('',#12084,#12085,#5990,.T.) ;
#14874=EDGE_CURVE('',#12085,#12086,#10738,.T.) ;
#14875=EDGE_CURVE('',#12086,#12087,#5991,.T.) ;
#14876=EDGE_CURVE('',#12087,#12088,#5992,.T.) ;
#14877=EDGE_CURVE('',#12088,#12089,#10739,.T.) ;
#14878=EDGE_CURVE('',#12089,#12090,#5993,.T.) ;
#14879=EDGE_CURVE('',#12090,#12091,#5994,.T.) ;
#14880=EDGE_CURVE('',#12091,#12092,#10740,.T.) ;
#14881=EDGE_CURVE('',#12092,#12093,#5995,.T.) ;
#14882=EDGE_CURVE('',#12093,#12094,#5996,.T.) ;
#14883=EDGE_CURVE('',#12094,#12095,#10741,.T.) ;
#14884=EDGE_CURVE('',#12095,#12096,#5997,.T.) ;
#14885=EDGE_CURVE('',#12096,#12097,#5998,.T.) ;
#14886=EDGE_CURVE('',#12097,#12098,#5999,.T.) ;
#14887=EDGE_CURVE('',#12098,#12099,#10742,.T.) ;
#14888=EDGE_CURVE('',#12099,#12100,#6000,.T.) ;
#14889=EDGE_CURVE('',#12100,#12101,#6001,.T.) ;
#14890=EDGE_CURVE('',#12101,#12102,#10743,.T.) ;
#14891=EDGE_CURVE('',#12102,#12103,#6002,.T.) ;
#14892=EDGE_CURVE('',#12103,#12104,#6003,.T.) ;
#14893=EDGE_CURVE('',#12104,#12105,#10744,.T.) ;
#14894=EDGE_CURVE('',#12105,#12106,#6004,.T.) ;
#14895=EDGE_CURVE('',#12106,#12107,#6005,.T.) ;
#14896=EDGE_CURVE('',#12107,#12108,#10745,.T.) ;
#14897=EDGE_CURVE('',#12108,#12109,#6006,.T.) ;
#14898=EDGE_CURVE('',#12109,#12110,#6007,.T.) ;
#14899=EDGE_CURVE('',#12110,#12111,#10746,.T.) ;
#14900=EDGE_CURVE('',#12111,#12112,#6008,.T.) ;
#14901=EDGE_CURVE('',#12112,#12113,#6009,.T.) ;
#14902=EDGE_CURVE('',#12113,#12114,#10747,.T.) ;
#14903=EDGE_CURVE('',#12114,#12115,#6010,.T.) ;
#14904=EDGE_CURVE('',#12115,#12116,#6011,.T.) ;
#14905=EDGE_CURVE('',#12116,#12117,#10748,.T.) ;
#14906=EDGE_CURVE('',#12117,#12118,#6012,.T.) ;
#14907=EDGE_CURVE('',#12118,#12119,#6013,.T.) ;
#14908=EDGE_CURVE('',#12119,#12120,#6014,.T.) ;
#14909=EDGE_CURVE('',#12120,#12121,#10749,.T.) ;
#14910=EDGE_CURVE('',#12121,#12122,#6015,.T.) ;
#14911=EDGE_CURVE('',#12122,#12123,#6016,.T.) ;
#14912=EDGE_CURVE('',#12123,#12124,#10750,.T.) ;
#14913=EDGE_CURVE('',#12124,#12125,#6017,.T.) ;
#14914=EDGE_CURVE('',#12125,#12126,#6018,.T.) ;
#14915=EDGE_CURVE('',#12126,#12127,#10751,.T.) ;
#14916=EDGE_CURVE('',#12127,#12128,#6019,.T.) ;
#14917=EDGE_CURVE('',#12128,#12129,#6020,.T.) ;
#14918=EDGE_CURVE('',#12129,#12040,#10752,.T.) ;
#14919=EDGE_CURVE('',#12019,#12130,#10753,.T.) ;
#14920=EDGE_CURVE('',#12130,#12131,#6021,.T.) ;
#14921=EDGE_CURVE('',#12131,#12132,#6022,.T.) ;
#14922=EDGE_CURVE('',#12132,#12133,#10754,.T.) ;
#14923=EDGE_CURVE('',#12133,#12134,#6023,.T.) ;
#14924=EDGE_CURVE('',#12134,#12135,#6024,.T.) ;
#14925=EDGE_CURVE('',#12135,#12136,#10755,.T.) ;
#14926=EDGE_CURVE('',#12136,#12137,#6025,.T.) ;
#14927=EDGE_CURVE('',#12137,#12138,#6026,.T.) ;
#14928=EDGE_CURVE('',#12138,#12139,#6027,.T.) ;
#14929=EDGE_CURVE('',#12139,#12140,#10756,.T.) ;
#14930=EDGE_CURVE('',#12140,#12141,#6028,.T.) ;
#14931=EDGE_CURVE('',#12141,#12142,#6029,.T.) ;
#14932=EDGE_CURVE('',#12142,#12143,#10757,.T.) ;
#14933=EDGE_CURVE('',#12143,#12144,#6030,.T.) ;
#14934=EDGE_CURVE('',#12144,#12043,#6031,.T.) ;
#14935=EDGE_CURVE('',#12048,#12037,#6032,.T.) ;
#14936=EDGE_CURVE('',#12052,#12145,#10758,.T.) ;
#14937=EDGE_CURVE('',#12145,#12033,#6033,.T.) ;
#14938=EDGE_CURVE('',#12056,#12146,#10759,.T.) ;
#14939=EDGE_CURVE('',#12146,#12029,#6034,.T.) ;
#14940=EDGE_CURVE('',#12060,#12025,#10760,.T.) ;
#14941=EDGE_CURVE('',#12054,#12147,#6035,.T.) ;
#14942=EDGE_CURVE('',#12147,#12008,#6036,.T.) ;
#14943=EDGE_CURVE('',#12058,#12148,#6037,.T.) ;
#14944=EDGE_CURVE('',#12148,#12004,#6038,.T.) ;
#14945=EDGE_CURVE('',#12062,#12149,#6039,.T.) ;
#14946=EDGE_CURVE('',#12149,#12000,#6040,.T.) ;
#14947=EDGE_CURVE('',#12064,#12150,#6041,.T.) ;
#14948=EDGE_CURVE('',#12150,#11996,#6042,.T.) ;
#14949=EDGE_CURVE('',#12050,#12151,#6043,.T.) ;
#14950=EDGE_CURVE('',#12151,#12152,#6044,.T.) ;
#14951=EDGE_CURVE('',#12152,#12012,#10761,.T.) ;
#14952=EDGE_CURVE('',#12153,#12154,#6045,.T.) ;
#14953=EDGE_CURVE('',#12154,#12155,#10762,.T.) ;
#14954=EDGE_CURVE('',#12155,#12153,#6046,.T.) ;
#14955=EDGE_CURVE('',#12156,#12157,#6047,.T.) ;
#14956=EDGE_CURVE('',#12157,#12158,#6048,.T.) ;
#14957=EDGE_CURVE('',#12158,#12159,#6049,.T.) ;
#14958=EDGE_CURVE('',#12159,#12156,#6050,.T.) ;
#14959=EDGE_CURVE('',#12160,#12161,#6051,.T.) ;
#14960=EDGE_CURVE('',#12161,#12162,#6052,.T.) ;
#14961=EDGE_CURVE('',#12162,#12163,#6053,.T.) ;
#14962=EDGE_CURVE('',#12163,#12160,#6054,.T.) ;
#14963=EDGE_CURVE('',#12164,#12165,#6055,.T.) ;
#14964=EDGE_CURVE('',#12165,#12166,#6056,.T.) ;
#14965=EDGE_CURVE('',#12166,#12167,#6057,.T.) ;
#14966=EDGE_CURVE('',#12167,#12164,#6058,.T.) ;
#14967=EDGE_CURVE('',#12168,#12169,#6059,.T.) ;
#14968=EDGE_CURVE('',#12169,#12170,#6060,.T.) ;
#14969=EDGE_CURVE('',#12170,#12171,#6061,.T.) ;
#14970=EDGE_CURVE('',#12171,#12168,#6062,.T.) ;
#14971=EDGE_CURVE('',#12172,#12173,#6063,.T.) ;
#14972=EDGE_CURVE('',#12173,#12174,#6064,.T.) ;
#14973=EDGE_CURVE('',#12174,#12175,#10763,.T.) ;
#14974=EDGE_CURVE('',#12175,#12172,#6065,.T.) ;
#14975=EDGE_CURVE('',#12176,#12177,#6066,.T.) ;
#14976=EDGE_CURVE('',#12177,#12178,#6067,.T.) ;
#14977=EDGE_CURVE('',#12178,#12179,#10764,.T.) ;
#14978=EDGE_CURVE('',#12179,#12176,#6068,.T.) ;
#14979=EDGE_CURVE('',#12180,#12181,#6069,.T.) ;
#14980=EDGE_CURVE('',#12181,#12182,#6070,.T.) ;
#14981=EDGE_CURVE('',#12182,#12183,#6071,.T.) ;
#14982=EDGE_CURVE('',#12183,#12184,#10765,.T.) ;
#14983=EDGE_CURVE('',#12184,#12180,#6072,.T.) ;
#14984=EDGE_CURVE('',#12185,#12186,#6073,.T.) ;
#14985=EDGE_CURVE('',#12186,#12187,#10766,.T.) ;
#14986=EDGE_CURVE('',#12187,#12185,#6074,.T.) ;
#14987=EDGE_CURVE('',#12188,#12189,#10767,.T.) ;
#14988=EDGE_CURVE('',#12189,#12190,#6075,.T.) ;
#14989=EDGE_CURVE('',#12190,#12191,#6076,.T.) ;
#14990=EDGE_CURVE('',#12191,#12188,#6077,.T.) ;
#14991=EDGE_CURVE('',#12192,#12193,#6078,.T.) ;
#14992=EDGE_CURVE('',#12193,#12194,#6079,.T.) ;
#14993=EDGE_CURVE('',#12194,#12195,#6080,.T.) ;
#14994=EDGE_CURVE('',#12195,#12192,#6081,.T.) ;
#14995=EDGE_CURVE('',#12196,#12197,#6082,.T.) ;
#14996=EDGE_CURVE('',#12197,#12198,#6083,.T.) ;
#14997=EDGE_CURVE('',#12198,#12199,#6084,.T.) ;
#14998=EDGE_CURVE('',#12199,#12196,#6085,.T.) ;
#14999=EDGE_CURVE('',#12200,#12201,#6086,.T.) ;
#15000=EDGE_CURVE('',#12201,#12202,#6087,.T.) ;
#15001=EDGE_CURVE('',#12202,#12203,#6088,.T.) ;
#15002=EDGE_CURVE('',#12203,#12200,#6089,.T.) ;
#15003=EDGE_CURVE('',#12204,#12205,#6090,.T.) ;
#15004=EDGE_CURVE('',#12205,#12206,#6091,.T.) ;
#15005=EDGE_CURVE('',#12206,#12207,#6092,.T.) ;
#15006=EDGE_CURVE('',#12207,#12204,#6093,.T.) ;
#15007=EDGE_CURVE('',#12208,#12209,#6094,.T.) ;
#15008=EDGE_CURVE('',#12209,#12210,#6095,.T.) ;
#15009=EDGE_CURVE('',#12210,#12211,#6096,.T.) ;
#15010=EDGE_CURVE('',#12211,#12208,#6097,.T.) ;
#15011=EDGE_CURVE('',#12212,#12213,#6098,.T.) ;
#15012=EDGE_CURVE('',#12213,#12214,#6099,.T.) ;
#15013=EDGE_CURVE('',#12214,#12215,#10768,.T.) ;
#15014=EDGE_CURVE('',#12215,#12212,#6100,.T.) ;
#15015=EDGE_CURVE('',#12216,#12217,#6101,.T.) ;
#15016=EDGE_CURVE('',#12217,#12218,#6102,.T.) ;
#15017=EDGE_CURVE('',#12218,#12219,#6103,.T.) ;
#15018=EDGE_CURVE('',#12219,#12216,#6104,.T.) ;
#15019=EDGE_CURVE('',#12220,#12221,#6105,.T.) ;
#15020=EDGE_CURVE('',#12221,#12222,#6106,.T.) ;
#15021=EDGE_CURVE('',#12222,#12223,#6107,.T.) ;
#15022=EDGE_CURVE('',#12223,#12220,#6108,.T.) ;
#15023=EDGE_CURVE('',#12224,#12225,#6109,.T.) ;
#15024=EDGE_CURVE('',#12225,#12226,#10769,.T.) ;
#15025=EDGE_CURVE('',#12226,#12224,#6110,.T.) ;
#15026=EDGE_CURVE('',#12227,#12228,#6111,.T.) ;
#15027=EDGE_CURVE('',#12228,#12229,#6112,.T.) ;
#15028=EDGE_CURVE('',#12229,#12230,#10770,.T.) ;
#15029=EDGE_CURVE('',#12230,#12231,#6113,.T.) ;
#15030=EDGE_CURVE('',#12231,#12227,#6114,.T.) ;
#15031=EDGE_CURVE('',#12232,#12233,#6115,.T.) ;
#15032=EDGE_CURVE('',#12233,#12234,#10771,.T.) ;
#15033=EDGE_CURVE('',#12234,#12232,#6116,.T.) ;
#15034=EDGE_CURVE('',#12235,#12236,#6117,.T.) ;
#15035=EDGE_CURVE('',#12236,#12237,#6118,.T.) ;
#15036=EDGE_CURVE('',#12237,#12238,#6119,.T.) ;
#15037=EDGE_CURVE('',#12238,#12235,#6120,.T.) ;
#15038=EDGE_CURVE('',#12239,#12240,#6121,.T.) ;
#15039=EDGE_CURVE('',#12240,#12241,#10772,.T.) ;
#15040=EDGE_CURVE('',#12241,#12239,#6122,.T.) ;
#15041=EDGE_CURVE('',#12242,#12243,#6123,.T.) ;
#15042=EDGE_CURVE('',#12243,#12244,#6124,.T.) ;
#15043=EDGE_CURVE('',#12244,#12245,#10773,.T.) ;
#15044=EDGE_CURVE('',#12245,#12242,#6125,.T.) ;
#15045=EDGE_CURVE('',#12246,#12247,#6126,.T.) ;
#15046=EDGE_CURVE('',#12247,#12248,#6127,.T.) ;
#15047=EDGE_CURVE('',#12248,#12249,#6128,.T.) ;
#15048=EDGE_CURVE('',#12249,#12246,#6129,.T.) ;
#15049=EDGE_CURVE('',#12250,#12251,#6130,.T.) ;
#15050=EDGE_CURVE('',#12251,#12252,#6131,.T.) ;
#15051=EDGE_CURVE('',#12252,#12253,#6132,.T.) ;
#15052=EDGE_CURVE('',#12253,#12250,#6133,.T.) ;
#15053=EDGE_CURVE('',#12254,#12255,#6134,.T.) ;
#15054=EDGE_CURVE('',#12255,#12256,#6135,.T.) ;
#15055=EDGE_CURVE('',#12256,#12257,#6136,.T.) ;
#15056=EDGE_CURVE('',#12257,#12254,#6137,.T.) ;
#15057=EDGE_CURVE('',#12258,#12259,#6138,.T.) ;
#15058=EDGE_CURVE('',#12259,#12260,#6139,.T.) ;
#15059=EDGE_CURVE('',#12260,#12261,#6140,.T.) ;
#15060=EDGE_CURVE('',#12261,#12258,#6141,.T.) ;
#15061=EDGE_CURVE('',#12262,#12263,#6142,.T.) ;
#15062=EDGE_CURVE('',#12263,#12264,#6143,.T.) ;
#15063=EDGE_CURVE('',#12264,#12265,#6144,.T.) ;
#15064=EDGE_CURVE('',#12265,#12262,#6145,.T.) ;
#15065=EDGE_CURVE('',#12266,#12267,#6146,.T.) ;
#15066=EDGE_CURVE('',#12267,#12268,#6147,.T.) ;
#15067=EDGE_CURVE('',#12268,#12269,#6148,.T.) ;
#15068=EDGE_CURVE('',#12269,#12266,#6149,.T.) ;
#15069=EDGE_CURVE('',#12270,#12271,#6150,.T.) ;
#15070=EDGE_CURVE('',#12271,#12272,#6151,.T.) ;
#15071=EDGE_CURVE('',#12272,#12270,#10774,.T.) ;
#15072=EDGE_CURVE('',#12273,#12274,#6152,.T.) ;
#15073=EDGE_CURVE('',#12274,#12275,#6153,.T.) ;
#15074=EDGE_CURVE('',#12275,#12276,#6154,.T.) ;
#15075=EDGE_CURVE('',#12276,#12273,#6155,.T.) ;
#15076=EDGE_CURVE('',#12277,#12278,#10775,.T.) ;
#15077=EDGE_CURVE('',#12278,#12279,#6156,.T.) ;
#15078=EDGE_CURVE('',#12279,#12280,#6157,.T.) ;
#15079=EDGE_CURVE('',#12280,#12277,#6158,.T.) ;
#15080=EDGE_CURVE('',#12281,#12282,#6159,.T.) ;
#15081=EDGE_CURVE('',#12282,#12283,#6160,.T.) ;
#15082=EDGE_CURVE('',#12283,#12284,#6161,.T.) ;
#15083=EDGE_CURVE('',#12284,#12281,#6162,.T.) ;
#15084=EDGE_CURVE('',#12285,#12286,#6163,.T.) ;
#15085=EDGE_CURVE('',#12286,#12287,#6164,.T.) ;
#15086=EDGE_CURVE('',#12287,#12288,#6165,.T.) ;
#15087=EDGE_CURVE('',#12288,#12285,#6166,.T.) ;
#15088=EDGE_CURVE('',#12289,#12290,#6167,.T.) ;
#15089=EDGE_CURVE('',#12290,#12291,#6168,.T.) ;
#15090=EDGE_CURVE('',#12291,#12292,#6169,.T.) ;
#15091=EDGE_CURVE('',#12292,#12289,#6170,.T.) ;
#15092=EDGE_CURVE('',#12293,#12294,#6171,.T.) ;
#15093=EDGE_CURVE('',#12294,#12295,#6172,.T.) ;
#15094=EDGE_CURVE('',#12295,#12296,#6173,.T.) ;
#15095=EDGE_CURVE('',#12296,#12293,#6174,.T.) ;
#15096=EDGE_CURVE('',#12297,#12298,#6175,.T.) ;
#15097=EDGE_CURVE('',#12298,#12299,#6176,.T.) ;
#15098=EDGE_CURVE('',#12299,#12300,#6177,.T.) ;
#15099=EDGE_CURVE('',#12300,#12297,#6178,.T.) ;
#15100=EDGE_CURVE('',#12301,#12302,#6179,.T.) ;
#15101=EDGE_CURVE('',#12302,#12303,#6180,.T.) ;
#15102=EDGE_CURVE('',#12303,#12304,#6181,.T.) ;
#15103=EDGE_CURVE('',#12304,#12301,#6182,.T.) ;
#15104=EDGE_CURVE('',#12305,#12306,#6183,.T.) ;
#15105=EDGE_CURVE('',#12306,#12307,#6184,.T.) ;
#15106=EDGE_CURVE('',#12307,#12308,#6185,.T.) ;
#15107=EDGE_CURVE('',#12308,#12305,#6186,.T.) ;
#15108=EDGE_CURVE('',#12309,#12310,#6187,.T.) ;
#15109=EDGE_CURVE('',#12310,#12311,#6188,.T.) ;
#15110=EDGE_CURVE('',#12311,#12312,#6189,.T.) ;
#15111=EDGE_CURVE('',#12312,#12309,#6190,.T.) ;
#15112=EDGE_CURVE('',#12313,#12314,#6191,.T.) ;
#15113=EDGE_CURVE('',#12314,#12315,#6192,.T.) ;
#15114=EDGE_CURVE('',#12315,#12316,#6193,.T.) ;
#15115=EDGE_CURVE('',#12316,#12313,#6194,.T.) ;
#15116=EDGE_CURVE('',#11994,#12317,#10776,.T.) ;
#15117=EDGE_CURVE('',#12317,#12318,#6195,.T.) ;
#15118=EDGE_CURVE('',#12318,#12319,#6196,.T.) ;
#15119=EDGE_CURVE('',#12319,#11992,#6197,.T.) ;
#15120=EDGE_CURVE('',#12320,#11993,#10777,.T.) ;
#15121=EDGE_CURVE('',#12320,#12317,#6198,.T.) ;
#15122=EDGE_CURVE('',#12044,#12321,#6199,.T.) ;
#15123=EDGE_CURVE('',#12321,#12322,#6200,.T.) ;
#15124=EDGE_CURVE('',#12322,#12323,#10778,.T.) ;
#15125=EDGE_CURVE('',#12323,#12324,#6201,.T.) ;
#15126=EDGE_CURVE('',#12324,#12325,#6202,.T.) ;
#15127=EDGE_CURVE('',#12325,#12326,#10779,.T.) ;
#15128=EDGE_CURVE('',#12326,#12327,#6203,.T.) ;
#15129=EDGE_CURVE('',#12327,#12328,#6204,.T.) ;
#15130=EDGE_CURVE('',#12328,#12329,#6205,.T.) ;
#15131=EDGE_CURVE('',#12329,#12330,#10780,.T.) ;
#15132=EDGE_CURVE('',#12330,#12331,#6206,.T.) ;
#15133=EDGE_CURVE('',#12331,#12332,#6207,.T.) ;
#15134=EDGE_CURVE('',#12332,#12333,#10781,.T.) ;
#15135=EDGE_CURVE('',#12333,#12334,#6208,.T.) ;
#15136=EDGE_CURVE('',#12334,#12335,#6209,.T.) ;
#15137=EDGE_CURVE('',#12335,#12020,#10782,.T.) ;
#15138=EDGE_CURVE('',#12039,#12336,#10783,.T.) ;
#15139=EDGE_CURVE('',#12336,#12337,#6210,.T.) ;
#15140=EDGE_CURVE('',#12337,#12338,#6211,.T.) ;
#15141=EDGE_CURVE('',#12338,#12339,#10784,.T.) ;
#15142=EDGE_CURVE('',#12339,#12340,#6212,.T.) ;
#15143=EDGE_CURVE('',#12340,#12341,#6213,.T.) ;
#15144=EDGE_CURVE('',#12341,#12342,#10785,.T.) ;
#15145=EDGE_CURVE('',#12342,#12343,#6214,.T.) ;
#15146=EDGE_CURVE('',#12343,#12344,#6215,.T.) ;
#15147=EDGE_CURVE('',#12344,#12345,#10786,.T.) ;
#15148=EDGE_CURVE('',#12345,#12346,#6216,.T.) ;
#15149=EDGE_CURVE('',#12346,#12347,#6217,.T.) ;
#15150=EDGE_CURVE('',#12347,#12348,#6218,.T.) ;
#15151=EDGE_CURVE('',#12348,#12349,#10787,.T.) ;
#15152=EDGE_CURVE('',#12349,#12350,#6219,.T.) ;
#15153=EDGE_CURVE('',#12350,#12351,#6220,.T.) ;
#15154=EDGE_CURVE('',#12351,#12352,#10788,.T.) ;
#15155=EDGE_CURVE('',#12352,#12353,#6221,.T.) ;
#15156=EDGE_CURVE('',#12353,#12354,#6222,.T.) ;
#15157=EDGE_CURVE('',#12354,#12355,#10789,.T.) ;
#15158=EDGE_CURVE('',#12355,#12356,#6223,.T.) ;
#15159=EDGE_CURVE('',#12356,#12357,#6224,.T.) ;
#15160=EDGE_CURVE('',#12357,#12358,#10790,.T.) ;
#15161=EDGE_CURVE('',#12358,#12359,#6225,.T.) ;
#15162=EDGE_CURVE('',#12359,#12360,#6226,.T.) ;
#15163=EDGE_CURVE('',#12360,#12361,#10791,.T.) ;
#15164=EDGE_CURVE('',#12361,#12362,#6227,.T.) ;
#15165=EDGE_CURVE('',#12362,#12363,#6228,.T.) ;
#15166=EDGE_CURVE('',#12363,#12364,#10792,.T.) ;
#15167=EDGE_CURVE('',#12364,#12365,#6229,.T.) ;
#15168=EDGE_CURVE('',#12365,#12366,#6230,.T.) ;
#15169=EDGE_CURVE('',#12366,#12367,#10793,.T.) ;
#15170=EDGE_CURVE('',#12367,#12368,#6231,.T.) ;
#15171=EDGE_CURVE('',#12368,#12369,#6232,.T.) ;
#15172=EDGE_CURVE('',#12369,#12370,#6233,.T.) ;
#15173=EDGE_CURVE('',#12370,#12371,#10794,.T.) ;
#15174=EDGE_CURVE('',#12371,#12372,#6234,.T.) ;
#15175=EDGE_CURVE('',#12372,#12373,#6235,.T.) ;
#15176=EDGE_CURVE('',#12373,#12374,#10795,.T.) ;
#15177=EDGE_CURVE('',#12374,#12375,#6236,.T.) ;
#15178=EDGE_CURVE('',#12375,#12376,#6237,.T.) ;
#15179=EDGE_CURVE('',#12376,#12377,#10796,.T.) ;
#15180=EDGE_CURVE('',#12377,#12378,#6238,.T.) ;
#15181=EDGE_CURVE('',#12378,#12379,#6239,.T.) ;
#15182=EDGE_CURVE('',#12379,#12380,#10797,.T.) ;
#15183=EDGE_CURVE('',#12380,#12381,#6240,.T.) ;
#15184=EDGE_CURVE('',#12381,#12382,#6241,.T.) ;
#15185=EDGE_CURVE('',#12382,#12383,#10798,.T.) ;
#15186=EDGE_CURVE('',#12383,#12384,#6242,.T.) ;
#15187=EDGE_CURVE('',#12384,#12385,#6243,.T.) ;
#15188=EDGE_CURVE('',#12385,#12386,#10799,.T.) ;
#15189=EDGE_CURVE('',#12386,#12387,#6244,.T.) ;
#15190=EDGE_CURVE('',#12387,#12388,#6245,.T.) ;
#15191=EDGE_CURVE('',#12388,#12389,#10800,.T.) ;
#15192=EDGE_CURVE('',#12389,#12390,#6246,.T.) ;
#15193=EDGE_CURVE('',#12390,#12391,#6247,.T.) ;
#15194=EDGE_CURVE('',#12391,#12392,#6248,.T.) ;
#15195=EDGE_CURVE('',#12392,#12393,#10801,.T.) ;
#15196=EDGE_CURVE('',#12393,#12394,#6249,.T.) ;
#15197=EDGE_CURVE('',#12394,#12395,#6250,.T.) ;
#15198=EDGE_CURVE('',#12395,#12396,#10802,.T.) ;
#15199=EDGE_CURVE('',#12396,#12397,#6251,.T.) ;
#15200=EDGE_CURVE('',#12397,#12398,#6252,.T.) ;
#15201=EDGE_CURVE('',#12398,#12399,#10803,.T.) ;
#15202=EDGE_CURVE('',#12399,#12400,#6253,.T.) ;
#15203=EDGE_CURVE('',#12400,#12045,#6254,.T.) ;
#15204=EDGE_CURVE('',#12007,#12401,#6255,.T.) ;
#15205=EDGE_CURVE('',#12401,#12053,#6256,.T.) ;
#15206=EDGE_CURVE('',#12003,#12402,#6257,.T.) ;
#15207=EDGE_CURVE('',#12402,#12057,#6258,.T.) ;
#15208=EDGE_CURVE('',#11999,#12403,#6259,.T.) ;
#15209=EDGE_CURVE('',#12403,#12061,#6260,.T.) ;
#15210=EDGE_CURVE('',#11995,#12404,#6261,.T.) ;
#15211=EDGE_CURVE('',#12404,#12063,#6262,.T.) ;
#15212=EDGE_CURVE('',#12011,#12405,#10804,.T.) ;
#15213=EDGE_CURVE('',#12405,#12406,#6263,.T.) ;
#15214=EDGE_CURVE('',#12406,#12049,#6264,.T.) ;
#15215=EDGE_CURVE('',#12034,#12407,#6265,.T.) ;
#15216=EDGE_CURVE('',#12407,#12051,#10805,.T.) ;
#15217=EDGE_CURVE('',#12030,#12408,#6266,.T.) ;
#15218=EDGE_CURVE('',#12408,#12055,#10806,.T.) ;
#15219=EDGE_CURVE('',#12026,#12059,#10807,.T.) ;
#15220=EDGE_CURVE('',#11991,#12409,#6267,.T.) ;
#15221=EDGE_CURVE('',#12409,#12410,#6268,.T.) ;
#15222=EDGE_CURVE('',#12410,#12320,#6269,.T.) ;
#15223=EDGE_CURVE('',#12038,#12047,#6270,.T.) ;
#15224=EDGE_CURVE('',#12411,#12412,#6271,.T.) ;
#15225=EDGE_CURVE('',#12412,#12413,#10808,.T.) ;
#15226=EDGE_CURVE('',#12413,#12414,#6272,.T.) ;
#15227=EDGE_CURVE('',#12414,#12415,#6273,.T.) ;
#15228=EDGE_CURVE('',#12415,#12411,#6274,.T.) ;
#15229=EDGE_CURVE('',#12416,#12417,#6275,.T.) ;
#15230=EDGE_CURVE('',#12417,#12418,#6276,.T.) ;
#15231=EDGE_CURVE('',#12418,#12419,#6277,.T.) ;
#15232=EDGE_CURVE('',#12419,#12416,#6278,.T.) ;
#15233=EDGE_CURVE('',#12420,#12421,#6279,.T.) ;
#15234=EDGE_CURVE('',#12421,#12422,#6280,.T.) ;
#15235=EDGE_CURVE('',#12422,#12423,#6281,.T.) ;
#15236=EDGE_CURVE('',#12423,#12420,#6282,.T.) ;
#15237=EDGE_CURVE('',#12424,#12425,#6283,.T.) ;
#15238=EDGE_CURVE('',#12425,#12426,#6284,.T.) ;
#15239=EDGE_CURVE('',#12426,#12427,#6285,.T.) ;
#15240=EDGE_CURVE('',#12427,#12424,#6286,.T.) ;
#15241=EDGE_CURVE('',#12428,#12429,#6287,.T.) ;
#15242=EDGE_CURVE('',#12429,#12430,#6288,.T.) ;
#15243=EDGE_CURVE('',#12430,#12431,#6289,.T.) ;
#15244=EDGE_CURVE('',#12431,#12428,#6290,.T.) ;
#15245=EDGE_CURVE('',#12432,#12433,#6291,.T.) ;
#15246=EDGE_CURVE('',#12433,#12434,#10809,.T.) ;
#15247=EDGE_CURVE('',#12434,#12432,#6292,.T.) ;
#15248=EDGE_CURVE('',#12435,#12436,#6293,.T.) ;
#15249=EDGE_CURVE('',#12436,#12437,#6294,.T.) ;
#15250=EDGE_CURVE('',#12437,#12438,#6295,.T.) ;
#15251=EDGE_CURVE('',#12438,#12435,#6296,.T.) ;
#15252=EDGE_CURVE('',#12439,#12440,#6297,.T.) ;
#15253=EDGE_CURVE('',#12440,#12441,#6298,.T.) ;
#15254=EDGE_CURVE('',#12441,#12442,#6299,.T.) ;
#15255=EDGE_CURVE('',#12442,#12439,#6300,.T.) ;
#15256=EDGE_CURVE('',#12443,#12444,#6301,.T.) ;
#15257=EDGE_CURVE('',#12444,#12445,#6302,.T.) ;
#15258=EDGE_CURVE('',#12445,#12446,#6303,.T.) ;
#15259=EDGE_CURVE('',#12446,#12443,#6304,.T.) ;
#15260=EDGE_CURVE('',#12447,#12448,#6305,.T.) ;
#15261=EDGE_CURVE('',#12448,#12449,#6306,.T.) ;
#15262=EDGE_CURVE('',#12449,#12450,#6307,.T.) ;
#15263=EDGE_CURVE('',#12450,#12447,#6308,.T.) ;
#15264=EDGE_CURVE('',#12451,#12452,#6309,.T.) ;
#15265=EDGE_CURVE('',#12452,#12453,#6310,.T.) ;
#15266=EDGE_CURVE('',#12453,#12454,#6311,.T.) ;
#15267=EDGE_CURVE('',#12454,#12451,#6312,.T.) ;
#15268=EDGE_CURVE('',#12455,#12456,#6313,.T.) ;
#15269=EDGE_CURVE('',#12456,#12457,#6314,.T.) ;
#15270=EDGE_CURVE('',#12457,#12458,#6315,.T.) ;
#15271=EDGE_CURVE('',#12458,#12455,#6316,.T.) ;
#15272=EDGE_CURVE('',#12459,#12460,#6317,.T.) ;
#15273=EDGE_CURVE('',#12460,#12461,#6318,.T.) ;
#15274=EDGE_CURVE('',#12461,#12462,#6319,.T.) ;
#15275=EDGE_CURVE('',#12462,#12459,#10810,.T.) ;
#15276=EDGE_CURVE('',#12463,#12464,#6320,.T.) ;
#15277=EDGE_CURVE('',#12464,#12465,#10811,.T.) ;
#15278=EDGE_CURVE('',#12465,#12466,#6321,.T.) ;
#15279=EDGE_CURVE('',#12466,#12463,#6322,.T.) ;
#15280=EDGE_CURVE('',#12467,#12468,#6323,.T.) ;
#15281=EDGE_CURVE('',#12468,#12469,#6324,.T.) ;
#15282=EDGE_CURVE('',#12469,#12470,#10812,.T.) ;
#15283=EDGE_CURVE('',#12470,#12471,#6325,.T.) ;
#15284=EDGE_CURVE('',#12471,#12467,#6326,.T.) ;
#15285=EDGE_CURVE('',#12472,#12473,#6327,.T.) ;
#15286=EDGE_CURVE('',#12473,#12474,#10813,.T.) ;
#15287=EDGE_CURVE('',#12474,#12472,#6328,.T.) ;
#15288=EDGE_CURVE('',#12475,#12476,#6329,.T.) ;
#15289=EDGE_CURVE('',#12476,#12477,#6330,.T.) ;
#15290=EDGE_CURVE('',#12477,#12478,#6331,.T.) ;
#15291=EDGE_CURVE('',#12478,#12475,#6332,.T.) ;
#15292=EDGE_CURVE('',#12479,#12480,#6333,.T.) ;
#15293=EDGE_CURVE('',#12480,#12481,#10814,.T.) ;
#15294=EDGE_CURVE('',#12481,#12479,#6334,.T.) ;
#15295=EDGE_CURVE('',#12482,#12483,#6335,.T.) ;
#15296=EDGE_CURVE('',#12483,#12484,#6336,.T.) ;
#15297=EDGE_CURVE('',#12484,#12485,#6337,.T.) ;
#15298=EDGE_CURVE('',#12485,#12482,#6338,.T.) ;
#15299=EDGE_CURVE('',#12486,#12487,#6339,.T.) ;
#15300=EDGE_CURVE('',#12487,#12488,#6340,.T.) ;
#15301=EDGE_CURVE('',#12488,#12489,#6341,.T.) ;
#15302=EDGE_CURVE('',#12489,#12486,#6342,.T.) ;
#15303=EDGE_CURVE('',#12490,#12491,#6343,.T.) ;
#15304=EDGE_CURVE('',#12491,#12492,#6344,.T.) ;
#15305=EDGE_CURVE('',#12492,#12493,#6345,.T.) ;
#15306=EDGE_CURVE('',#12493,#12490,#6346,.T.) ;
#15307=EDGE_CURVE('',#12494,#12495,#6347,.T.) ;
#15308=EDGE_CURVE('',#12495,#12496,#6348,.T.) ;
#15309=EDGE_CURVE('',#12496,#12497,#6349,.T.) ;
#15310=EDGE_CURVE('',#12497,#12494,#6350,.T.) ;
#15311=EDGE_CURVE('',#12498,#12499,#6351,.T.) ;
#15312=EDGE_CURVE('',#12499,#12500,#10815,.T.) ;
#15313=EDGE_CURVE('',#12500,#12501,#6352,.T.) ;
#15314=EDGE_CURVE('',#12501,#12498,#6353,.T.) ;
#15315=EDGE_CURVE('',#12502,#12503,#6354,.T.) ;
#15316=EDGE_CURVE('',#12503,#12504,#6355,.T.) ;
#15317=EDGE_CURVE('',#12504,#12505,#6356,.T.) ;
#15318=EDGE_CURVE('',#12505,#12502,#10816,.T.) ;
#15319=EDGE_CURVE('',#12506,#12507,#6357,.T.) ;
#15320=EDGE_CURVE('',#12507,#12508,#6358,.T.) ;
#15321=EDGE_CURVE('',#12508,#12509,#6359,.T.) ;
#15322=EDGE_CURVE('',#12509,#12506,#6360,.T.) ;
#15323=EDGE_CURVE('',#12510,#12511,#6361,.T.) ;
#15324=EDGE_CURVE('',#12511,#12512,#6362,.T.) ;
#15325=EDGE_CURVE('',#12512,#12513,#6363,.T.) ;
#15326=EDGE_CURVE('',#12513,#12510,#6364,.T.) ;
#15327=EDGE_CURVE('',#12514,#12515,#6365,.T.) ;
#15328=EDGE_CURVE('',#12515,#12516,#6366,.T.) ;
#15329=EDGE_CURVE('',#12516,#12517,#6367,.T.) ;
#15330=EDGE_CURVE('',#12517,#12514,#6368,.T.) ;
#15331=EDGE_CURVE('',#12518,#12519,#10817,.T.) ;
#15332=EDGE_CURVE('',#12519,#12520,#6369,.T.) ;
#15333=EDGE_CURVE('',#12520,#12518,#6370,.T.) ;
#15334=EDGE_CURVE('',#12521,#12522,#6371,.T.) ;
#15335=EDGE_CURVE('',#12522,#12523,#6372,.T.) ;
#15336=EDGE_CURVE('',#12523,#12524,#6373,.T.) ;
#15337=EDGE_CURVE('',#12524,#12521,#6374,.T.) ;
#15338=EDGE_CURVE('',#12525,#12526,#6375,.T.) ;
#15339=EDGE_CURVE('',#12526,#12527,#6376,.T.) ;
#15340=EDGE_CURVE('',#12527,#12528,#6377,.T.) ;
#15341=EDGE_CURVE('',#12528,#12525,#6378,.T.) ;
#15342=EDGE_CURVE('',#12529,#12530,#6379,.T.) ;
#15343=EDGE_CURVE('',#12530,#12531,#6380,.T.) ;
#15344=EDGE_CURVE('',#12531,#12532,#6381,.T.) ;
#15345=EDGE_CURVE('',#12532,#12529,#6382,.T.) ;
#15346=EDGE_CURVE('',#12533,#12534,#6383,.T.) ;
#15347=EDGE_CURVE('',#12534,#12535,#6384,.T.) ;
#15348=EDGE_CURVE('',#12535,#12536,#6385,.T.) ;
#15349=EDGE_CURVE('',#12536,#12533,#6386,.T.) ;
#15350=EDGE_CURVE('',#12537,#12538,#6387,.T.) ;
#15351=EDGE_CURVE('',#12538,#12539,#6388,.T.) ;
#15352=EDGE_CURVE('',#12539,#12540,#6389,.T.) ;
#15353=EDGE_CURVE('',#12540,#12537,#6390,.T.) ;
#15354=EDGE_CURVE('',#12541,#12542,#6391,.T.) ;
#15355=EDGE_CURVE('',#12542,#12543,#6392,.T.) ;
#15356=EDGE_CURVE('',#12543,#12544,#6393,.T.) ;
#15357=EDGE_CURVE('',#12544,#12541,#6394,.T.) ;
#15358=EDGE_CURVE('',#12545,#12546,#6395,.T.) ;
#15359=EDGE_CURVE('',#12546,#12547,#6396,.T.) ;
#15360=EDGE_CURVE('',#12547,#12548,#6397,.T.) ;
#15361=EDGE_CURVE('',#12548,#12545,#6398,.T.) ;
#15362=EDGE_CURVE('',#12549,#12550,#6399,.T.) ;
#15363=EDGE_CURVE('',#12550,#12551,#6400,.T.) ;
#15364=EDGE_CURVE('',#12551,#12552,#6401,.T.) ;
#15365=EDGE_CURVE('',#12552,#12549,#6402,.T.) ;
#15366=EDGE_CURVE('',#12553,#12554,#6403,.T.) ;
#15367=EDGE_CURVE('',#12554,#12555,#6404,.T.) ;
#15368=EDGE_CURVE('',#12555,#12556,#6405,.T.) ;
#15369=EDGE_CURVE('',#12556,#12553,#6406,.T.) ;
#15370=EDGE_CURVE('',#12557,#12558,#6407,.T.) ;
#15371=EDGE_CURVE('',#12558,#12559,#10818,.T.) ;
#15372=EDGE_CURVE('',#12559,#12557,#6408,.T.) ;
#15373=EDGE_CURVE('',#12560,#12561,#6409,.T.) ;
#15374=EDGE_CURVE('',#12561,#12562,#10819,.T.) ;
#15375=EDGE_CURVE('',#12562,#12560,#6410,.T.) ;
#15376=EDGE_CURVE('',#12563,#12564,#6411,.T.) ;
#15377=EDGE_CURVE('',#12564,#12565,#10820,.T.) ;
#15378=EDGE_CURVE('',#12565,#12566,#6412,.T.) ;
#15379=EDGE_CURVE('',#12566,#12563,#6413,.T.) ;
#15380=EDGE_CURVE('',#12567,#12568,#6414,.T.) ;
#15381=EDGE_CURVE('',#12568,#12569,#10821,.T.) ;
#15382=EDGE_CURVE('',#12569,#12570,#6415,.T.) ;
#15383=EDGE_CURVE('',#12570,#12567,#6416,.T.) ;
#15384=EDGE_CURVE('',#12571,#12572,#6417,.T.) ;
#15385=EDGE_CURVE('',#12572,#12573,#6418,.T.) ;
#15386=EDGE_CURVE('',#12573,#12574,#6419,.T.) ;
#15387=EDGE_CURVE('',#12574,#12571,#6420,.T.) ;
#15388=EDGE_CURVE('',#12129,#12336,#6421,.T.) ;
#15389=EDGE_CURVE('',#12335,#12130,#6422,.T.) ;
#15390=EDGE_CURVE('',#12065,#12400,#6423,.T.) ;
#15391=EDGE_CURVE('',#12180,#12411,#6424,.T.) ;
#15392=EDGE_CURVE('',#12412,#12184,#6425,.T.) ;
#15393=EDGE_CURVE('',#12164,#12545,#6426,.T.) ;
#15394=EDGE_CURVE('',#12546,#12167,#6427,.T.) ;
#15395=EDGE_CURVE('',#12160,#12549,#6428,.T.) ;
#15396=EDGE_CURVE('',#12550,#12163,#6429,.T.) ;
#15397=EDGE_CURVE('',#12406,#12151,#6430,.T.) ;
#15398=EDGE_CURVE('',#12152,#12405,#6431,.T.) ;
#15399=EDGE_CURVE('',#12571,#12168,#6432,.T.) ;
#15400=EDGE_CURVE('',#12169,#12574,#6433,.T.) ;
#15401=EDGE_CURVE('',#12156,#12553,#6434,.T.) ;
#15402=EDGE_CURVE('',#12554,#12159,#6435,.T.) ;
#15403=EDGE_CURVE('',#12382,#12083,#6436,.T.) ;
#15404=EDGE_CURVE('',#12084,#12381,#6437,.T.) ;
#15405=EDGE_CURVE('',#12560,#12185,#6438,.T.) ;
#15406=EDGE_CURVE('',#12186,#12562,#6439,.T.) ;
#15407=EDGE_CURVE('',#12563,#12176,#6440,.T.) ;
#15408=EDGE_CURVE('',#12177,#12566,#6441,.T.) ;
#15409=EDGE_CURVE('',#12567,#12172,#6442,.T.) ;
#15410=EDGE_CURVE('',#12173,#12570,#6443,.T.) ;
#15411=EDGE_CURVE('',#12066,#12399,#6444,.T.) ;
#15412=EDGE_CURVE('',#12085,#12380,#6445,.T.) ;
#15413=EDGE_CURVE('',#12153,#12557,#6446,.T.) ;
#15414=EDGE_CURVE('',#12558,#12155,#6447,.T.) ;
#15415=EDGE_CURVE('',#12154,#12559,#6448,.T.) ;
#15416=EDGE_CURVE('',#12556,#12157,#6449,.T.) ;
#15417=EDGE_CURVE('',#12170,#12573,#6450,.T.) ;
#15418=EDGE_CURVE('',#12398,#12067,#6451,.T.) ;
#15419=EDGE_CURVE('',#12174,#12569,#6452,.T.) ;
#15420=EDGE_CURVE('',#12552,#12161,#6453,.T.) ;
#15421=EDGE_CURVE('',#12178,#12565,#6454,.T.) ;
#15422=EDGE_CURVE('',#12548,#12165,#6455,.T.) ;
#15423=EDGE_CURVE('',#12415,#12181,#6456,.T.) ;
#15424=EDGE_CURVE('',#12561,#12187,#6457,.T.) ;
#15425=EDGE_CURVE('',#12082,#12383,#6458,.T.) ;
#15426=EDGE_CURVE('',#12379,#12086,#6459,.T.) ;
#15427=EDGE_CURVE('',#12341,#12124,#6460,.T.) ;
#15428=EDGE_CURVE('',#12125,#12340,#6461,.T.) ;
#15429=EDGE_CURVE('',#12068,#12397,#6462,.T.) ;
#15430=EDGE_CURVE('',#12126,#12339,#6463,.T.) ;
#15431=EDGE_CURVE('',#12319,#12409,#6464,.T.) ;
#15432=EDGE_CURVE('',#12410,#12318,#6465,.T.) ;
#15433=EDGE_CURVE('',#12150,#12404,#6466,.T.) ;
#15434=EDGE_CURVE('',#12149,#12403,#6467,.T.) ;
#15435=EDGE_CURVE('',#12148,#12402,#6468,.T.) ;
#15436=EDGE_CURVE('',#12525,#12297,#6469,.T.) ;
#15437=EDGE_CURVE('',#12298,#12528,#6470,.T.) ;
#15438=EDGE_CURVE('',#12529,#12301,#6471,.T.) ;
#15439=EDGE_CURVE('',#12302,#12532,#6472,.T.) ;
#15440=EDGE_CURVE('',#12533,#12305,#6473,.T.) ;
#15441=EDGE_CURVE('',#12306,#12536,#6474,.T.) ;
#15442=EDGE_CURVE('',#12537,#12309,#6475,.T.) ;
#15443=EDGE_CURVE('',#12310,#12540,#6476,.T.) ;
#15444=EDGE_CURVE('',#12541,#12313,#6477,.T.) ;
#15445=EDGE_CURVE('',#12314,#12544,#6478,.T.) ;
#15446=EDGE_CURVE('',#12069,#12396,#6479,.T.) ;
#15447=EDGE_CURVE('',#12147,#12401,#6480,.T.) ;
#15448=EDGE_CURVE('',#12171,#12572,#6481,.T.) ;
#15449=EDGE_CURVE('',#12395,#12070,#6482,.T.) ;
#15450=EDGE_CURVE('',#12543,#12315,#6483,.T.) ;
#15451=EDGE_CURVE('',#12539,#12311,#6484,.T.) ;
#15452=EDGE_CURVE('',#12535,#12307,#6485,.T.) ;
#15453=EDGE_CURVE('',#12531,#12303,#6486,.T.) ;
#15454=EDGE_CURVE('',#12338,#12127,#6487,.T.) ;
#15455=EDGE_CURVE('',#12527,#12299,#6488,.T.) ;
#15456=EDGE_CURVE('',#12322,#12143,#6489,.T.) ;
#15457=EDGE_CURVE('',#12144,#12321,#6490,.T.) ;
#15458=EDGE_CURVE('',#12376,#12089,#6491,.T.) ;
#15459=EDGE_CURVE('',#12090,#12375,#6492,.T.) ;
#15460=EDGE_CURVE('',#12166,#12547,#6493,.T.) ;
#15461=EDGE_CURVE('',#12162,#12551,#6494,.T.) ;
#15462=EDGE_CURVE('',#12182,#12414,#6495,.T.) ;
#15463=EDGE_CURVE('',#12158,#12555,#6496,.T.) ;
#15464=EDGE_CURVE('',#12416,#12281,#6497,.T.) ;
#15465=EDGE_CURVE('',#12282,#12419,#6498,.T.) ;
#15466=EDGE_CURVE('',#12285,#12428,#6499,.T.) ;
#15467=EDGE_CURVE('',#12429,#12288,#6500,.T.) ;
#15468=EDGE_CURVE('',#12542,#12316,#6501,.T.) ;
#15469=EDGE_CURVE('',#12289,#12424,#6502,.T.) ;
#15470=EDGE_CURVE('',#12425,#12292,#6503,.T.) ;
#15471=EDGE_CURVE('',#12293,#12420,#6504,.T.) ;
#15472=EDGE_CURVE('',#12421,#12296,#6505,.T.) ;
#15473=EDGE_CURVE('',#12091,#12374,#6506,.T.) ;
#15474=EDGE_CURVE('',#12568,#12175,#6507,.T.) ;
#15475=EDGE_CURVE('',#12294,#12423,#6508,.T.) ;
#15476=EDGE_CURVE('',#12427,#12290,#6509,.T.) ;
#15477=EDGE_CURVE('',#12142,#12323,#6510,.T.) ;
#15478=EDGE_CURVE('',#12183,#12413,#6511,.T.) ;
#15479=EDGE_CURVE('',#12088,#12377,#6512,.T.) ;
#15480=EDGE_CURVE('',#12373,#12092,#6513,.T.) ;
#15481=EDGE_CURVE('',#12431,#12286,#6514,.T.) ;
#15482=EDGE_CURVE('',#12418,#12283,#6515,.T.) ;
#15483=EDGE_CURVE('',#12344,#12121,#6516,.T.) ;
#15484=EDGE_CURVE('',#12122,#12343,#6517,.T.) ;
#15485=EDGE_CURVE('',#12071,#12394,#6518,.T.) ;
#15486=EDGE_CURVE('',#12518,#12270,#6519,.T.) ;
#15487=EDGE_CURVE('',#12271,#12520,#6520,.T.) ;
#15488=EDGE_CURVE('',#12300,#12526,#6521,.T.) ;
#15489=EDGE_CURVE('',#12304,#12530,#6522,.T.) ;
#15490=EDGE_CURVE('',#12308,#12534,#6523,.T.) ;
#15491=EDGE_CURVE('',#12123,#12342,#6524,.T.) ;
#15492=EDGE_CURVE('',#12506,#12258,#6525,.T.) ;
#15493=EDGE_CURVE('',#12259,#12509,#6526,.T.) ;
#15494=EDGE_CURVE('',#12510,#12262,#6527,.T.) ;
#15495=EDGE_CURVE('',#12263,#12513,#6528,.T.) ;
#15496=EDGE_CURVE('',#12514,#12266,#6529,.T.) ;
#15497=EDGE_CURVE('',#12267,#12517,#6530,.T.) ;
#15498=EDGE_CURVE('',#12521,#12273,#6531,.T.) ;
#15499=EDGE_CURVE('',#12274,#12524,#6532,.T.) ;
#15500=EDGE_CURVE('',#12277,#12502,#6533,.T.) ;
#15501=EDGE_CURVE('',#12503,#12280,#6534,.T.) ;
#15502=EDGE_CURVE('',#12072,#12393,#6535,.T.) ;
#15503=EDGE_CURVE('',#12312,#12538,#6536,.T.) ;
#15504=EDGE_CURVE('',#12295,#12422,#6537,.T.) ;
#15505=EDGE_CURVE('',#12392,#12073,#6538,.T.) ;
#15506=EDGE_CURVE('',#12272,#12519,#6539,.T.) ;
#15507=EDGE_CURVE('',#12505,#12278,#6540,.T.) ;
#15508=EDGE_CURVE('',#12523,#12275,#6541,.T.) ;
#15509=EDGE_CURVE('',#12516,#12268,#6542,.T.) ;
#15510=EDGE_CURVE('',#12512,#12264,#6543,.T.) ;
#15511=EDGE_CURVE('',#12508,#12260,#6544,.T.) ;
#15512=EDGE_CURVE('',#12325,#12140,#6545,.T.) ;
#15513=EDGE_CURVE('',#12141,#12324,#6546,.T.) ;
#15514=EDGE_CURVE('',#12242,#12498,#6547,.T.) ;
#15515=EDGE_CURVE('',#12499,#12245,#6548,.T.) ;
#15516=EDGE_CURVE('',#12246,#12443,#6549,.T.) ;
#15517=EDGE_CURVE('',#12444,#12249,#6550,.T.) ;
#15518=EDGE_CURVE('',#12250,#12439,#6551,.T.) ;
#15519=EDGE_CURVE('',#12440,#12253,#6552,.T.) ;
#15520=EDGE_CURVE('',#12522,#12276,#6553,.T.) ;
#15521=EDGE_CURVE('',#12254,#12435,#6554,.T.) ;
#15522=EDGE_CURVE('',#12436,#12257,#6555,.T.) ;
#15523=EDGE_CURVE('',#12093,#12372,#6556,.T.) ;
#15524=EDGE_CURVE('',#12432,#12239,#6557,.T.) ;
#15525=EDGE_CURVE('',#12240,#12434,#6558,.T.) ;
#15526=EDGE_CURVE('',#12284,#12417,#6559,.T.) ;
#15527=EDGE_CURVE('',#12287,#12430,#6560,.T.) ;
#15528=EDGE_CURVE('',#12291,#12426,#6561,.T.) ;
#15529=EDGE_CURVE('',#12094,#12371,#6562,.T.) ;
#15530=EDGE_CURVE('',#12564,#12179,#6563,.T.) ;
#15531=EDGE_CURVE('',#12255,#12438,#6564,.T.) ;
#15532=EDGE_CURVE('',#12407,#12145,#6565,.T.) ;
#15533=EDGE_CURVE('',#12139,#12326,#6566,.T.) ;
#15534=EDGE_CURVE('',#12442,#12251,#6567,.T.) ;
#15535=EDGE_CURVE('',#12446,#12247,#6568,.T.) ;
#15536=EDGE_CURVE('',#12501,#12243,#6569,.T.) ;
#15537=EDGE_CURVE('',#12433,#12241,#6570,.T.) ;
#15538=EDGE_CURVE('',#12370,#12095,#6571,.T.) ;
#15539=EDGE_CURVE('',#12074,#12391,#6572,.T.) ;
#15540=EDGE_CURVE('',#12279,#12504,#6573,.T.) ;
#15541=EDGE_CURVE('',#12261,#12507,#6574,.T.) ;
#15542=EDGE_CURVE('',#12120,#12345,#6575,.T.) ;
#15543=EDGE_CURVE('',#12119,#12346,#6576,.T.) ;
#15544=EDGE_CURVE('',#12265,#12511,#6577,.T.) ;
#15545=EDGE_CURVE('',#12269,#12515,#6578,.T.) ;
#15546=EDGE_CURVE('',#12348,#12117,#6579,.T.) ;
#15547=EDGE_CURVE('',#12118,#12347,#6580,.T.) ;
#15548=EDGE_CURVE('',#12455,#12200,#6581,.T.) ;
#15549=EDGE_CURVE('',#12201,#12458,#6582,.T.) ;
#15550=EDGE_CURVE('',#12451,#12196,#6583,.T.) ;
#15551=EDGE_CURVE('',#12197,#12454,#6584,.T.) ;
#15552=EDGE_CURVE('',#12188,#12459,#6585,.T.) ;
#15553=EDGE_CURVE('',#12460,#12191,#6586,.T.) ;
#15554=EDGE_CURVE('',#12447,#12192,#6587,.T.) ;
#15555=EDGE_CURVE('',#12193,#12450,#6588,.T.) ;
#15556=EDGE_CURVE('',#12076,#12389,#6589,.T.) ;
#15557=EDGE_CURVE('',#12075,#12390,#6590,.T.) ;
#15558=EDGE_CURVE('',#12256,#12437,#6591,.T.) ;
#15559=EDGE_CURVE('',#12448,#12195,#6592,.T.) ;
#15560=EDGE_CURVE('',#12388,#12077,#6593,.T.) ;
#15561=EDGE_CURVE('',#12449,#12194,#6594,.T.) ;
#15562=EDGE_CURVE('',#12116,#12349,#6595,.T.) ;
#15563=EDGE_CURVE('',#12462,#12189,#6596,.T.) ;
#15564=EDGE_CURVE('',#12453,#12198,#6597,.T.) ;
#15565=EDGE_CURVE('',#12457,#12202,#6598,.T.) ;
#15566=EDGE_CURVE('',#12096,#12369,#6599,.T.) ;
#15567=EDGE_CURVE('',#12244,#12500,#6600,.T.) ;
#15568=EDGE_CURVE('',#12248,#12445,#6601,.T.) ;
#15569=EDGE_CURVE('',#12138,#12327,#6602,.T.) ;
#15570=EDGE_CURVE('',#12252,#12441,#6603,.T.) ;
#15571=EDGE_CURVE('',#12329,#12136,#6604,.T.) ;
#15572=EDGE_CURVE('',#12137,#12328,#6605,.T.) ;
#15573=EDGE_CURVE('',#12098,#12367,#6606,.T.) ;
#15574=EDGE_CURVE('',#12097,#12368,#6607,.T.) ;
#15575=EDGE_CURVE('',#12212,#12463,#6608,.T.) ;
#15576=EDGE_CURVE('',#12464,#12215,#6609,.T.) ;
#15577=EDGE_CURVE('',#12208,#12490,#6610,.T.) ;
#15578=EDGE_CURVE('',#12491,#12211,#6611,.T.) ;
#15579=EDGE_CURVE('',#12204,#12494,#6612,.T.) ;
#15580=EDGE_CURVE('',#12495,#12207,#6613,.T.) ;
#15581=EDGE_CURVE('',#12205,#12497,#6614,.T.) ;
#15582=EDGE_CURVE('',#12493,#12209,#6615,.T.) ;
#15583=EDGE_CURVE('',#12408,#12146,#6616,.T.) ;
#15584=EDGE_CURVE('',#12466,#12213,#6617,.T.) ;
#15585=EDGE_CURVE('',#12214,#12465,#6618,.T.) ;
#15586=EDGE_CURVE('',#12366,#12099,#6619,.T.) ;
#15587=EDGE_CURVE('',#12078,#12387,#6620,.T.) ;
#15588=EDGE_CURVE('',#12351,#12114,#6621,.T.) ;
#15589=EDGE_CURVE('',#12115,#12350,#6622,.T.) ;
#15590=EDGE_CURVE('',#12479,#12224,#6623,.T.) ;
#15591=EDGE_CURVE('',#12225,#12481,#6624,.T.) ;
#15592=EDGE_CURVE('',#12482,#12216,#6625,.T.) ;
#15593=EDGE_CURVE('',#12217,#12485,#6626,.T.) ;
#15594=EDGE_CURVE('',#12079,#12386,#6627,.T.) ;
#15595=EDGE_CURVE('',#12486,#12220,#6628,.T.) ;
#15596=EDGE_CURVE('',#12221,#12489,#6629,.T.) ;
#15597=EDGE_CURVE('',#12190,#12461,#6630,.T.) ;
#15598=EDGE_CURVE('',#12203,#12456,#6631,.T.) ;
#15599=EDGE_CURVE('',#12199,#12452,#6632,.T.) ;
#15600=EDGE_CURVE('',#12206,#12496,#6633,.T.) ;
#15601=EDGE_CURVE('',#12488,#12222,#6634,.T.) ;
#15602=EDGE_CURVE('',#12385,#12080,#6635,.T.) ;
#15603=EDGE_CURVE('',#12484,#12218,#6636,.T.) ;
#15604=EDGE_CURVE('',#12113,#12352,#6637,.T.) ;
#15605=EDGE_CURVE('',#12480,#12226,#6638,.T.) ;
#15606=EDGE_CURVE('',#12100,#12365,#6639,.T.) ;
#15607=EDGE_CURVE('',#12210,#12492,#6640,.T.) ;
#15608=EDGE_CURVE('',#12101,#12364,#6641,.T.) ;
#15609=EDGE_CURVE('',#12232,#12472,#6642,.T.) ;
#15610=EDGE_CURVE('',#12473,#12234,#6643,.T.) ;
#15611=EDGE_CURVE('',#12332,#12133,#6644,.T.) ;
#15612=EDGE_CURVE('',#12134,#12331,#6645,.T.) ;
#15613=EDGE_CURVE('',#12235,#12475,#6646,.T.) ;
#15614=EDGE_CURVE('',#12476,#12238,#6647,.T.) ;
#15615=EDGE_CURVE('',#12487,#12223,#6648,.T.) ;
#15616=EDGE_CURVE('',#12135,#12330,#6649,.T.) ;
#15617=EDGE_CURVE('',#12236,#12478,#6650,.T.) ;
#15618=EDGE_CURVE('',#12132,#12333,#6651,.T.) ;
#15619=EDGE_CURVE('',#12233,#12474,#6652,.T.) ;
#15620=EDGE_CURVE('',#12363,#12102,#6653,.T.) ;
#15621=EDGE_CURVE('',#12081,#12384,#6654,.T.) ;
#15622=EDGE_CURVE('',#12354,#12111,#6655,.T.) ;
#15623=EDGE_CURVE('',#12112,#12353,#6656,.T.) ;
#15624=EDGE_CURVE('',#12467,#12227,#6657,.T.) ;
#15625=EDGE_CURVE('',#12228,#12471,#6658,.T.) ;
#15626=EDGE_CURVE('',#12219,#12483,#6659,.T.) ;
#15627=EDGE_CURVE('',#12237,#12477,#6660,.T.) ;
#15628=EDGE_CURVE('',#12229,#12470,#6661,.T.) ;
#15629=EDGE_CURVE('',#12110,#12355,#6662,.T.) ;
#15630=EDGE_CURVE('',#12103,#12362,#6663,.T.) ;
#15631=EDGE_CURVE('',#12131,#12334,#6664,.T.) ;
#15632=EDGE_CURVE('',#12104,#12361,#6665,.T.) ;
#15633=EDGE_CURVE('',#12468,#12231,#6666,.T.) ;
#15634=EDGE_CURVE('',#12469,#12230,#6667,.T.) ;
#15635=EDGE_CURVE('',#12360,#12105,#6668,.T.) ;
#15636=EDGE_CURVE('',#12087,#12378,#6669,.T.) ;
#15637=EDGE_CURVE('',#12106,#12359,#6670,.T.) ;
#15638=EDGE_CURVE('',#12107,#12358,#6671,.T.) ;
#15639=EDGE_CURVE('',#12357,#12108,#6672,.T.) ;
#15640=EDGE_CURVE('',#12109,#12356,#6673,.T.) ;
#15641=EDGE_CURVE('',#12128,#12337,#6674,.T.) ;
#19001=ORIENTED_EDGE('',*,*,#14766,.F.) ;
#19002=ORIENTED_EDGE('',*,*,#14767,.F.) ;
#19003=ORIENTED_EDGE('',*,*,#14768,.F.) ;
#19004=ORIENTED_EDGE('',*,*,#14769,.F.) ;
#19005=ORIENTED_EDGE('',*,*,#14770,.F.) ;
#19006=ORIENTED_EDGE('',*,*,#14771,.F.) ;
#19007=ORIENTED_EDGE('',*,*,#14772,.F.) ;
#19008=ORIENTED_EDGE('',*,*,#14773,.F.) ;
#19009=ORIENTED_EDGE('',*,*,#14774,.F.) ;
#19010=ORIENTED_EDGE('',*,*,#14775,.F.) ;
#19011=ORIENTED_EDGE('',*,*,#14776,.F.) ;
#19012=ORIENTED_EDGE('',*,*,#14777,.F.) ;
#19013=ORIENTED_EDGE('',*,*,#14778,.F.) ;
#19014=ORIENTED_EDGE('',*,*,#14779,.F.) ;
#19015=ORIENTED_EDGE('',*,*,#14780,.F.) ;
#19016=ORIENTED_EDGE('',*,*,#14781,.F.) ;
#19017=ORIENTED_EDGE('',*,*,#14782,.F.) ;
#19018=ORIENTED_EDGE('',*,*,#14783,.F.) ;
#19019=ORIENTED_EDGE('',*,*,#14784,.F.) ;
#19020=ORIENTED_EDGE('',*,*,#14785,.F.) ;
#19021=ORIENTED_EDGE('',*,*,#14786,.F.) ;
#19022=ORIENTED_EDGE('',*,*,#14787,.F.) ;
#19023=ORIENTED_EDGE('',*,*,#14788,.F.) ;
#19024=ORIENTED_EDGE('',*,*,#14789,.F.) ;
#19025=ORIENTED_EDGE('',*,*,#14790,.F.) ;
#19026=ORIENTED_EDGE('',*,*,#14791,.F.) ;
#19027=ORIENTED_EDGE('',*,*,#14792,.F.) ;
#19028=ORIENTED_EDGE('',*,*,#14793,.F.) ;
#19029=ORIENTED_EDGE('',*,*,#14794,.F.) ;
#19030=ORIENTED_EDGE('',*,*,#14795,.F.) ;
#19031=ORIENTED_EDGE('',*,*,#14796,.T.) ;
#19032=ORIENTED_EDGE('',*,*,#14797,.F.) ;
#19033=ORIENTED_EDGE('',*,*,#14798,.F.) ;
#19034=ORIENTED_EDGE('',*,*,#14799,.F.) ;
#19035=ORIENTED_EDGE('',*,*,#14800,.F.) ;
#19036=ORIENTED_EDGE('',*,*,#14801,.F.) ;
#19037=ORIENTED_EDGE('',*,*,#14802,.F.) ;
#19038=ORIENTED_EDGE('',*,*,#14803,.F.) ;
#19039=ORIENTED_EDGE('',*,*,#14804,.F.) ;
#19040=ORIENTED_EDGE('',*,*,#14805,.F.) ;
#19041=ORIENTED_EDGE('',*,*,#14806,.F.) ;
#19042=ORIENTED_EDGE('',*,*,#14807,.F.) ;
#19043=ORIENTED_EDGE('',*,*,#14808,.F.) ;
#19044=ORIENTED_EDGE('',*,*,#14809,.F.) ;
#19045=ORIENTED_EDGE('',*,*,#14810,.F.) ;
#19046=ORIENTED_EDGE('',*,*,#14811,.F.) ;
#19047=ORIENTED_EDGE('',*,*,#14812,.F.) ;
#19048=ORIENTED_EDGE('',*,*,#14813,.F.) ;
#19049=ORIENTED_EDGE('',*,*,#14814,.F.) ;
#19050=ORIENTED_EDGE('',*,*,#14815,.F.) ;
#19051=ORIENTED_EDGE('',*,*,#14796,.F.) ;
#19052=ORIENTED_EDGE('',*,*,#14816,.F.) ;
#19053=ORIENTED_EDGE('',*,*,#14817,.F.) ;
#19054=ORIENTED_EDGE('',*,*,#14818,.F.) ;
#19055=ORIENTED_EDGE('',*,*,#14792,.T.) ;
#19056=ORIENTED_EDGE('',*,*,#14819,.F.) ;
#19057=ORIENTED_EDGE('',*,*,#14790,.T.) ;
#19058=ORIENTED_EDGE('',*,*,#14820,.F.) ;
#19059=ORIENTED_EDGE('',*,*,#14821,.T.) ;
#19060=ORIENTED_EDGE('',*,*,#14822,.F.) ;
#19061=ORIENTED_EDGE('',*,*,#14817,.T.) ;
#19062=ORIENTED_EDGE('',*,*,#14823,.F.) ;
#19063=ORIENTED_EDGE('',*,*,#14824,.T.) ;
#19064=ORIENTED_EDGE('',*,*,#14825,.F.) ;
#19065=ORIENTED_EDGE('',*,*,#14810,.T.) ;
#19066=ORIENTED_EDGE('',*,*,#14826,.F.) ;
#19067=ORIENTED_EDGE('',*,*,#14827,.T.) ;
#19068=ORIENTED_EDGE('',*,*,#14828,.F.) ;
#19069=ORIENTED_EDGE('',*,*,#14788,.T.) ;
#19070=ORIENTED_EDGE('',*,*,#14829,.F.) ;
#19071=ORIENTED_EDGE('',*,*,#14830,.T.) ;
#19072=ORIENTED_EDGE('',*,*,#14831,.F.) ;
#19073=ORIENTED_EDGE('',*,*,#14806,.T.) ;
#19074=ORIENTED_EDGE('',*,*,#14832,.F.) ;
#19075=ORIENTED_EDGE('',*,*,#14833,.F.) ;
#19076=ORIENTED_EDGE('',*,*,#14834,.F.) ;
#19077=ORIENTED_EDGE('',*,*,#14784,.T.) ;
#19078=ORIENTED_EDGE('',*,*,#14835,.F.) ;
#19079=ORIENTED_EDGE('',*,*,#14836,.T.) ;
#19080=ORIENTED_EDGE('',*,*,#14837,.F.) ;
#19081=ORIENTED_EDGE('',*,*,#14802,.T.) ;
#19082=ORIENTED_EDGE('',*,*,#14838,.F.) ;
#19083=ORIENTED_EDGE('',*,*,#14839,.F.) ;
#19084=ORIENTED_EDGE('',*,*,#14840,.F.) ;
#19085=ORIENTED_EDGE('',*,*,#14780,.T.) ;
#19086=ORIENTED_EDGE('',*,*,#14841,.F.) ;
#19087=ORIENTED_EDGE('',*,*,#14842,.T.) ;
#19088=ORIENTED_EDGE('',*,*,#14843,.F.) ;
#19089=ORIENTED_EDGE('',*,*,#14798,.T.) ;
#19090=ORIENTED_EDGE('',*,*,#14844,.F.) ;
#19091=ORIENTED_EDGE('',*,*,#14845,.F.) ;
#19092=ORIENTED_EDGE('',*,*,#14846,.F.) ;
#19093=ORIENTED_EDGE('',*,*,#14776,.T.) ;
#19094=ORIENTED_EDGE('',*,*,#14847,.F.) ;
#19095=ORIENTED_EDGE('',*,*,#14848,.T.) ;
#19096=ORIENTED_EDGE('',*,*,#14849,.F.) ;
#19097=ORIENTED_EDGE('',*,*,#14772,.T.) ;
#19098=ORIENTED_EDGE('',*,*,#14850,.F.) ;
#19099=ORIENTED_EDGE('',*,*,#14851,.T.) ;
#19100=ORIENTED_EDGE('',*,*,#14852,.F.) ;
#19101=ORIENTED_EDGE('',*,*,#14825,.T.) ;
#19102=ORIENTED_EDGE('',*,*,#14853,.T.) ;
#19103=ORIENTED_EDGE('',*,*,#14854,.T.) ;
#19104=ORIENTED_EDGE('',*,*,#14855,.T.) ;
#19105=ORIENTED_EDGE('',*,*,#14856,.T.) ;
#19106=ORIENTED_EDGE('',*,*,#14857,.T.) ;
#19107=ORIENTED_EDGE('',*,*,#14858,.T.) ;
#19108=ORIENTED_EDGE('',*,*,#14859,.T.) ;
#19109=ORIENTED_EDGE('',*,*,#14860,.T.) ;
#19110=ORIENTED_EDGE('',*,*,#14861,.T.) ;
#19111=ORIENTED_EDGE('',*,*,#14862,.T.) ;
#19112=ORIENTED_EDGE('',*,*,#14863,.T.) ;
#19113=ORIENTED_EDGE('',*,*,#14864,.T.) ;
#19114=ORIENTED_EDGE('',*,*,#14865,.T.) ;
#19115=ORIENTED_EDGE('',*,*,#14866,.T.) ;
#19116=ORIENTED_EDGE('',*,*,#14867,.T.) ;
#19117=ORIENTED_EDGE('',*,*,#14868,.T.) ;
#19118=ORIENTED_EDGE('',*,*,#14869,.T.) ;
#19119=ORIENTED_EDGE('',*,*,#14870,.T.) ;
#19120=ORIENTED_EDGE('',*,*,#14871,.T.) ;
#19121=ORIENTED_EDGE('',*,*,#14872,.T.) ;
#19122=ORIENTED_EDGE('',*,*,#14873,.T.) ;
#19123=ORIENTED_EDGE('',*,*,#14874,.T.) ;
#19124=ORIENTED_EDGE('',*,*,#14875,.T.) ;
#19125=ORIENTED_EDGE('',*,*,#14876,.T.) ;
#19126=ORIENTED_EDGE('',*,*,#14877,.T.) ;
#19127=ORIENTED_EDGE('',*,*,#14878,.T.) ;
#19128=ORIENTED_EDGE('',*,*,#14879,.T.) ;
#19129=ORIENTED_EDGE('',*,*,#14880,.T.) ;
#19130=ORIENTED_EDGE('',*,*,#14881,.T.) ;
#19131=ORIENTED_EDGE('',*,*,#14882,.T.) ;
#19132=ORIENTED_EDGE('',*,*,#14883,.T.) ;
#19133=ORIENTED_EDGE('',*,*,#14884,.T.) ;
#19134=ORIENTED_EDGE('',*,*,#14885,.T.) ;
#19135=ORIENTED_EDGE('',*,*,#14886,.T.) ;
#19136=ORIENTED_EDGE('',*,*,#14887,.T.) ;
#19137=ORIENTED_EDGE('',*,*,#14888,.T.) ;
#19138=ORIENTED_EDGE('',*,*,#14889,.T.) ;
#19139=ORIENTED_EDGE('',*,*,#14890,.T.) ;
#19140=ORIENTED_EDGE('',*,*,#14891,.T.) ;
#19141=ORIENTED_EDGE('',*,*,#14892,.T.) ;
#19142=ORIENTED_EDGE('',*,*,#14893,.T.) ;
#19143=ORIENTED_EDGE('',*,*,#14894,.T.) ;
#19144=ORIENTED_EDGE('',*,*,#14895,.T.) ;
#19145=ORIENTED_EDGE('',*,*,#14896,.T.) ;
#19146=ORIENTED_EDGE('',*,*,#14897,.T.) ;
#19147=ORIENTED_EDGE('',*,*,#14898,.T.) ;
#19148=ORIENTED_EDGE('',*,*,#14899,.T.) ;
#19149=ORIENTED_EDGE('',*,*,#14900,.T.) ;
#19150=ORIENTED_EDGE('',*,*,#14901,.T.) ;
#19151=ORIENTED_EDGE('',*,*,#14902,.T.) ;
#19152=ORIENTED_EDGE('',*,*,#14903,.T.) ;
#19153=ORIENTED_EDGE('',*,*,#14904,.T.) ;
#19154=ORIENTED_EDGE('',*,*,#14905,.T.) ;
#19155=ORIENTED_EDGE('',*,*,#14906,.T.) ;
#19156=ORIENTED_EDGE('',*,*,#14907,.T.) ;
#19157=ORIENTED_EDGE('',*,*,#14908,.T.) ;
#19158=ORIENTED_EDGE('',*,*,#14909,.T.) ;
#19159=ORIENTED_EDGE('',*,*,#14910,.T.) ;
#19160=ORIENTED_EDGE('',*,*,#14911,.T.) ;
#19161=ORIENTED_EDGE('',*,*,#14912,.T.) ;
#19162=ORIENTED_EDGE('',*,*,#14913,.T.) ;
#19163=ORIENTED_EDGE('',*,*,#14914,.T.) ;
#19164=ORIENTED_EDGE('',*,*,#14915,.T.) ;
#19165=ORIENTED_EDGE('',*,*,#14916,.T.) ;
#19166=ORIENTED_EDGE('',*,*,#14917,.T.) ;
#19167=ORIENTED_EDGE('',*,*,#14918,.T.) ;
#19168=ORIENTED_EDGE('',*,*,#14816,.T.) ;
#19169=ORIENTED_EDGE('',*,*,#14795,.T.) ;
#19170=ORIENTED_EDGE('',*,*,#14919,.T.) ;
#19171=ORIENTED_EDGE('',*,*,#14920,.T.) ;
#19172=ORIENTED_EDGE('',*,*,#14921,.T.) ;
#19173=ORIENTED_EDGE('',*,*,#14922,.T.) ;
#19174=ORIENTED_EDGE('',*,*,#14923,.T.) ;
#19175=ORIENTED_EDGE('',*,*,#14924,.T.) ;
#19176=ORIENTED_EDGE('',*,*,#14925,.T.) ;
#19177=ORIENTED_EDGE('',*,*,#14926,.T.) ;
#19178=ORIENTED_EDGE('',*,*,#14927,.T.) ;
#19179=ORIENTED_EDGE('',*,*,#14928,.T.) ;
#19180=ORIENTED_EDGE('',*,*,#14929,.T.) ;
#19181=ORIENTED_EDGE('',*,*,#14930,.T.) ;
#19182=ORIENTED_EDGE('',*,*,#14931,.T.) ;
#19183=ORIENTED_EDGE('',*,*,#14932,.T.) ;
#19184=ORIENTED_EDGE('',*,*,#14933,.T.) ;
#19185=ORIENTED_EDGE('',*,*,#14934,.T.) ;
#19186=ORIENTED_EDGE('',*,*,#14820,.T.) ;
#19187=ORIENTED_EDGE('',*,*,#14793,.T.) ;
#19188=ORIENTED_EDGE('',*,*,#14818,.T.) ;
#19189=ORIENTED_EDGE('',*,*,#14828,.T.) ;
#19190=ORIENTED_EDGE('',*,*,#14935,.T.) ;
#19191=ORIENTED_EDGE('',*,*,#14811,.T.) ;
#19192=ORIENTED_EDGE('',*,*,#14834,.T.) ;
#19193=ORIENTED_EDGE('',*,*,#14936,.T.) ;
#19194=ORIENTED_EDGE('',*,*,#14937,.T.) ;
#19195=ORIENTED_EDGE('',*,*,#14807,.T.) ;
#19196=ORIENTED_EDGE('',*,*,#14840,.T.) ;
#19197=ORIENTED_EDGE('',*,*,#14938,.T.) ;
#19198=ORIENTED_EDGE('',*,*,#14939,.T.) ;
#19199=ORIENTED_EDGE('',*,*,#14803,.T.) ;
#19200=ORIENTED_EDGE('',*,*,#14846,.T.) ;
#19201=ORIENTED_EDGE('',*,*,#14940,.T.) ;
#19202=ORIENTED_EDGE('',*,*,#14799,.T.) ;
#19203=ORIENTED_EDGE('',*,*,#14785,.T.) ;
#19204=ORIENTED_EDGE('',*,*,#14837,.T.) ;
#19205=ORIENTED_EDGE('',*,*,#14941,.T.) ;
#19206=ORIENTED_EDGE('',*,*,#14942,.T.) ;
#19207=ORIENTED_EDGE('',*,*,#14781,.T.) ;
#19208=ORIENTED_EDGE('',*,*,#14843,.T.) ;
#19209=ORIENTED_EDGE('',*,*,#14943,.T.) ;
#19210=ORIENTED_EDGE('',*,*,#14944,.T.) ;
#19211=ORIENTED_EDGE('',*,*,#14777,.T.) ;
#19212=ORIENTED_EDGE('',*,*,#14849,.T.) ;
#19213=ORIENTED_EDGE('',*,*,#14945,.T.) ;
#19214=ORIENTED_EDGE('',*,*,#14946,.T.) ;
#19215=ORIENTED_EDGE('',*,*,#14773,.T.) ;
#19216=ORIENTED_EDGE('',*,*,#14852,.T.) ;
#19217=ORIENTED_EDGE('',*,*,#14947,.T.) ;
#19218=ORIENTED_EDGE('',*,*,#14948,.T.) ;
#19219=ORIENTED_EDGE('',*,*,#14789,.T.) ;
#19220=ORIENTED_EDGE('',*,*,#14831,.T.) ;
#19221=ORIENTED_EDGE('',*,*,#14949,.T.) ;
#19222=ORIENTED_EDGE('',*,*,#14950,.T.) ;
#19223=ORIENTED_EDGE('',*,*,#14951,.T.) ;
#19224=ORIENTED_EDGE('',*,*,#14952,.T.) ;
#19225=ORIENTED_EDGE('',*,*,#14953,.T.) ;
#19226=ORIENTED_EDGE('',*,*,#14954,.T.) ;
#19227=ORIENTED_EDGE('',*,*,#14955,.T.) ;
#19228=ORIENTED_EDGE('',*,*,#14956,.T.) ;
#19229=ORIENTED_EDGE('',*,*,#14957,.T.) ;
#19230=ORIENTED_EDGE('',*,*,#14958,.T.) ;
#19231=ORIENTED_EDGE('',*,*,#14959,.T.) ;
#19232=ORIENTED_EDGE('',*,*,#14960,.T.) ;
#19233=ORIENTED_EDGE('',*,*,#14961,.T.) ;
#19234=ORIENTED_EDGE('',*,*,#14962,.T.) ;
#19235=ORIENTED_EDGE('',*,*,#14963,.T.) ;
#19236=ORIENTED_EDGE('',*,*,#14964,.T.) ;
#19237=ORIENTED_EDGE('',*,*,#14965,.T.) ;
#19238=ORIENTED_EDGE('',*,*,#14966,.T.) ;
#19239=ORIENTED_EDGE('',*,*,#14967,.T.) ;
#19240=ORIENTED_EDGE('',*,*,#14968,.T.) ;
#19241=ORIENTED_EDGE('',*,*,#14969,.T.) ;
#19242=ORIENTED_EDGE('',*,*,#14970,.T.) ;
#19243=ORIENTED_EDGE('',*,*,#14971,.T.) ;
#19244=ORIENTED_EDGE('',*,*,#14972,.T.) ;
#19245=ORIENTED_EDGE('',*,*,#14973,.T.) ;
#19246=ORIENTED_EDGE('',*,*,#14974,.T.) ;
#19247=ORIENTED_EDGE('',*,*,#14975,.T.) ;
#19248=ORIENTED_EDGE('',*,*,#14976,.T.) ;
#19249=ORIENTED_EDGE('',*,*,#14977,.T.) ;
#19250=ORIENTED_EDGE('',*,*,#14978,.T.) ;
#19251=ORIENTED_EDGE('',*,*,#14979,.T.) ;
#19252=ORIENTED_EDGE('',*,*,#14980,.T.) ;
#19253=ORIENTED_EDGE('',*,*,#14981,.T.) ;
#19254=ORIENTED_EDGE('',*,*,#14982,.T.) ;
#19255=ORIENTED_EDGE('',*,*,#14983,.T.) ;
#19256=ORIENTED_EDGE('',*,*,#14984,.T.) ;
#19257=ORIENTED_EDGE('',*,*,#14985,.T.) ;
#19258=ORIENTED_EDGE('',*,*,#14986,.T.) ;
#19259=ORIENTED_EDGE('',*,*,#14987,.T.) ;
#19260=ORIENTED_EDGE('',*,*,#14988,.T.) ;
#19261=ORIENTED_EDGE('',*,*,#14989,.T.) ;
#19262=ORIENTED_EDGE('',*,*,#14990,.T.) ;
#19263=ORIENTED_EDGE('',*,*,#14991,.T.) ;
#19264=ORIENTED_EDGE('',*,*,#14992,.T.) ;
#19265=ORIENTED_EDGE('',*,*,#14993,.T.) ;
#19266=ORIENTED_EDGE('',*,*,#14994,.T.) ;
#19267=ORIENTED_EDGE('',*,*,#14995,.T.) ;
#19268=ORIENTED_EDGE('',*,*,#14996,.T.) ;
#19269=ORIENTED_EDGE('',*,*,#14997,.T.) ;
#19270=ORIENTED_EDGE('',*,*,#14998,.T.) ;
#19271=ORIENTED_EDGE('',*,*,#14999,.T.) ;
#19272=ORIENTED_EDGE('',*,*,#15000,.T.) ;
#19273=ORIENTED_EDGE('',*,*,#15001,.T.) ;
#19274=ORIENTED_EDGE('',*,*,#15002,.T.) ;
#19275=ORIENTED_EDGE('',*,*,#15003,.T.) ;
#19276=ORIENTED_EDGE('',*,*,#15004,.T.) ;
#19277=ORIENTED_EDGE('',*,*,#15005,.T.) ;
#19278=ORIENTED_EDGE('',*,*,#15006,.T.) ;
#19279=ORIENTED_EDGE('',*,*,#15007,.T.) ;
#19280=ORIENTED_EDGE('',*,*,#15008,.T.) ;
#19281=ORIENTED_EDGE('',*,*,#15009,.T.) ;
#19282=ORIENTED_EDGE('',*,*,#15010,.T.) ;
#19283=ORIENTED_EDGE('',*,*,#15011,.T.) ;
#19284=ORIENTED_EDGE('',*,*,#15012,.T.) ;
#19285=ORIENTED_EDGE('',*,*,#15013,.T.) ;
#19286=ORIENTED_EDGE('',*,*,#15014,.T.) ;
#19287=ORIENTED_EDGE('',*,*,#15015,.T.) ;
#19288=ORIENTED_EDGE('',*,*,#15016,.T.) ;
#19289=ORIENTED_EDGE('',*,*,#15017,.T.) ;
#19290=ORIENTED_EDGE('',*,*,#15018,.T.) ;
#19291=ORIENTED_EDGE('',*,*,#15019,.T.) ;
#19292=ORIENTED_EDGE('',*,*,#15020,.T.) ;
#19293=ORIENTED_EDGE('',*,*,#15021,.T.) ;
#19294=ORIENTED_EDGE('',*,*,#15022,.T.) ;
#19295=ORIENTED_EDGE('',*,*,#15023,.T.) ;
#19296=ORIENTED_EDGE('',*,*,#15024,.T.) ;
#19297=ORIENTED_EDGE('',*,*,#15025,.T.) ;
#19298=ORIENTED_EDGE('',*,*,#15026,.T.) ;
#19299=ORIENTED_EDGE('',*,*,#15027,.T.) ;
#19300=ORIENTED_EDGE('',*,*,#15028,.T.) ;
#19301=ORIENTED_EDGE('',*,*,#15029,.T.) ;
#19302=ORIENTED_EDGE('',*,*,#15030,.T.) ;
#19303=ORIENTED_EDGE('',*,*,#15031,.T.) ;
#19304=ORIENTED_EDGE('',*,*,#15032,.T.) ;
#19305=ORIENTED_EDGE('',*,*,#15033,.T.) ;
#19306=ORIENTED_EDGE('',*,*,#15034,.T.) ;
#19307=ORIENTED_EDGE('',*,*,#15035,.T.) ;
#19308=ORIENTED_EDGE('',*,*,#15036,.T.) ;
#19309=ORIENTED_EDGE('',*,*,#15037,.T.) ;
#19310=ORIENTED_EDGE('',*,*,#15038,.T.) ;
#19311=ORIENTED_EDGE('',*,*,#15039,.T.) ;
#19312=ORIENTED_EDGE('',*,*,#15040,.T.) ;
#19313=ORIENTED_EDGE('',*,*,#15041,.T.) ;
#19314=ORIENTED_EDGE('',*,*,#15042,.T.) ;
#19315=ORIENTED_EDGE('',*,*,#15043,.T.) ;
#19316=ORIENTED_EDGE('',*,*,#15044,.T.) ;
#19317=ORIENTED_EDGE('',*,*,#15045,.T.) ;
#19318=ORIENTED_EDGE('',*,*,#15046,.T.) ;
#19319=ORIENTED_EDGE('',*,*,#15047,.T.) ;
#19320=ORIENTED_EDGE('',*,*,#15048,.T.) ;
#19321=ORIENTED_EDGE('',*,*,#15049,.T.) ;
#19322=ORIENTED_EDGE('',*,*,#15050,.T.) ;
#19323=ORIENTED_EDGE('',*,*,#15051,.T.) ;
#19324=ORIENTED_EDGE('',*,*,#15052,.T.) ;
#19325=ORIENTED_EDGE('',*,*,#15053,.T.) ;
#19326=ORIENTED_EDGE('',*,*,#15054,.T.) ;
#19327=ORIENTED_EDGE('',*,*,#15055,.T.) ;
#19328=ORIENTED_EDGE('',*,*,#15056,.T.) ;
#19329=ORIENTED_EDGE('',*,*,#15057,.T.) ;
#19330=ORIENTED_EDGE('',*,*,#15058,.T.) ;
#19331=ORIENTED_EDGE('',*,*,#15059,.T.) ;
#19332=ORIENTED_EDGE('',*,*,#15060,.T.) ;
#19333=ORIENTED_EDGE('',*,*,#15061,.T.) ;
#19334=ORIENTED_EDGE('',*,*,#15062,.T.) ;
#19335=ORIENTED_EDGE('',*,*,#15063,.T.) ;
#19336=ORIENTED_EDGE('',*,*,#15064,.T.) ;
#19337=ORIENTED_EDGE('',*,*,#15065,.T.) ;
#19338=ORIENTED_EDGE('',*,*,#15066,.T.) ;
#19339=ORIENTED_EDGE('',*,*,#15067,.T.) ;
#19340=ORIENTED_EDGE('',*,*,#15068,.T.) ;
#19341=ORIENTED_EDGE('',*,*,#15069,.T.) ;
#19342=ORIENTED_EDGE('',*,*,#15070,.T.) ;
#19343=ORIENTED_EDGE('',*,*,#15071,.T.) ;
#19344=ORIENTED_EDGE('',*,*,#15072,.T.) ;
#19345=ORIENTED_EDGE('',*,*,#15073,.T.) ;
#19346=ORIENTED_EDGE('',*,*,#15074,.T.) ;
#19347=ORIENTED_EDGE('',*,*,#15075,.T.) ;
#19348=ORIENTED_EDGE('',*,*,#15076,.T.) ;
#19349=ORIENTED_EDGE('',*,*,#15077,.T.) ;
#19350=ORIENTED_EDGE('',*,*,#15078,.T.) ;
#19351=ORIENTED_EDGE('',*,*,#15079,.T.) ;
#19352=ORIENTED_EDGE('',*,*,#15080,.T.) ;
#19353=ORIENTED_EDGE('',*,*,#15081,.T.) ;
#19354=ORIENTED_EDGE('',*,*,#15082,.T.) ;
#19355=ORIENTED_EDGE('',*,*,#15083,.T.) ;
#19356=ORIENTED_EDGE('',*,*,#15084,.T.) ;
#19357=ORIENTED_EDGE('',*,*,#15085,.T.) ;
#19358=ORIENTED_EDGE('',*,*,#15086,.T.) ;
#19359=ORIENTED_EDGE('',*,*,#15087,.T.) ;
#19360=ORIENTED_EDGE('',*,*,#15088,.T.) ;
#19361=ORIENTED_EDGE('',*,*,#15089,.T.) ;
#19362=ORIENTED_EDGE('',*,*,#15090,.T.) ;
#19363=ORIENTED_EDGE('',*,*,#15091,.T.) ;
#19364=ORIENTED_EDGE('',*,*,#15092,.T.) ;
#19365=ORIENTED_EDGE('',*,*,#15093,.T.) ;
#19366=ORIENTED_EDGE('',*,*,#15094,.T.) ;
#19367=ORIENTED_EDGE('',*,*,#15095,.T.) ;
#19368=ORIENTED_EDGE('',*,*,#15096,.T.) ;
#19369=ORIENTED_EDGE('',*,*,#15097,.T.) ;
#19370=ORIENTED_EDGE('',*,*,#15098,.T.) ;
#19371=ORIENTED_EDGE('',*,*,#15099,.T.) ;
#19372=ORIENTED_EDGE('',*,*,#15100,.T.) ;
#19373=ORIENTED_EDGE('',*,*,#15101,.T.) ;
#19374=ORIENTED_EDGE('',*,*,#15102,.T.) ;
#19375=ORIENTED_EDGE('',*,*,#15103,.T.) ;
#19376=ORIENTED_EDGE('',*,*,#15104,.T.) ;
#19377=ORIENTED_EDGE('',*,*,#15105,.T.) ;
#19378=ORIENTED_EDGE('',*,*,#15106,.T.) ;
#19379=ORIENTED_EDGE('',*,*,#15107,.T.) ;
#19380=ORIENTED_EDGE('',*,*,#15108,.T.) ;
#19381=ORIENTED_EDGE('',*,*,#15109,.T.) ;
#19382=ORIENTED_EDGE('',*,*,#15110,.T.) ;
#19383=ORIENTED_EDGE('',*,*,#15111,.T.) ;
#19384=ORIENTED_EDGE('',*,*,#15112,.T.) ;
#19385=ORIENTED_EDGE('',*,*,#15113,.T.) ;
#19386=ORIENTED_EDGE('',*,*,#15114,.T.) ;
#19387=ORIENTED_EDGE('',*,*,#15115,.T.) ;
#19388=ORIENTED_EDGE('',*,*,#14769,.T.) ;
#19389=ORIENTED_EDGE('',*,*,#15116,.T.) ;
#19390=ORIENTED_EDGE('',*,*,#15117,.T.) ;
#19391=ORIENTED_EDGE('',*,*,#15118,.T.) ;
#19392=ORIENTED_EDGE('',*,*,#15119,.T.) ;
#19393=ORIENTED_EDGE('',*,*,#14768,.T.) ;
#19394=ORIENTED_EDGE('',*,*,#15120,.F.) ;
#19395=ORIENTED_EDGE('',*,*,#15121,.T.) ;
#19396=ORIENTED_EDGE('',*,*,#15116,.F.) ;
#19397=ORIENTED_EDGE('',*,*,#14822,.T.) ;
#19398=ORIENTED_EDGE('',*,*,#15122,.T.) ;
#19399=ORIENTED_EDGE('',*,*,#15123,.T.) ;
#19400=ORIENTED_EDGE('',*,*,#15124,.T.) ;
#19401=ORIENTED_EDGE('',*,*,#15125,.T.) ;
#19402=ORIENTED_EDGE('',*,*,#15126,.T.) ;
#19403=ORIENTED_EDGE('',*,*,#15127,.T.) ;
#19404=ORIENTED_EDGE('',*,*,#15128,.T.) ;
#19405=ORIENTED_EDGE('',*,*,#15129,.T.) ;
#19406=ORIENTED_EDGE('',*,*,#15130,.T.) ;
#19407=ORIENTED_EDGE('',*,*,#15131,.T.) ;
#19408=ORIENTED_EDGE('',*,*,#15132,.T.) ;
#19409=ORIENTED_EDGE('',*,*,#15133,.T.) ;
#19410=ORIENTED_EDGE('',*,*,#15134,.T.) ;
#19411=ORIENTED_EDGE('',*,*,#15135,.T.) ;
#19412=ORIENTED_EDGE('',*,*,#15136,.T.) ;
#19413=ORIENTED_EDGE('',*,*,#15137,.T.) ;
#19414=ORIENTED_EDGE('',*,*,#14797,.T.) ;
#19415=ORIENTED_EDGE('',*,*,#14815,.T.) ;
#19416=ORIENTED_EDGE('',*,*,#15138,.T.) ;
#19417=ORIENTED_EDGE('',*,*,#15139,.T.) ;
#19418=ORIENTED_EDGE('',*,*,#15140,.T.) ;
#19419=ORIENTED_EDGE('',*,*,#15141,.T.) ;
#19420=ORIENTED_EDGE('',*,*,#15142,.T.) ;
#19421=ORIENTED_EDGE('',*,*,#15143,.T.) ;
#19422=ORIENTED_EDGE('',*,*,#15144,.T.) ;
#19423=ORIENTED_EDGE('',*,*,#15145,.T.) ;
#19424=ORIENTED_EDGE('',*,*,#15146,.T.) ;
#19425=ORIENTED_EDGE('',*,*,#15147,.T.) ;
#19426=ORIENTED_EDGE('',*,*,#15148,.T.) ;
#19427=ORIENTED_EDGE('',*,*,#15149,.T.) ;
#19428=ORIENTED_EDGE('',*,*,#15150,.T.) ;
#19429=ORIENTED_EDGE('',*,*,#15151,.T.) ;
#19430=ORIENTED_EDGE('',*,*,#15152,.T.) ;
#19431=ORIENTED_EDGE('',*,*,#15153,.T.) ;
#19432=ORIENTED_EDGE('',*,*,#15154,.T.) ;
#19433=ORIENTED_EDGE('',*,*,#15155,.T.) ;
#19434=ORIENTED_EDGE('',*,*,#15156,.T.) ;
#19435=ORIENTED_EDGE('',*,*,#15157,.T.) ;
#19436=ORIENTED_EDGE('',*,*,#15158,.T.) ;
#19437=ORIENTED_EDGE('',*,*,#15159,.T.) ;
#19438=ORIENTED_EDGE('',*,*,#15160,.T.) ;
#19439=ORIENTED_EDGE('',*,*,#15161,.T.) ;
#19440=ORIENTED_EDGE('',*,*,#15162,.T.) ;
#19441=ORIENTED_EDGE('',*,*,#15163,.T.) ;
#19442=ORIENTED_EDGE('',*,*,#15164,.T.) ;
#19443=ORIENTED_EDGE('',*,*,#15165,.T.) ;
#19444=ORIENTED_EDGE('',*,*,#15166,.T.) ;
#19445=ORIENTED_EDGE('',*,*,#15167,.T.) ;
#19446=ORIENTED_EDGE('',*,*,#15168,.T.) ;
#19447=ORIENTED_EDGE('',*,*,#15169,.T.) ;
#19448=ORIENTED_EDGE('',*,*,#15170,.T.) ;
#19449=ORIENTED_EDGE('',*,*,#15171,.T.) ;
#19450=ORIENTED_EDGE('',*,*,#15172,.T.) ;
#19451=ORIENTED_EDGE('',*,*,#15173,.T.) ;
#19452=ORIENTED_EDGE('',*,*,#15174,.T.) ;
#19453=ORIENTED_EDGE('',*,*,#15175,.T.) ;
#19454=ORIENTED_EDGE('',*,*,#15176,.T.) ;
#19455=ORIENTED_EDGE('',*,*,#15177,.T.) ;
#19456=ORIENTED_EDGE('',*,*,#15178,.T.) ;
#19457=ORIENTED_EDGE('',*,*,#15179,.T.) ;
#19458=ORIENTED_EDGE('',*,*,#15180,.T.) ;
#19459=ORIENTED_EDGE('',*,*,#15181,.T.) ;
#19460=ORIENTED_EDGE('',*,*,#15182,.T.) ;
#19461=ORIENTED_EDGE('',*,*,#15183,.T.) ;
#19462=ORIENTED_EDGE('',*,*,#15184,.T.) ;
#19463=ORIENTED_EDGE('',*,*,#15185,.T.) ;
#19464=ORIENTED_EDGE('',*,*,#15186,.T.) ;
#19465=ORIENTED_EDGE('',*,*,#15187,.T.) ;
#19466=ORIENTED_EDGE('',*,*,#15188,.T.) ;
#19467=ORIENTED_EDGE('',*,*,#15189,.T.) ;
#19468=ORIENTED_EDGE('',*,*,#15190,.T.) ;
#19469=ORIENTED_EDGE('',*,*,#15191,.T.) ;
#19470=ORIENTED_EDGE('',*,*,#15192,.T.) ;
#19471=ORIENTED_EDGE('',*,*,#15193,.T.) ;
#19472=ORIENTED_EDGE('',*,*,#15194,.T.) ;
#19473=ORIENTED_EDGE('',*,*,#15195,.T.) ;
#19474=ORIENTED_EDGE('',*,*,#15196,.T.) ;
#19475=ORIENTED_EDGE('',*,*,#15197,.T.) ;
#19476=ORIENTED_EDGE('',*,*,#15198,.T.) ;
#19477=ORIENTED_EDGE('',*,*,#15199,.T.) ;
#19478=ORIENTED_EDGE('',*,*,#15200,.T.) ;
#19479=ORIENTED_EDGE('',*,*,#15201,.T.) ;
#19480=ORIENTED_EDGE('',*,*,#15202,.T.) ;
#19481=ORIENTED_EDGE('',*,*,#15203,.T.) ;
#19482=ORIENTED_EDGE('',*,*,#14823,.T.) ;
#19483=ORIENTED_EDGE('',*,*,#14819,.T.) ;
#19484=ORIENTED_EDGE('',*,*,#14791,.T.) ;
#19485=ORIENTED_EDGE('',*,*,#15204,.T.) ;
#19486=ORIENTED_EDGE('',*,*,#15205,.T.) ;
#19487=ORIENTED_EDGE('',*,*,#14835,.T.) ;
#19488=ORIENTED_EDGE('',*,*,#14783,.T.) ;
#19489=ORIENTED_EDGE('',*,*,#15206,.T.) ;
#19490=ORIENTED_EDGE('',*,*,#15207,.T.) ;
#19491=ORIENTED_EDGE('',*,*,#14841,.T.) ;
#19492=ORIENTED_EDGE('',*,*,#14779,.T.) ;
#19493=ORIENTED_EDGE('',*,*,#15208,.T.) ;
#19494=ORIENTED_EDGE('',*,*,#15209,.T.) ;
#19495=ORIENTED_EDGE('',*,*,#14847,.T.) ;
#19496=ORIENTED_EDGE('',*,*,#14775,.T.) ;
#19497=ORIENTED_EDGE('',*,*,#15210,.T.) ;
#19498=ORIENTED_EDGE('',*,*,#15211,.T.) ;
#19499=ORIENTED_EDGE('',*,*,#14850,.T.) ;
#19500=ORIENTED_EDGE('',*,*,#14771,.T.) ;
#19501=ORIENTED_EDGE('',*,*,#15212,.T.) ;
#19502=ORIENTED_EDGE('',*,*,#15213,.T.) ;
#19503=ORIENTED_EDGE('',*,*,#15214,.T.) ;
#19504=ORIENTED_EDGE('',*,*,#14829,.T.) ;
#19505=ORIENTED_EDGE('',*,*,#14787,.T.) ;
#19506=ORIENTED_EDGE('',*,*,#14809,.T.) ;
#19507=ORIENTED_EDGE('',*,*,#15215,.T.) ;
#19508=ORIENTED_EDGE('',*,*,#15216,.T.) ;
#19509=ORIENTED_EDGE('',*,*,#14832,.T.) ;
#19510=ORIENTED_EDGE('',*,*,#14805,.T.) ;
#19511=ORIENTED_EDGE('',*,*,#15217,.T.) ;
#19512=ORIENTED_EDGE('',*,*,#15218,.T.) ;
#19513=ORIENTED_EDGE('',*,*,#14838,.T.) ;
#19514=ORIENTED_EDGE('',*,*,#14801,.T.) ;
#19515=ORIENTED_EDGE('',*,*,#15219,.T.) ;
#19516=ORIENTED_EDGE('',*,*,#14844,.T.) ;
#19517=ORIENTED_EDGE('',*,*,#15220,.T.) ;
#19518=ORIENTED_EDGE('',*,*,#15221,.T.) ;
#19519=ORIENTED_EDGE('',*,*,#15222,.T.) ;
#19520=ORIENTED_EDGE('',*,*,#15120,.T.) ;
#19521=ORIENTED_EDGE('',*,*,#14767,.T.) ;
#19522=ORIENTED_EDGE('',*,*,#14813,.T.) ;
#19523=ORIENTED_EDGE('',*,*,#15223,.T.) ;
#19524=ORIENTED_EDGE('',*,*,#14826,.T.) ;
#19525=ORIENTED_EDGE('',*,*,#15224,.T.) ;
#19526=ORIENTED_EDGE('',*,*,#15225,.T.) ;
#19527=ORIENTED_EDGE('',*,*,#15226,.T.) ;
#19528=ORIENTED_EDGE('',*,*,#15227,.T.) ;
#19529=ORIENTED_EDGE('',*,*,#15228,.T.) ;
#19530=ORIENTED_EDGE('',*,*,#15229,.T.) ;
#19531=ORIENTED_EDGE('',*,*,#15230,.T.) ;
#19532=ORIENTED_EDGE('',*,*,#15231,.T.) ;
#19533=ORIENTED_EDGE('',*,*,#15232,.T.) ;
#19534=ORIENTED_EDGE('',*,*,#15233,.T.) ;
#19535=ORIENTED_EDGE('',*,*,#15234,.T.) ;
#19536=ORIENTED_EDGE('',*,*,#15235,.T.) ;
#19537=ORIENTED_EDGE('',*,*,#15236,.T.) ;
#19538=ORIENTED_EDGE('',*,*,#15237,.T.) ;
#19539=ORIENTED_EDGE('',*,*,#15238,.T.) ;
#19540=ORIENTED_EDGE('',*,*,#15239,.T.) ;
#19541=ORIENTED_EDGE('',*,*,#15240,.T.) ;
#19542=ORIENTED_EDGE('',*,*,#15241,.T.) ;
#19543=ORIENTED_EDGE('',*,*,#15242,.T.) ;
#19544=ORIENTED_EDGE('',*,*,#15243,.T.) ;
#19545=ORIENTED_EDGE('',*,*,#15244,.T.) ;
#19546=ORIENTED_EDGE('',*,*,#15245,.T.) ;
#19547=ORIENTED_EDGE('',*,*,#15246,.T.) ;
#19548=ORIENTED_EDGE('',*,*,#15247,.T.) ;
#19549=ORIENTED_EDGE('',*,*,#15248,.T.) ;
#19550=ORIENTED_EDGE('',*,*,#15249,.T.) ;
#19551=ORIENTED_EDGE('',*,*,#15250,.T.) ;
#19552=ORIENTED_EDGE('',*,*,#15251,.T.) ;
#19553=ORIENTED_EDGE('',*,*,#15252,.T.) ;
#19554=ORIENTED_EDGE('',*,*,#15253,.T.) ;
#19555=ORIENTED_EDGE('',*,*,#15254,.T.) ;
#19556=ORIENTED_EDGE('',*,*,#15255,.T.) ;
#19557=ORIENTED_EDGE('',*,*,#15256,.T.) ;
#19558=ORIENTED_EDGE('',*,*,#15257,.T.) ;
#19559=ORIENTED_EDGE('',*,*,#15258,.T.) ;
#19560=ORIENTED_EDGE('',*,*,#15259,.T.) ;
#19561=ORIENTED_EDGE('',*,*,#15260,.T.) ;
#19562=ORIENTED_EDGE('',*,*,#15261,.T.) ;
#19563=ORIENTED_EDGE('',*,*,#15262,.T.) ;
#19564=ORIENTED_EDGE('',*,*,#15263,.T.) ;
#19565=ORIENTED_EDGE('',*,*,#15264,.T.) ;
#19566=ORIENTED_EDGE('',*,*,#15265,.T.) ;
#19567=ORIENTED_EDGE('',*,*,#15266,.T.) ;
#19568=ORIENTED_EDGE('',*,*,#15267,.T.) ;
#19569=ORIENTED_EDGE('',*,*,#15268,.T.) ;
#19570=ORIENTED_EDGE('',*,*,#15269,.T.) ;
#19571=ORIENTED_EDGE('',*,*,#15270,.T.) ;
#19572=ORIENTED_EDGE('',*,*,#15271,.T.) ;
#19573=ORIENTED_EDGE('',*,*,#15272,.T.) ;
#19574=ORIENTED_EDGE('',*,*,#15273,.T.) ;
#19575=ORIENTED_EDGE('',*,*,#15274,.T.) ;
#19576=ORIENTED_EDGE('',*,*,#15275,.T.) ;
#19577=ORIENTED_EDGE('',*,*,#15276,.T.) ;
#19578=ORIENTED_EDGE('',*,*,#15277,.T.) ;
#19579=ORIENTED_EDGE('',*,*,#15278,.T.) ;
#19580=ORIENTED_EDGE('',*,*,#15279,.T.) ;
#19581=ORIENTED_EDGE('',*,*,#15280,.T.) ;
#19582=ORIENTED_EDGE('',*,*,#15281,.T.) ;
#19583=ORIENTED_EDGE('',*,*,#15282,.T.) ;
#19584=ORIENTED_EDGE('',*,*,#15283,.T.) ;
#19585=ORIENTED_EDGE('',*,*,#15284,.T.) ;
#19586=ORIENTED_EDGE('',*,*,#15285,.T.) ;
#19587=ORIENTED_EDGE('',*,*,#15286,.T.) ;
#19588=ORIENTED_EDGE('',*,*,#15287,.T.) ;
#19589=ORIENTED_EDGE('',*,*,#15288,.T.) ;
#19590=ORIENTED_EDGE('',*,*,#15289,.T.) ;
#19591=ORIENTED_EDGE('',*,*,#15290,.T.) ;
#19592=ORIENTED_EDGE('',*,*,#15291,.T.) ;
#19593=ORIENTED_EDGE('',*,*,#15292,.T.) ;
#19594=ORIENTED_EDGE('',*,*,#15293,.T.) ;
#19595=ORIENTED_EDGE('',*,*,#15294,.T.) ;
#19596=ORIENTED_EDGE('',*,*,#15295,.T.) ;
#19597=ORIENTED_EDGE('',*,*,#15296,.T.) ;
#19598=ORIENTED_EDGE('',*,*,#15297,.T.) ;
#19599=ORIENTED_EDGE('',*,*,#15298,.T.) ;
#19600=ORIENTED_EDGE('',*,*,#15299,.T.) ;
#19601=ORIENTED_EDGE('',*,*,#15300,.T.) ;
#19602=ORIENTED_EDGE('',*,*,#15301,.T.) ;
#19603=ORIENTED_EDGE('',*,*,#15302,.T.) ;
#19604=ORIENTED_EDGE('',*,*,#15303,.T.) ;
#19605=ORIENTED_EDGE('',*,*,#15304,.T.) ;
#19606=ORIENTED_EDGE('',*,*,#15305,.T.) ;
#19607=ORIENTED_EDGE('',*,*,#15306,.T.) ;
#19608=ORIENTED_EDGE('',*,*,#15307,.T.) ;
#19609=ORIENTED_EDGE('',*,*,#15308,.T.) ;
#19610=ORIENTED_EDGE('',*,*,#15309,.T.) ;
#19611=ORIENTED_EDGE('',*,*,#15310,.T.) ;
#19612=ORIENTED_EDGE('',*,*,#15311,.T.) ;
#19613=ORIENTED_EDGE('',*,*,#15312,.T.) ;
#19614=ORIENTED_EDGE('',*,*,#15313,.T.) ;
#19615=ORIENTED_EDGE('',*,*,#15314,.T.) ;
#19616=ORIENTED_EDGE('',*,*,#15315,.T.) ;
#19617=ORIENTED_EDGE('',*,*,#15316,.T.) ;
#19618=ORIENTED_EDGE('',*,*,#15317,.T.) ;
#19619=ORIENTED_EDGE('',*,*,#15318,.T.) ;
#19620=ORIENTED_EDGE('',*,*,#15319,.T.) ;
#19621=ORIENTED_EDGE('',*,*,#15320,.T.) ;
#19622=ORIENTED_EDGE('',*,*,#15321,.T.) ;
#19623=ORIENTED_EDGE('',*,*,#15322,.T.) ;
#19624=ORIENTED_EDGE('',*,*,#15323,.T.) ;
#19625=ORIENTED_EDGE('',*,*,#15324,.T.) ;
#19626=ORIENTED_EDGE('',*,*,#15325,.T.) ;
#19627=ORIENTED_EDGE('',*,*,#15326,.T.) ;
#19628=ORIENTED_EDGE('',*,*,#15327,.T.) ;
#19629=ORIENTED_EDGE('',*,*,#15328,.T.) ;
#19630=ORIENTED_EDGE('',*,*,#15329,.T.) ;
#19631=ORIENTED_EDGE('',*,*,#15330,.T.) ;
#19632=ORIENTED_EDGE('',*,*,#15331,.T.) ;
#19633=ORIENTED_EDGE('',*,*,#15332,.T.) ;
#19634=ORIENTED_EDGE('',*,*,#15333,.T.) ;
#19635=ORIENTED_EDGE('',*,*,#15334,.T.) ;
#19636=ORIENTED_EDGE('',*,*,#15335,.T.) ;
#19637=ORIENTED_EDGE('',*,*,#15336,.T.) ;
#19638=ORIENTED_EDGE('',*,*,#15337,.T.) ;
#19639=ORIENTED_EDGE('',*,*,#15338,.T.) ;
#19640=ORIENTED_EDGE('',*,*,#15339,.T.) ;
#19641=ORIENTED_EDGE('',*,*,#15340,.T.) ;
#19642=ORIENTED_EDGE('',*,*,#15341,.T.) ;
#19643=ORIENTED_EDGE('',*,*,#15342,.T.) ;
#19644=ORIENTED_EDGE('',*,*,#15343,.T.) ;
#19645=ORIENTED_EDGE('',*,*,#15344,.T.) ;
#19646=ORIENTED_EDGE('',*,*,#15345,.T.) ;
#19647=ORIENTED_EDGE('',*,*,#15346,.T.) ;
#19648=ORIENTED_EDGE('',*,*,#15347,.T.) ;
#19649=ORIENTED_EDGE('',*,*,#15348,.T.) ;
#19650=ORIENTED_EDGE('',*,*,#15349,.T.) ;
#19651=ORIENTED_EDGE('',*,*,#15350,.T.) ;
#19652=ORIENTED_EDGE('',*,*,#15351,.T.) ;
#19653=ORIENTED_EDGE('',*,*,#15352,.T.) ;
#19654=ORIENTED_EDGE('',*,*,#15353,.T.) ;
#19655=ORIENTED_EDGE('',*,*,#15354,.T.) ;
#19656=ORIENTED_EDGE('',*,*,#15355,.T.) ;
#19657=ORIENTED_EDGE('',*,*,#15356,.T.) ;
#19658=ORIENTED_EDGE('',*,*,#15357,.T.) ;
#19659=ORIENTED_EDGE('',*,*,#15358,.T.) ;
#19660=ORIENTED_EDGE('',*,*,#15359,.T.) ;
#19661=ORIENTED_EDGE('',*,*,#15360,.T.) ;
#19662=ORIENTED_EDGE('',*,*,#15361,.T.) ;
#19663=ORIENTED_EDGE('',*,*,#15362,.T.) ;
#19664=ORIENTED_EDGE('',*,*,#15363,.T.) ;
#19665=ORIENTED_EDGE('',*,*,#15364,.T.) ;
#19666=ORIENTED_EDGE('',*,*,#15365,.T.) ;
#19667=ORIENTED_EDGE('',*,*,#15366,.T.) ;
#19668=ORIENTED_EDGE('',*,*,#15367,.T.) ;
#19669=ORIENTED_EDGE('',*,*,#15368,.T.) ;
#19670=ORIENTED_EDGE('',*,*,#15369,.T.) ;
#19671=ORIENTED_EDGE('',*,*,#15370,.T.) ;
#19672=ORIENTED_EDGE('',*,*,#15371,.T.) ;
#19673=ORIENTED_EDGE('',*,*,#15372,.T.) ;
#19674=ORIENTED_EDGE('',*,*,#15373,.T.) ;
#19675=ORIENTED_EDGE('',*,*,#15374,.T.) ;
#19676=ORIENTED_EDGE('',*,*,#15375,.T.) ;
#19677=ORIENTED_EDGE('',*,*,#15376,.T.) ;
#19678=ORIENTED_EDGE('',*,*,#15377,.T.) ;
#19679=ORIENTED_EDGE('',*,*,#15378,.T.) ;
#19680=ORIENTED_EDGE('',*,*,#15379,.T.) ;
#19681=ORIENTED_EDGE('',*,*,#15380,.T.) ;
#19682=ORIENTED_EDGE('',*,*,#15381,.T.) ;
#19683=ORIENTED_EDGE('',*,*,#15382,.T.) ;
#19684=ORIENTED_EDGE('',*,*,#15383,.T.) ;
#19685=ORIENTED_EDGE('',*,*,#15384,.T.) ;
#19686=ORIENTED_EDGE('',*,*,#15385,.T.) ;
#19687=ORIENTED_EDGE('',*,*,#15386,.T.) ;
#19688=ORIENTED_EDGE('',*,*,#15387,.T.) ;
#19689=ORIENTED_EDGE('',*,*,#14814,.T.) ;
#19690=ORIENTED_EDGE('',*,*,#14918,.F.) ;
#19691=ORIENTED_EDGE('',*,*,#15388,.T.) ;
#19692=ORIENTED_EDGE('',*,*,#15138,.F.) ;
#19693=ORIENTED_EDGE('',*,*,#14794,.T.) ;
#19694=ORIENTED_EDGE('',*,*,#15137,.F.) ;
#19695=ORIENTED_EDGE('',*,*,#15389,.T.) ;
#19696=ORIENTED_EDGE('',*,*,#14919,.F.) ;
#19697=ORIENTED_EDGE('',*,*,#14824,.F.) ;
#19698=ORIENTED_EDGE('',*,*,#15203,.F.) ;
#19699=ORIENTED_EDGE('',*,*,#15390,.F.) ;
#19700=ORIENTED_EDGE('',*,*,#14853,.F.) ;
#19701=ORIENTED_EDGE('',*,*,#15391,.F.) ;
#19702=ORIENTED_EDGE('',*,*,#14983,.F.) ;
#19703=ORIENTED_EDGE('',*,*,#15392,.F.) ;
#19704=ORIENTED_EDGE('',*,*,#15224,.F.) ;
#19705=ORIENTED_EDGE('',*,*,#15393,.F.) ;
#19706=ORIENTED_EDGE('',*,*,#14966,.F.) ;
#19707=ORIENTED_EDGE('',*,*,#15394,.F.) ;
#19708=ORIENTED_EDGE('',*,*,#15358,.F.) ;
#19709=ORIENTED_EDGE('',*,*,#15395,.F.) ;
#19710=ORIENTED_EDGE('',*,*,#14962,.F.) ;
#19711=ORIENTED_EDGE('',*,*,#15396,.F.) ;
#19712=ORIENTED_EDGE('',*,*,#15362,.F.) ;
#19713=ORIENTED_EDGE('',*,*,#15397,.F.) ;
#19714=ORIENTED_EDGE('',*,*,#15213,.F.) ;
#19715=ORIENTED_EDGE('',*,*,#15398,.F.) ;
#19716=ORIENTED_EDGE('',*,*,#14950,.F.) ;
#19717=ORIENTED_EDGE('',*,*,#15399,.F.) ;
#19718=ORIENTED_EDGE('',*,*,#15387,.F.) ;
#19719=ORIENTED_EDGE('',*,*,#15400,.F.) ;
#19720=ORIENTED_EDGE('',*,*,#14967,.F.) ;
#19721=ORIENTED_EDGE('',*,*,#15401,.F.) ;
#19722=ORIENTED_EDGE('',*,*,#14958,.F.) ;
#19723=ORIENTED_EDGE('',*,*,#15402,.F.) ;
#19724=ORIENTED_EDGE('',*,*,#15366,.F.) ;
#19725=ORIENTED_EDGE('',*,*,#15403,.F.) ;
#19726=ORIENTED_EDGE('',*,*,#15184,.F.) ;
#19727=ORIENTED_EDGE('',*,*,#15404,.F.) ;
#19728=ORIENTED_EDGE('',*,*,#14872,.F.) ;
#19729=ORIENTED_EDGE('',*,*,#15405,.F.) ;
#19730=ORIENTED_EDGE('',*,*,#15375,.F.) ;
#19731=ORIENTED_EDGE('',*,*,#15406,.F.) ;
#19732=ORIENTED_EDGE('',*,*,#14984,.F.) ;
#19733=ORIENTED_EDGE('',*,*,#15407,.F.) ;
#19734=ORIENTED_EDGE('',*,*,#15379,.F.) ;
#19735=ORIENTED_EDGE('',*,*,#15408,.F.) ;
#19736=ORIENTED_EDGE('',*,*,#14975,.F.) ;
#19737=ORIENTED_EDGE('',*,*,#15409,.F.) ;
#19738=ORIENTED_EDGE('',*,*,#15383,.F.) ;
#19739=ORIENTED_EDGE('',*,*,#15410,.F.) ;
#19740=ORIENTED_EDGE('',*,*,#14971,.F.) ;
#19741=ORIENTED_EDGE('',*,*,#15411,.F.) ;
#19742=ORIENTED_EDGE('',*,*,#14854,.F.) ;
#19743=ORIENTED_EDGE('',*,*,#15390,.T.) ;
#19744=ORIENTED_EDGE('',*,*,#15202,.F.) ;
#19745=ORIENTED_EDGE('',*,*,#15412,.F.) ;
#19746=ORIENTED_EDGE('',*,*,#14873,.F.) ;
#19747=ORIENTED_EDGE('',*,*,#15404,.T.) ;
#19748=ORIENTED_EDGE('',*,*,#15183,.F.) ;
#19749=ORIENTED_EDGE('',*,*,#15413,.F.) ;
#19750=ORIENTED_EDGE('',*,*,#14954,.F.) ;
#19751=ORIENTED_EDGE('',*,*,#15414,.F.) ;
#19752=ORIENTED_EDGE('',*,*,#15370,.F.) ;
#19753=ORIENTED_EDGE('',*,*,#15413,.T.) ;
#19754=ORIENTED_EDGE('',*,*,#15372,.F.) ;
#19755=ORIENTED_EDGE('',*,*,#15415,.F.) ;
#19756=ORIENTED_EDGE('',*,*,#14952,.F.) ;
#19757=ORIENTED_EDGE('',*,*,#15401,.T.) ;
#19758=ORIENTED_EDGE('',*,*,#15369,.F.) ;
#19759=ORIENTED_EDGE('',*,*,#15416,.T.) ;
#19760=ORIENTED_EDGE('',*,*,#14955,.F.) ;
#19761=ORIENTED_EDGE('',*,*,#15400,.T.) ;
#19762=ORIENTED_EDGE('',*,*,#15386,.F.) ;
#19763=ORIENTED_EDGE('',*,*,#15417,.F.) ;
#19764=ORIENTED_EDGE('',*,*,#14968,.F.) ;
#19765=ORIENTED_EDGE('',*,*,#14786,.T.) ;
#19766=ORIENTED_EDGE('',*,*,#14951,.F.) ;
#19767=ORIENTED_EDGE('',*,*,#15398,.T.) ;
#19768=ORIENTED_EDGE('',*,*,#15212,.F.) ;
#19769=ORIENTED_EDGE('',*,*,#15411,.T.) ;
#19770=ORIENTED_EDGE('',*,*,#15201,.F.) ;
#19771=ORIENTED_EDGE('',*,*,#15418,.T.) ;
#19772=ORIENTED_EDGE('',*,*,#14855,.F.) ;
#19773=ORIENTED_EDGE('',*,*,#15410,.T.) ;
#19774=ORIENTED_EDGE('',*,*,#15382,.F.) ;
#19775=ORIENTED_EDGE('',*,*,#15419,.F.) ;
#19776=ORIENTED_EDGE('',*,*,#14972,.F.) ;
#19777=ORIENTED_EDGE('',*,*,#15395,.T.) ;
#19778=ORIENTED_EDGE('',*,*,#15365,.F.) ;
#19779=ORIENTED_EDGE('',*,*,#15420,.T.) ;
#19780=ORIENTED_EDGE('',*,*,#14959,.F.) ;
#19781=ORIENTED_EDGE('',*,*,#15408,.T.) ;
#19782=ORIENTED_EDGE('',*,*,#15378,.F.) ;
#19783=ORIENTED_EDGE('',*,*,#15421,.F.) ;
#19784=ORIENTED_EDGE('',*,*,#14976,.F.) ;
#19785=ORIENTED_EDGE('',*,*,#15393,.T.) ;
#19786=ORIENTED_EDGE('',*,*,#15361,.F.) ;
#19787=ORIENTED_EDGE('',*,*,#15422,.T.) ;
#19788=ORIENTED_EDGE('',*,*,#14963,.F.) ;
#19789=ORIENTED_EDGE('',*,*,#15391,.T.) ;
#19790=ORIENTED_EDGE('',*,*,#15228,.F.) ;
#19791=ORIENTED_EDGE('',*,*,#15423,.T.) ;
#19792=ORIENTED_EDGE('',*,*,#14979,.F.) ;
#19793=ORIENTED_EDGE('',*,*,#15406,.T.) ;
#19794=ORIENTED_EDGE('',*,*,#15374,.F.) ;
#19795=ORIENTED_EDGE('',*,*,#15424,.T.) ;
#19796=ORIENTED_EDGE('',*,*,#14985,.F.) ;
#19797=ORIENTED_EDGE('',*,*,#15403,.T.) ;
#19798=ORIENTED_EDGE('',*,*,#14871,.F.) ;
#19799=ORIENTED_EDGE('',*,*,#15425,.T.) ;
#19800=ORIENTED_EDGE('',*,*,#15185,.F.) ;
#19801=ORIENTED_EDGE('',*,*,#15412,.T.) ;
#19802=ORIENTED_EDGE('',*,*,#15182,.F.) ;
#19803=ORIENTED_EDGE('',*,*,#15426,.T.) ;
#19804=ORIENTED_EDGE('',*,*,#14874,.F.) ;
#19805=ORIENTED_EDGE('',*,*,#15427,.F.) ;
#19806=ORIENTED_EDGE('',*,*,#15143,.F.) ;
#19807=ORIENTED_EDGE('',*,*,#15428,.F.) ;
#19808=ORIENTED_EDGE('',*,*,#14913,.F.) ;
#19809=ORIENTED_EDGE('',*,*,#15418,.F.) ;
#19810=ORIENTED_EDGE('',*,*,#15200,.F.) ;
#19811=ORIENTED_EDGE('',*,*,#15429,.F.) ;
#19812=ORIENTED_EDGE('',*,*,#14856,.F.) ;
#19813=ORIENTED_EDGE('',*,*,#15430,.F.) ;
#19814=ORIENTED_EDGE('',*,*,#14914,.F.) ;
#19815=ORIENTED_EDGE('',*,*,#15428,.T.) ;
#19816=ORIENTED_EDGE('',*,*,#15142,.F.) ;
#19817=ORIENTED_EDGE('',*,*,#15431,.F.) ;
#19818=ORIENTED_EDGE('',*,*,#15118,.F.) ;
#19819=ORIENTED_EDGE('',*,*,#15432,.F.) ;
#19820=ORIENTED_EDGE('',*,*,#15221,.F.) ;
#19821=ORIENTED_EDGE('',*,*,#15433,.F.) ;
#19822=ORIENTED_EDGE('',*,*,#14947,.F.) ;
#19823=ORIENTED_EDGE('',*,*,#14851,.F.) ;
#19824=ORIENTED_EDGE('',*,*,#15211,.F.) ;
#19825=ORIENTED_EDGE('',*,*,#15434,.F.) ;
#19826=ORIENTED_EDGE('',*,*,#14945,.F.) ;
#19827=ORIENTED_EDGE('',*,*,#14848,.F.) ;
#19828=ORIENTED_EDGE('',*,*,#15209,.F.) ;
#19829=ORIENTED_EDGE('',*,*,#15435,.F.) ;
#19830=ORIENTED_EDGE('',*,*,#14943,.F.) ;
#19831=ORIENTED_EDGE('',*,*,#14842,.F.) ;
#19832=ORIENTED_EDGE('',*,*,#15207,.F.) ;
#19833=ORIENTED_EDGE('',*,*,#15397,.T.) ;
#19834=ORIENTED_EDGE('',*,*,#14949,.F.) ;
#19835=ORIENTED_EDGE('',*,*,#14830,.F.) ;
#19836=ORIENTED_EDGE('',*,*,#15214,.F.) ;
#19837=ORIENTED_EDGE('',*,*,#15436,.F.) ;
#19838=ORIENTED_EDGE('',*,*,#15341,.F.) ;
#19839=ORIENTED_EDGE('',*,*,#15437,.F.) ;
#19840=ORIENTED_EDGE('',*,*,#15096,.F.) ;
#19841=ORIENTED_EDGE('',*,*,#15438,.F.) ;
#19842=ORIENTED_EDGE('',*,*,#15345,.F.) ;
#19843=ORIENTED_EDGE('',*,*,#15439,.F.) ;
#19844=ORIENTED_EDGE('',*,*,#15100,.F.) ;
#19845=ORIENTED_EDGE('',*,*,#15440,.F.) ;
#19846=ORIENTED_EDGE('',*,*,#15349,.F.) ;
#19847=ORIENTED_EDGE('',*,*,#15441,.F.) ;
#19848=ORIENTED_EDGE('',*,*,#15104,.F.) ;
#19849=ORIENTED_EDGE('',*,*,#15442,.F.) ;
#19850=ORIENTED_EDGE('',*,*,#15353,.F.) ;
#19851=ORIENTED_EDGE('',*,*,#15443,.F.) ;
#19852=ORIENTED_EDGE('',*,*,#15108,.F.) ;
#19853=ORIENTED_EDGE('',*,*,#15444,.F.) ;
#19854=ORIENTED_EDGE('',*,*,#15357,.F.) ;
#19855=ORIENTED_EDGE('',*,*,#15445,.F.) ;
#19856=ORIENTED_EDGE('',*,*,#15112,.F.) ;
#19857=ORIENTED_EDGE('',*,*,#15446,.F.) ;
#19858=ORIENTED_EDGE('',*,*,#14857,.F.) ;
#19859=ORIENTED_EDGE('',*,*,#15429,.T.) ;
#19860=ORIENTED_EDGE('',*,*,#15199,.F.) ;
#19861=ORIENTED_EDGE('',*,*,#15447,.F.) ;
#19862=ORIENTED_EDGE('',*,*,#14941,.F.) ;
#19863=ORIENTED_EDGE('',*,*,#14836,.F.) ;
#19864=ORIENTED_EDGE('',*,*,#15205,.F.) ;
#19865=ORIENTED_EDGE('',*,*,#14782,.T.) ;
#19866=ORIENTED_EDGE('',*,*,#14942,.F.) ;
#19867=ORIENTED_EDGE('',*,*,#15447,.T.) ;
#19868=ORIENTED_EDGE('',*,*,#15204,.F.) ;
#19869=ORIENTED_EDGE('',*,*,#15417,.T.) ;
#19870=ORIENTED_EDGE('',*,*,#15385,.F.) ;
#19871=ORIENTED_EDGE('',*,*,#15448,.F.) ;
#19872=ORIENTED_EDGE('',*,*,#14969,.F.) ;
#19873=ORIENTED_EDGE('',*,*,#15446,.T.) ;
#19874=ORIENTED_EDGE('',*,*,#15198,.F.) ;
#19875=ORIENTED_EDGE('',*,*,#15449,.T.) ;
#19876=ORIENTED_EDGE('',*,*,#14858,.F.) ;
#19877=ORIENTED_EDGE('',*,*,#14778,.T.) ;
#19878=ORIENTED_EDGE('',*,*,#14944,.F.) ;
#19879=ORIENTED_EDGE('',*,*,#15435,.T.) ;
#19880=ORIENTED_EDGE('',*,*,#15206,.F.) ;
#19881=ORIENTED_EDGE('',*,*,#15445,.T.) ;
#19882=ORIENTED_EDGE('',*,*,#15356,.F.) ;
#19883=ORIENTED_EDGE('',*,*,#15450,.T.) ;
#19884=ORIENTED_EDGE('',*,*,#15113,.F.) ;
#19885=ORIENTED_EDGE('',*,*,#14774,.T.) ;
#19886=ORIENTED_EDGE('',*,*,#14946,.F.) ;
#19887=ORIENTED_EDGE('',*,*,#15434,.T.) ;
#19888=ORIENTED_EDGE('',*,*,#15208,.F.) ;
#19889=ORIENTED_EDGE('',*,*,#15443,.T.) ;
#19890=ORIENTED_EDGE('',*,*,#15352,.F.) ;
#19891=ORIENTED_EDGE('',*,*,#15451,.T.) ;
#19892=ORIENTED_EDGE('',*,*,#15109,.F.) ;
#19893=ORIENTED_EDGE('',*,*,#14770,.T.) ;
#19894=ORIENTED_EDGE('',*,*,#14948,.F.) ;
#19895=ORIENTED_EDGE('',*,*,#15433,.T.) ;
#19896=ORIENTED_EDGE('',*,*,#15210,.F.) ;
#19897=ORIENTED_EDGE('',*,*,#15441,.T.) ;
#19898=ORIENTED_EDGE('',*,*,#15348,.F.) ;
#19899=ORIENTED_EDGE('',*,*,#15452,.T.) ;
#19900=ORIENTED_EDGE('',*,*,#15105,.F.) ;
#19901=ORIENTED_EDGE('',*,*,#14766,.T.) ;
#19902=ORIENTED_EDGE('',*,*,#15119,.F.) ;
#19903=ORIENTED_EDGE('',*,*,#15431,.T.) ;
#19904=ORIENTED_EDGE('',*,*,#15220,.F.) ;
#19905=ORIENTED_EDGE('',*,*,#15439,.T.) ;
#19906=ORIENTED_EDGE('',*,*,#15344,.F.) ;
#19907=ORIENTED_EDGE('',*,*,#15453,.T.) ;
#19908=ORIENTED_EDGE('',*,*,#15101,.F.) ;
#19909=ORIENTED_EDGE('',*,*,#15430,.T.) ;
#19910=ORIENTED_EDGE('',*,*,#15141,.F.) ;
#19911=ORIENTED_EDGE('',*,*,#15454,.T.) ;
#19912=ORIENTED_EDGE('',*,*,#14915,.F.) ;
#19913=ORIENTED_EDGE('',*,*,#15437,.T.) ;
#19914=ORIENTED_EDGE('',*,*,#15340,.F.) ;
#19915=ORIENTED_EDGE('',*,*,#15455,.T.) ;
#19916=ORIENTED_EDGE('',*,*,#15097,.F.) ;
#19917=ORIENTED_EDGE('',*,*,#15456,.F.) ;
#19918=ORIENTED_EDGE('',*,*,#15123,.F.) ;
#19919=ORIENTED_EDGE('',*,*,#15457,.F.) ;
#19920=ORIENTED_EDGE('',*,*,#14933,.F.) ;
#19921=ORIENTED_EDGE('',*,*,#15458,.F.) ;
#19922=ORIENTED_EDGE('',*,*,#15178,.F.) ;
#19923=ORIENTED_EDGE('',*,*,#15459,.F.) ;
#19924=ORIENTED_EDGE('',*,*,#14878,.F.) ;
#19925=ORIENTED_EDGE('',*,*,#15422,.F.) ;
#19926=ORIENTED_EDGE('',*,*,#15360,.F.) ;
#19927=ORIENTED_EDGE('',*,*,#15460,.F.) ;
#19928=ORIENTED_EDGE('',*,*,#14964,.F.) ;
#19929=ORIENTED_EDGE('',*,*,#15420,.F.) ;
#19930=ORIENTED_EDGE('',*,*,#15364,.F.) ;
#19931=ORIENTED_EDGE('',*,*,#15461,.F.) ;
#19932=ORIENTED_EDGE('',*,*,#14960,.F.) ;
#19933=ORIENTED_EDGE('',*,*,#15462,.F.) ;
#19934=ORIENTED_EDGE('',*,*,#14980,.F.) ;
#19935=ORIENTED_EDGE('',*,*,#15423,.F.) ;
#19936=ORIENTED_EDGE('',*,*,#15227,.F.) ;
#19937=ORIENTED_EDGE('',*,*,#14821,.F.) ;
#19938=ORIENTED_EDGE('',*,*,#14934,.F.) ;
#19939=ORIENTED_EDGE('',*,*,#15457,.T.) ;
#19940=ORIENTED_EDGE('',*,*,#15122,.F.) ;
#19941=ORIENTED_EDGE('',*,*,#15416,.F.) ;
#19942=ORIENTED_EDGE('',*,*,#15368,.F.) ;
#19943=ORIENTED_EDGE('',*,*,#15463,.F.) ;
#19944=ORIENTED_EDGE('',*,*,#14956,.F.) ;
#19945=ORIENTED_EDGE('',*,*,#15464,.F.) ;
#19946=ORIENTED_EDGE('',*,*,#15232,.F.) ;
#19947=ORIENTED_EDGE('',*,*,#15465,.F.) ;
#19948=ORIENTED_EDGE('',*,*,#15080,.F.) ;
#19949=ORIENTED_EDGE('',*,*,#15466,.F.) ;
#19950=ORIENTED_EDGE('',*,*,#15087,.F.) ;
#19951=ORIENTED_EDGE('',*,*,#15467,.F.) ;
#19952=ORIENTED_EDGE('',*,*,#15241,.F.) ;
#19953=ORIENTED_EDGE('',*,*,#15444,.T.) ;
#19954=ORIENTED_EDGE('',*,*,#15115,.F.) ;
#19955=ORIENTED_EDGE('',*,*,#15468,.F.) ;
#19956=ORIENTED_EDGE('',*,*,#15354,.F.) ;
#19957=ORIENTED_EDGE('',*,*,#15469,.F.) ;
#19958=ORIENTED_EDGE('',*,*,#15091,.F.) ;
#19959=ORIENTED_EDGE('',*,*,#15470,.F.) ;
#19960=ORIENTED_EDGE('',*,*,#15237,.F.) ;
#19961=ORIENTED_EDGE('',*,*,#15471,.F.) ;
#19962=ORIENTED_EDGE('',*,*,#15095,.F.) ;
#19963=ORIENTED_EDGE('',*,*,#15472,.F.) ;
#19964=ORIENTED_EDGE('',*,*,#15233,.F.) ;
#19965=ORIENTED_EDGE('',*,*,#15473,.F.) ;
#19966=ORIENTED_EDGE('',*,*,#14879,.F.) ;
#19967=ORIENTED_EDGE('',*,*,#15459,.T.) ;
#19968=ORIENTED_EDGE('',*,*,#15177,.F.) ;
#19969=ORIENTED_EDGE('',*,*,#15399,.T.) ;
#19970=ORIENTED_EDGE('',*,*,#14970,.F.) ;
#19971=ORIENTED_EDGE('',*,*,#15448,.T.) ;
#19972=ORIENTED_EDGE('',*,*,#15384,.F.) ;
#19973=ORIENTED_EDGE('',*,*,#15409,.T.) ;
#19974=ORIENTED_EDGE('',*,*,#14974,.F.) ;
#19975=ORIENTED_EDGE('',*,*,#15474,.F.) ;
#19976=ORIENTED_EDGE('',*,*,#15380,.F.) ;
#19977=ORIENTED_EDGE('',*,*,#15471,.T.) ;
#19978=ORIENTED_EDGE('',*,*,#15236,.F.) ;
#19979=ORIENTED_EDGE('',*,*,#15475,.F.) ;
#19980=ORIENTED_EDGE('',*,*,#15092,.F.) ;
#19981=ORIENTED_EDGE('',*,*,#15402,.T.) ;
#19982=ORIENTED_EDGE('',*,*,#14957,.F.) ;
#19983=ORIENTED_EDGE('',*,*,#15463,.T.) ;
#19984=ORIENTED_EDGE('',*,*,#15367,.F.) ;
#19985=ORIENTED_EDGE('',*,*,#15469,.T.) ;
#19986=ORIENTED_EDGE('',*,*,#15240,.F.) ;
#19987=ORIENTED_EDGE('',*,*,#15476,.T.) ;
#19988=ORIENTED_EDGE('',*,*,#15088,.F.) ;
#19989=ORIENTED_EDGE('',*,*,#15414,.T.) ;
#19990=ORIENTED_EDGE('',*,*,#14953,.F.) ;
#19991=ORIENTED_EDGE('',*,*,#15415,.T.) ;
#19992=ORIENTED_EDGE('',*,*,#15371,.F.) ;
#19993=ORIENTED_EDGE('',*,*,#15456,.T.) ;
#19994=ORIENTED_EDGE('',*,*,#14932,.F.) ;
#19995=ORIENTED_EDGE('',*,*,#15477,.T.) ;
#19996=ORIENTED_EDGE('',*,*,#15124,.F.) ;
#19997=ORIENTED_EDGE('',*,*,#15462,.T.) ;
#19998=ORIENTED_EDGE('',*,*,#15226,.F.) ;
#19999=ORIENTED_EDGE('',*,*,#15478,.F.) ;
#20000=ORIENTED_EDGE('',*,*,#14981,.F.) ;
#20001=ORIENTED_EDGE('',*,*,#15458,.T.) ;
#20002=ORIENTED_EDGE('',*,*,#14877,.F.) ;
#20003=ORIENTED_EDGE('',*,*,#15479,.T.) ;
#20004=ORIENTED_EDGE('',*,*,#15179,.F.) ;
#20005=ORIENTED_EDGE('',*,*,#15473,.T.) ;
#20006=ORIENTED_EDGE('',*,*,#15176,.F.) ;
#20007=ORIENTED_EDGE('',*,*,#15480,.T.) ;
#20008=ORIENTED_EDGE('',*,*,#14880,.F.) ;
#20009=ORIENTED_EDGE('',*,*,#15396,.T.) ;
#20010=ORIENTED_EDGE('',*,*,#14961,.F.) ;
#20011=ORIENTED_EDGE('',*,*,#15461,.T.) ;
#20012=ORIENTED_EDGE('',*,*,#15363,.F.) ;
#20013=ORIENTED_EDGE('',*,*,#15466,.T.) ;
#20014=ORIENTED_EDGE('',*,*,#15244,.F.) ;
#20015=ORIENTED_EDGE('',*,*,#15481,.T.) ;
#20016=ORIENTED_EDGE('',*,*,#15084,.F.) ;
#20017=ORIENTED_EDGE('',*,*,#15394,.T.) ;
#20018=ORIENTED_EDGE('',*,*,#14965,.F.) ;
#20019=ORIENTED_EDGE('',*,*,#15460,.T.) ;
#20020=ORIENTED_EDGE('',*,*,#15359,.F.) ;
#20021=ORIENTED_EDGE('',*,*,#15465,.T.) ;
#20022=ORIENTED_EDGE('',*,*,#15231,.F.) ;
#20023=ORIENTED_EDGE('',*,*,#15482,.T.) ;
#20024=ORIENTED_EDGE('',*,*,#15081,.F.) ;
#20025=ORIENTED_EDGE('',*,*,#15483,.F.) ;
#20026=ORIENTED_EDGE('',*,*,#15146,.F.) ;
#20027=ORIENTED_EDGE('',*,*,#15484,.F.) ;
#20028=ORIENTED_EDGE('',*,*,#14910,.F.) ;
#20029=ORIENTED_EDGE('',*,*,#15449,.F.) ;
#20030=ORIENTED_EDGE('',*,*,#15197,.F.) ;
#20031=ORIENTED_EDGE('',*,*,#15485,.F.) ;
#20032=ORIENTED_EDGE('',*,*,#14859,.F.) ;
#20033=ORIENTED_EDGE('',*,*,#15486,.F.) ;
#20034=ORIENTED_EDGE('',*,*,#15333,.F.) ;
#20035=ORIENTED_EDGE('',*,*,#15487,.F.) ;
#20036=ORIENTED_EDGE('',*,*,#15069,.F.) ;
#20037=ORIENTED_EDGE('',*,*,#15488,.F.) ;
#20038=ORIENTED_EDGE('',*,*,#15098,.F.) ;
#20039=ORIENTED_EDGE('',*,*,#15455,.F.) ;
#20040=ORIENTED_EDGE('',*,*,#15339,.F.) ;
#20041=ORIENTED_EDGE('',*,*,#15489,.F.) ;
#20042=ORIENTED_EDGE('',*,*,#15102,.F.) ;
#20043=ORIENTED_EDGE('',*,*,#15453,.F.) ;
#20044=ORIENTED_EDGE('',*,*,#15343,.F.) ;
#20045=ORIENTED_EDGE('',*,*,#15490,.F.) ;
#20046=ORIENTED_EDGE('',*,*,#15106,.F.) ;
#20047=ORIENTED_EDGE('',*,*,#15452,.F.) ;
#20048=ORIENTED_EDGE('',*,*,#15347,.F.) ;
#20049=ORIENTED_EDGE('',*,*,#15491,.F.) ;
#20050=ORIENTED_EDGE('',*,*,#14911,.F.) ;
#20051=ORIENTED_EDGE('',*,*,#15484,.T.) ;
#20052=ORIENTED_EDGE('',*,*,#15145,.F.) ;
#20053=ORIENTED_EDGE('',*,*,#15468,.T.) ;
#20054=ORIENTED_EDGE('',*,*,#15114,.F.) ;
#20055=ORIENTED_EDGE('',*,*,#15450,.F.) ;
#20056=ORIENTED_EDGE('',*,*,#15355,.F.) ;
#20057=ORIENTED_EDGE('',*,*,#15492,.F.) ;
#20058=ORIENTED_EDGE('',*,*,#15322,.F.) ;
#20059=ORIENTED_EDGE('',*,*,#15493,.F.) ;
#20060=ORIENTED_EDGE('',*,*,#15057,.F.) ;
#20061=ORIENTED_EDGE('',*,*,#15494,.F.) ;
#20062=ORIENTED_EDGE('',*,*,#15326,.F.) ;
#20063=ORIENTED_EDGE('',*,*,#15495,.F.) ;
#20064=ORIENTED_EDGE('',*,*,#15061,.F.) ;
#20065=ORIENTED_EDGE('',*,*,#15496,.F.) ;
#20066=ORIENTED_EDGE('',*,*,#15330,.F.) ;
#20067=ORIENTED_EDGE('',*,*,#15497,.F.) ;
#20068=ORIENTED_EDGE('',*,*,#15065,.F.) ;
#20069=ORIENTED_EDGE('',*,*,#15498,.F.) ;
#20070=ORIENTED_EDGE('',*,*,#15337,.F.) ;
#20071=ORIENTED_EDGE('',*,*,#15499,.F.) ;
#20072=ORIENTED_EDGE('',*,*,#15072,.F.) ;
#20073=ORIENTED_EDGE('',*,*,#15500,.F.) ;
#20074=ORIENTED_EDGE('',*,*,#15079,.F.) ;
#20075=ORIENTED_EDGE('',*,*,#15501,.F.) ;
#20076=ORIENTED_EDGE('',*,*,#15315,.F.) ;
#20077=ORIENTED_EDGE('',*,*,#15502,.F.) ;
#20078=ORIENTED_EDGE('',*,*,#14860,.F.) ;
#20079=ORIENTED_EDGE('',*,*,#15485,.T.) ;
#20080=ORIENTED_EDGE('',*,*,#15196,.F.) ;
#20081=ORIENTED_EDGE('',*,*,#15503,.F.) ;
#20082=ORIENTED_EDGE('',*,*,#15110,.F.) ;
#20083=ORIENTED_EDGE('',*,*,#15451,.F.) ;
#20084=ORIENTED_EDGE('',*,*,#15351,.F.) ;
#20085=ORIENTED_EDGE('',*,*,#15442,.T.) ;
#20086=ORIENTED_EDGE('',*,*,#15111,.F.) ;
#20087=ORIENTED_EDGE('',*,*,#15503,.T.) ;
#20088=ORIENTED_EDGE('',*,*,#15350,.F.) ;
#20089=ORIENTED_EDGE('',*,*,#14812,.T.) ;
#20090=ORIENTED_EDGE('',*,*,#14935,.F.) ;
#20091=ORIENTED_EDGE('',*,*,#14827,.F.) ;
#20092=ORIENTED_EDGE('',*,*,#15223,.F.) ;
#20093=ORIENTED_EDGE('',*,*,#15475,.T.) ;
#20094=ORIENTED_EDGE('',*,*,#15235,.F.) ;
#20095=ORIENTED_EDGE('',*,*,#15504,.F.) ;
#20096=ORIENTED_EDGE('',*,*,#15093,.F.) ;
#20097=ORIENTED_EDGE('',*,*,#15502,.T.) ;
#20098=ORIENTED_EDGE('',*,*,#15195,.F.) ;
#20099=ORIENTED_EDGE('',*,*,#15505,.T.) ;
#20100=ORIENTED_EDGE('',*,*,#14861,.F.) ;
#20101=ORIENTED_EDGE('',*,*,#15427,.T.) ;
#20102=ORIENTED_EDGE('',*,*,#14912,.F.) ;
#20103=ORIENTED_EDGE('',*,*,#15491,.T.) ;
#20104=ORIENTED_EDGE('',*,*,#15144,.F.) ;
#20105=ORIENTED_EDGE('',*,*,#15486,.T.) ;
#20106=ORIENTED_EDGE('',*,*,#15071,.F.) ;
#20107=ORIENTED_EDGE('',*,*,#15506,.T.) ;
#20108=ORIENTED_EDGE('',*,*,#15331,.F.) ;
#20109=ORIENTED_EDGE('',*,*,#15500,.T.) ;
#20110=ORIENTED_EDGE('',*,*,#15318,.F.) ;
#20111=ORIENTED_EDGE('',*,*,#15507,.T.) ;
#20112=ORIENTED_EDGE('',*,*,#15076,.F.) ;
#20113=ORIENTED_EDGE('',*,*,#15440,.T.) ;
#20114=ORIENTED_EDGE('',*,*,#15107,.F.) ;
#20115=ORIENTED_EDGE('',*,*,#15490,.T.) ;
#20116=ORIENTED_EDGE('',*,*,#15346,.F.) ;
#20117=ORIENTED_EDGE('',*,*,#15499,.T.) ;
#20118=ORIENTED_EDGE('',*,*,#15336,.F.) ;
#20119=ORIENTED_EDGE('',*,*,#15508,.T.) ;
#20120=ORIENTED_EDGE('',*,*,#15073,.F.) ;
#20121=ORIENTED_EDGE('',*,*,#15438,.T.) ;
#20122=ORIENTED_EDGE('',*,*,#15103,.F.) ;
#20123=ORIENTED_EDGE('',*,*,#15489,.T.) ;
#20124=ORIENTED_EDGE('',*,*,#15342,.F.) ;
#20125=ORIENTED_EDGE('',*,*,#15497,.T.) ;
#20126=ORIENTED_EDGE('',*,*,#15329,.F.) ;
#20127=ORIENTED_EDGE('',*,*,#15509,.T.) ;
#20128=ORIENTED_EDGE('',*,*,#15066,.F.) ;
#20129=ORIENTED_EDGE('',*,*,#15436,.T.) ;
#20130=ORIENTED_EDGE('',*,*,#15099,.F.) ;
#20131=ORIENTED_EDGE('',*,*,#15488,.T.) ;
#20132=ORIENTED_EDGE('',*,*,#15338,.F.) ;
#20133=ORIENTED_EDGE('',*,*,#15495,.T.) ;
#20134=ORIENTED_EDGE('',*,*,#15325,.F.) ;
#20135=ORIENTED_EDGE('',*,*,#15510,.T.) ;
#20136=ORIENTED_EDGE('',*,*,#15062,.F.) ;
#20137=ORIENTED_EDGE('',*,*,#15487,.T.) ;
#20138=ORIENTED_EDGE('',*,*,#15332,.F.) ;
#20139=ORIENTED_EDGE('',*,*,#15506,.F.) ;
#20140=ORIENTED_EDGE('',*,*,#15070,.F.) ;
#20141=ORIENTED_EDGE('',*,*,#15493,.T.) ;
#20142=ORIENTED_EDGE('',*,*,#15321,.F.) ;
#20143=ORIENTED_EDGE('',*,*,#15511,.T.) ;
#20144=ORIENTED_EDGE('',*,*,#15058,.F.) ;
#20145=ORIENTED_EDGE('',*,*,#15512,.F.) ;
#20146=ORIENTED_EDGE('',*,*,#15126,.F.) ;
#20147=ORIENTED_EDGE('',*,*,#15513,.F.) ;
#20148=ORIENTED_EDGE('',*,*,#14930,.F.) ;
#20149=ORIENTED_EDGE('',*,*,#15514,.F.) ;
#20150=ORIENTED_EDGE('',*,*,#15044,.F.) ;
#20151=ORIENTED_EDGE('',*,*,#15515,.F.) ;
#20152=ORIENTED_EDGE('',*,*,#15311,.F.) ;
#20153=ORIENTED_EDGE('',*,*,#15516,.F.) ;
#20154=ORIENTED_EDGE('',*,*,#15048,.F.) ;
#20155=ORIENTED_EDGE('',*,*,#15517,.F.) ;
#20156=ORIENTED_EDGE('',*,*,#15256,.F.) ;
#20157=ORIENTED_EDGE('',*,*,#15518,.F.) ;
#20158=ORIENTED_EDGE('',*,*,#15052,.F.) ;
#20159=ORIENTED_EDGE('',*,*,#15519,.F.) ;
#20160=ORIENTED_EDGE('',*,*,#15252,.F.) ;
#20161=ORIENTED_EDGE('',*,*,#15498,.T.) ;
#20162=ORIENTED_EDGE('',*,*,#15075,.F.) ;
#20163=ORIENTED_EDGE('',*,*,#15520,.F.) ;
#20164=ORIENTED_EDGE('',*,*,#15334,.F.) ;
#20165=ORIENTED_EDGE('',*,*,#15521,.F.) ;
#20166=ORIENTED_EDGE('',*,*,#15056,.F.) ;
#20167=ORIENTED_EDGE('',*,*,#15522,.F.) ;
#20168=ORIENTED_EDGE('',*,*,#15248,.F.) ;
#20169=ORIENTED_EDGE('',*,*,#15480,.F.) ;
#20170=ORIENTED_EDGE('',*,*,#15175,.F.) ;
#20171=ORIENTED_EDGE('',*,*,#15523,.F.) ;
#20172=ORIENTED_EDGE('',*,*,#14881,.F.) ;
#20173=ORIENTED_EDGE('',*,*,#15524,.F.) ;
#20174=ORIENTED_EDGE('',*,*,#15247,.F.) ;
#20175=ORIENTED_EDGE('',*,*,#15525,.F.) ;
#20176=ORIENTED_EDGE('',*,*,#15038,.F.) ;
#20177=ORIENTED_EDGE('',*,*,#15482,.F.) ;
#20178=ORIENTED_EDGE('',*,*,#15230,.F.) ;
#20179=ORIENTED_EDGE('',*,*,#15526,.F.) ;
#20180=ORIENTED_EDGE('',*,*,#15082,.F.) ;
#20181=ORIENTED_EDGE('',*,*,#15481,.F.) ;
#20182=ORIENTED_EDGE('',*,*,#15243,.F.) ;
#20183=ORIENTED_EDGE('',*,*,#15527,.F.) ;
#20184=ORIENTED_EDGE('',*,*,#15085,.F.) ;
#20185=ORIENTED_EDGE('',*,*,#15476,.F.) ;
#20186=ORIENTED_EDGE('',*,*,#15239,.F.) ;
#20187=ORIENTED_EDGE('',*,*,#15528,.F.) ;
#20188=ORIENTED_EDGE('',*,*,#15089,.F.) ;
#20189=ORIENTED_EDGE('',*,*,#15477,.F.) ;
#20190=ORIENTED_EDGE('',*,*,#14931,.F.) ;
#20191=ORIENTED_EDGE('',*,*,#15513,.T.) ;
#20192=ORIENTED_EDGE('',*,*,#15125,.F.) ;
#20193=ORIENTED_EDGE('',*,*,#15529,.F.) ;
#20194=ORIENTED_EDGE('',*,*,#14882,.F.) ;
#20195=ORIENTED_EDGE('',*,*,#15523,.T.) ;
#20196=ORIENTED_EDGE('',*,*,#15174,.F.) ;
#20197=ORIENTED_EDGE('',*,*,#15472,.T.) ;
#20198=ORIENTED_EDGE('',*,*,#15094,.F.) ;
#20199=ORIENTED_EDGE('',*,*,#15504,.T.) ;
#20200=ORIENTED_EDGE('',*,*,#15234,.F.) ;
#20201=ORIENTED_EDGE('',*,*,#15407,.T.) ;
#20202=ORIENTED_EDGE('',*,*,#14978,.F.) ;
#20203=ORIENTED_EDGE('',*,*,#15530,.F.) ;
#20204=ORIENTED_EDGE('',*,*,#15376,.F.) ;
#20205=ORIENTED_EDGE('',*,*,#15521,.T.) ;
#20206=ORIENTED_EDGE('',*,*,#15251,.F.) ;
#20207=ORIENTED_EDGE('',*,*,#15531,.F.) ;
#20208=ORIENTED_EDGE('',*,*,#15053,.F.) ;
#20209=ORIENTED_EDGE('',*,*,#15474,.T.) ;
#20210=ORIENTED_EDGE('',*,*,#14973,.F.) ;
#20211=ORIENTED_EDGE('',*,*,#15419,.T.) ;
#20212=ORIENTED_EDGE('',*,*,#15381,.F.) ;
#20213=ORIENTED_EDGE('',*,*,#14833,.T.) ;
#20214=ORIENTED_EDGE('',*,*,#15216,.F.) ;
#20215=ORIENTED_EDGE('',*,*,#15532,.T.) ;
#20216=ORIENTED_EDGE('',*,*,#14936,.F.) ;
#20217=ORIENTED_EDGE('',*,*,#15512,.T.) ;
#20218=ORIENTED_EDGE('',*,*,#14929,.F.) ;
#20219=ORIENTED_EDGE('',*,*,#15533,.T.) ;
#20220=ORIENTED_EDGE('',*,*,#15127,.F.) ;
#20221=ORIENTED_EDGE('',*,*,#15470,.T.) ;
#20222=ORIENTED_EDGE('',*,*,#15090,.F.) ;
#20223=ORIENTED_EDGE('',*,*,#15528,.T.) ;
#20224=ORIENTED_EDGE('',*,*,#15238,.F.) ;
#20225=ORIENTED_EDGE('',*,*,#15518,.T.) ;
#20226=ORIENTED_EDGE('',*,*,#15255,.F.) ;
#20227=ORIENTED_EDGE('',*,*,#15534,.T.) ;
#20228=ORIENTED_EDGE('',*,*,#15049,.F.) ;
#20229=ORIENTED_EDGE('',*,*,#15467,.T.) ;
#20230=ORIENTED_EDGE('',*,*,#15086,.F.) ;
#20231=ORIENTED_EDGE('',*,*,#15527,.T.) ;
#20232=ORIENTED_EDGE('',*,*,#15242,.F.) ;
#20233=ORIENTED_EDGE('',*,*,#15516,.T.) ;
#20234=ORIENTED_EDGE('',*,*,#15259,.F.) ;
#20235=ORIENTED_EDGE('',*,*,#15535,.T.) ;
#20236=ORIENTED_EDGE('',*,*,#15045,.F.) ;
#20237=ORIENTED_EDGE('',*,*,#15464,.T.) ;
#20238=ORIENTED_EDGE('',*,*,#15083,.F.) ;
#20239=ORIENTED_EDGE('',*,*,#15526,.T.) ;
#20240=ORIENTED_EDGE('',*,*,#15229,.F.) ;
#20241=ORIENTED_EDGE('',*,*,#15514,.T.) ;
#20242=ORIENTED_EDGE('',*,*,#15314,.F.) ;
#20243=ORIENTED_EDGE('',*,*,#15536,.T.) ;
#20244=ORIENTED_EDGE('',*,*,#15041,.F.) ;
#20245=ORIENTED_EDGE('',*,*,#15525,.T.) ;
#20246=ORIENTED_EDGE('',*,*,#15246,.F.) ;
#20247=ORIENTED_EDGE('',*,*,#15537,.T.) ;
#20248=ORIENTED_EDGE('',*,*,#15039,.F.) ;
#20249=ORIENTED_EDGE('',*,*,#15529,.T.) ;
#20250=ORIENTED_EDGE('',*,*,#15173,.F.) ;
#20251=ORIENTED_EDGE('',*,*,#15538,.T.) ;
#20252=ORIENTED_EDGE('',*,*,#14883,.F.) ;
#20253=ORIENTED_EDGE('',*,*,#15505,.F.) ;
#20254=ORIENTED_EDGE('',*,*,#15194,.F.) ;
#20255=ORIENTED_EDGE('',*,*,#15539,.F.) ;
#20256=ORIENTED_EDGE('',*,*,#14862,.F.) ;
#20257=ORIENTED_EDGE('',*,*,#15507,.F.) ;
#20258=ORIENTED_EDGE('',*,*,#15317,.F.) ;
#20259=ORIENTED_EDGE('',*,*,#15540,.F.) ;
#20260=ORIENTED_EDGE('',*,*,#15077,.F.) ;
#20261=ORIENTED_EDGE('',*,*,#15541,.F.) ;
#20262=ORIENTED_EDGE('',*,*,#15059,.F.) ;
#20263=ORIENTED_EDGE('',*,*,#15511,.F.) ;
#20264=ORIENTED_EDGE('',*,*,#15320,.F.) ;
#20265=ORIENTED_EDGE('',*,*,#15542,.F.) ;
#20266=ORIENTED_EDGE('',*,*,#14908,.F.) ;
#20267=ORIENTED_EDGE('',*,*,#15543,.T.) ;
#20268=ORIENTED_EDGE('',*,*,#15148,.F.) ;
#20269=ORIENTED_EDGE('',*,*,#15544,.F.) ;
#20270=ORIENTED_EDGE('',*,*,#15063,.F.) ;
#20271=ORIENTED_EDGE('',*,*,#15510,.F.) ;
#20272=ORIENTED_EDGE('',*,*,#15324,.F.) ;
#20273=ORIENTED_EDGE('',*,*,#15520,.T.) ;
#20274=ORIENTED_EDGE('',*,*,#15074,.F.) ;
#20275=ORIENTED_EDGE('',*,*,#15508,.F.) ;
#20276=ORIENTED_EDGE('',*,*,#15335,.F.) ;
#20277=ORIENTED_EDGE('',*,*,#15545,.F.) ;
#20278=ORIENTED_EDGE('',*,*,#15067,.F.) ;
#20279=ORIENTED_EDGE('',*,*,#15509,.F.) ;
#20280=ORIENTED_EDGE('',*,*,#15328,.F.) ;
#20281=ORIENTED_EDGE('',*,*,#15546,.F.) ;
#20282=ORIENTED_EDGE('',*,*,#15150,.F.) ;
#20283=ORIENTED_EDGE('',*,*,#15547,.F.) ;
#20284=ORIENTED_EDGE('',*,*,#14906,.F.) ;
#20285=ORIENTED_EDGE('',*,*,#15548,.F.) ;
#20286=ORIENTED_EDGE('',*,*,#15271,.F.) ;
#20287=ORIENTED_EDGE('',*,*,#15549,.F.) ;
#20288=ORIENTED_EDGE('',*,*,#14999,.F.) ;
#20289=ORIENTED_EDGE('',*,*,#15550,.F.) ;
#20290=ORIENTED_EDGE('',*,*,#15267,.F.) ;
#20291=ORIENTED_EDGE('',*,*,#15551,.F.) ;
#20292=ORIENTED_EDGE('',*,*,#14995,.F.) ;
#20293=ORIENTED_EDGE('',*,*,#15552,.F.) ;
#20294=ORIENTED_EDGE('',*,*,#14990,.F.) ;
#20295=ORIENTED_EDGE('',*,*,#15553,.F.) ;
#20296=ORIENTED_EDGE('',*,*,#15272,.F.) ;
#20297=ORIENTED_EDGE('',*,*,#15554,.F.) ;
#20298=ORIENTED_EDGE('',*,*,#15263,.F.) ;
#20299=ORIENTED_EDGE('',*,*,#15555,.F.) ;
#20300=ORIENTED_EDGE('',*,*,#14991,.F.) ;
#20301=ORIENTED_EDGE('',*,*,#15556,.F.) ;
#20302=ORIENTED_EDGE('',*,*,#14864,.F.) ;
#20303=ORIENTED_EDGE('',*,*,#15557,.T.) ;
#20304=ORIENTED_EDGE('',*,*,#15192,.F.) ;
#20305=ORIENTED_EDGE('',*,*,#14907,.F.) ;
#20306=ORIENTED_EDGE('',*,*,#15547,.T.) ;
#20307=ORIENTED_EDGE('',*,*,#15149,.F.) ;
#20308=ORIENTED_EDGE('',*,*,#15543,.F.) ;
#20309=ORIENTED_EDGE('',*,*,#14863,.F.) ;
#20310=ORIENTED_EDGE('',*,*,#15539,.T.) ;
#20311=ORIENTED_EDGE('',*,*,#15193,.F.) ;
#20312=ORIENTED_EDGE('',*,*,#15557,.F.) ;
#20313=ORIENTED_EDGE('',*,*,#15531,.T.) ;
#20314=ORIENTED_EDGE('',*,*,#15250,.F.) ;
#20315=ORIENTED_EDGE('',*,*,#15558,.F.) ;
#20316=ORIENTED_EDGE('',*,*,#15054,.F.) ;
#20317=ORIENTED_EDGE('',*,*,#15554,.T.) ;
#20318=ORIENTED_EDGE('',*,*,#14994,.F.) ;
#20319=ORIENTED_EDGE('',*,*,#15559,.F.) ;
#20320=ORIENTED_EDGE('',*,*,#15260,.F.) ;
#20321=ORIENTED_EDGE('',*,*,#15496,.T.) ;
#20322=ORIENTED_EDGE('',*,*,#15068,.F.) ;
#20323=ORIENTED_EDGE('',*,*,#15545,.T.) ;
#20324=ORIENTED_EDGE('',*,*,#15327,.F.) ;
#20325=ORIENTED_EDGE('',*,*,#15530,.T.) ;
#20326=ORIENTED_EDGE('',*,*,#14977,.F.) ;
#20327=ORIENTED_EDGE('',*,*,#15421,.T.) ;
#20328=ORIENTED_EDGE('',*,*,#15377,.F.) ;
#20329=ORIENTED_EDGE('',*,*,#15556,.T.) ;
#20330=ORIENTED_EDGE('',*,*,#15191,.F.) ;
#20331=ORIENTED_EDGE('',*,*,#15560,.T.) ;
#20332=ORIENTED_EDGE('',*,*,#14865,.F.) ;
#20333=ORIENTED_EDGE('',*,*,#15494,.T.) ;
#20334=ORIENTED_EDGE('',*,*,#15064,.F.) ;
#20335=ORIENTED_EDGE('',*,*,#15544,.T.) ;
#20336=ORIENTED_EDGE('',*,*,#15323,.F.) ;
#20337=ORIENTED_EDGE('',*,*,#15555,.T.) ;
#20338=ORIENTED_EDGE('',*,*,#15262,.F.) ;
#20339=ORIENTED_EDGE('',*,*,#15561,.T.) ;
#20340=ORIENTED_EDGE('',*,*,#14992,.F.) ;
#20341=ORIENTED_EDGE('',*,*,#15483,.T.) ;
#20342=ORIENTED_EDGE('',*,*,#14909,.F.) ;
#20343=ORIENTED_EDGE('',*,*,#15542,.T.) ;
#20344=ORIENTED_EDGE('',*,*,#15147,.F.) ;
#20345=ORIENTED_EDGE('',*,*,#15546,.T.) ;
#20346=ORIENTED_EDGE('',*,*,#14905,.F.) ;
#20347=ORIENTED_EDGE('',*,*,#15562,.T.) ;
#20348=ORIENTED_EDGE('',*,*,#15151,.F.) ;
#20349=ORIENTED_EDGE('',*,*,#15552,.T.) ;
#20350=ORIENTED_EDGE('',*,*,#15275,.F.) ;
#20351=ORIENTED_EDGE('',*,*,#15563,.T.) ;
#20352=ORIENTED_EDGE('',*,*,#14987,.F.) ;
#20353=ORIENTED_EDGE('',*,*,#15492,.T.) ;
#20354=ORIENTED_EDGE('',*,*,#15060,.F.) ;
#20355=ORIENTED_EDGE('',*,*,#15541,.T.) ;
#20356=ORIENTED_EDGE('',*,*,#15319,.F.) ;
#20357=ORIENTED_EDGE('',*,*,#15551,.T.) ;
#20358=ORIENTED_EDGE('',*,*,#15266,.F.) ;
#20359=ORIENTED_EDGE('',*,*,#15564,.T.) ;
#20360=ORIENTED_EDGE('',*,*,#14996,.F.) ;
#20361=ORIENTED_EDGE('',*,*,#15501,.T.) ;
#20362=ORIENTED_EDGE('',*,*,#15078,.F.) ;
#20363=ORIENTED_EDGE('',*,*,#15540,.T.) ;
#20364=ORIENTED_EDGE('',*,*,#15316,.F.) ;
#20365=ORIENTED_EDGE('',*,*,#15549,.T.) ;
#20366=ORIENTED_EDGE('',*,*,#15270,.F.) ;
#20367=ORIENTED_EDGE('',*,*,#15565,.T.) ;
#20368=ORIENTED_EDGE('',*,*,#15000,.F.) ;
#20369=ORIENTED_EDGE('',*,*,#15538,.F.) ;
#20370=ORIENTED_EDGE('',*,*,#15172,.F.) ;
#20371=ORIENTED_EDGE('',*,*,#15566,.F.) ;
#20372=ORIENTED_EDGE('',*,*,#14884,.F.) ;
#20373=ORIENTED_EDGE('',*,*,#15536,.F.) ;
#20374=ORIENTED_EDGE('',*,*,#15313,.F.) ;
#20375=ORIENTED_EDGE('',*,*,#15567,.F.) ;
#20376=ORIENTED_EDGE('',*,*,#15042,.F.) ;
#20377=ORIENTED_EDGE('',*,*,#15535,.F.) ;
#20378=ORIENTED_EDGE('',*,*,#15258,.F.) ;
#20379=ORIENTED_EDGE('',*,*,#15568,.F.) ;
#20380=ORIENTED_EDGE('',*,*,#15046,.F.) ;
#20381=ORIENTED_EDGE('',*,*,#15533,.F.) ;
#20382=ORIENTED_EDGE('',*,*,#14928,.F.) ;
#20383=ORIENTED_EDGE('',*,*,#15569,.T.) ;
#20384=ORIENTED_EDGE('',*,*,#15128,.F.) ;
#20385=ORIENTED_EDGE('',*,*,#15534,.F.) ;
#20386=ORIENTED_EDGE('',*,*,#15254,.F.) ;
#20387=ORIENTED_EDGE('',*,*,#15570,.F.) ;
#20388=ORIENTED_EDGE('',*,*,#15050,.F.) ;
#20389=ORIENTED_EDGE('',*,*,#14808,.T.) ;
#20390=ORIENTED_EDGE('',*,*,#14937,.F.) ;
#20391=ORIENTED_EDGE('',*,*,#15532,.F.) ;
#20392=ORIENTED_EDGE('',*,*,#15215,.F.) ;
#20393=ORIENTED_EDGE('',*,*,#15571,.F.) ;
#20394=ORIENTED_EDGE('',*,*,#15130,.F.) ;
#20395=ORIENTED_EDGE('',*,*,#15572,.F.) ;
#20396=ORIENTED_EDGE('',*,*,#14926,.F.) ;
#20397=ORIENTED_EDGE('',*,*,#15573,.F.) ;
#20398=ORIENTED_EDGE('',*,*,#14886,.F.) ;
#20399=ORIENTED_EDGE('',*,*,#15574,.T.) ;
#20400=ORIENTED_EDGE('',*,*,#15170,.F.) ;
#20401=ORIENTED_EDGE('',*,*,#15575,.F.) ;
#20402=ORIENTED_EDGE('',*,*,#15014,.F.) ;
#20403=ORIENTED_EDGE('',*,*,#15576,.F.) ;
#20404=ORIENTED_EDGE('',*,*,#15276,.F.) ;
#20405=ORIENTED_EDGE('',*,*,#15577,.F.) ;
#20406=ORIENTED_EDGE('',*,*,#15010,.F.) ;
#20407=ORIENTED_EDGE('',*,*,#15578,.F.) ;
#20408=ORIENTED_EDGE('',*,*,#15303,.F.) ;
#20409=ORIENTED_EDGE('',*,*,#15579,.F.) ;
#20410=ORIENTED_EDGE('',*,*,#15006,.F.) ;
#20411=ORIENTED_EDGE('',*,*,#15580,.F.) ;
#20412=ORIENTED_EDGE('',*,*,#15307,.F.) ;
#20413=ORIENTED_EDGE('',*,*,#14885,.F.) ;
#20414=ORIENTED_EDGE('',*,*,#15566,.T.) ;
#20415=ORIENTED_EDGE('',*,*,#15171,.F.) ;
#20416=ORIENTED_EDGE('',*,*,#15574,.F.) ;
#20417=ORIENTED_EDGE('',*,*,#14927,.F.) ;
#20418=ORIENTED_EDGE('',*,*,#15572,.T.) ;
#20419=ORIENTED_EDGE('',*,*,#15129,.F.) ;
#20420=ORIENTED_EDGE('',*,*,#15569,.F.) ;
#20421=ORIENTED_EDGE('',*,*,#15579,.T.) ;
#20422=ORIENTED_EDGE('',*,*,#15310,.F.) ;
#20423=ORIENTED_EDGE('',*,*,#15581,.F.) ;
#20424=ORIENTED_EDGE('',*,*,#15003,.F.) ;
#20425=ORIENTED_EDGE('',*,*,#15559,.T.) ;
#20426=ORIENTED_EDGE('',*,*,#14993,.F.) ;
#20427=ORIENTED_EDGE('',*,*,#15561,.F.) ;
#20428=ORIENTED_EDGE('',*,*,#15261,.F.) ;
#20429=ORIENTED_EDGE('',*,*,#15522,.T.) ;
#20430=ORIENTED_EDGE('',*,*,#15055,.F.) ;
#20431=ORIENTED_EDGE('',*,*,#15558,.T.) ;
#20432=ORIENTED_EDGE('',*,*,#15249,.F.) ;
#20433=ORIENTED_EDGE('',*,*,#15519,.T.) ;
#20434=ORIENTED_EDGE('',*,*,#15051,.F.) ;
#20435=ORIENTED_EDGE('',*,*,#15570,.T.) ;
#20436=ORIENTED_EDGE('',*,*,#15253,.F.) ;
#20437=ORIENTED_EDGE('',*,*,#15577,.T.) ;
#20438=ORIENTED_EDGE('',*,*,#15306,.F.) ;
#20439=ORIENTED_EDGE('',*,*,#15582,.T.) ;
#20440=ORIENTED_EDGE('',*,*,#15007,.F.) ;
#20441=ORIENTED_EDGE('',*,*,#14839,.T.) ;
#20442=ORIENTED_EDGE('',*,*,#15218,.F.) ;
#20443=ORIENTED_EDGE('',*,*,#15583,.T.) ;
#20444=ORIENTED_EDGE('',*,*,#14938,.F.) ;
#20445=ORIENTED_EDGE('',*,*,#15517,.T.) ;
#20446=ORIENTED_EDGE('',*,*,#15047,.F.) ;
#20447=ORIENTED_EDGE('',*,*,#15568,.T.) ;
#20448=ORIENTED_EDGE('',*,*,#15257,.F.) ;
#20449=ORIENTED_EDGE('',*,*,#15575,.T.) ;
#20450=ORIENTED_EDGE('',*,*,#15279,.F.) ;
#20451=ORIENTED_EDGE('',*,*,#15584,.T.) ;
#20452=ORIENTED_EDGE('',*,*,#15011,.F.) ;
#20453=ORIENTED_EDGE('',*,*,#15576,.T.) ;
#20454=ORIENTED_EDGE('',*,*,#15013,.F.) ;
#20455=ORIENTED_EDGE('',*,*,#15585,.T.) ;
#20456=ORIENTED_EDGE('',*,*,#15277,.F.) ;
#20457=ORIENTED_EDGE('',*,*,#15515,.T.) ;
#20458=ORIENTED_EDGE('',*,*,#15043,.F.) ;
#20459=ORIENTED_EDGE('',*,*,#15567,.T.) ;
#20460=ORIENTED_EDGE('',*,*,#15312,.F.) ;
#20461=ORIENTED_EDGE('',*,*,#15573,.T.) ;
#20462=ORIENTED_EDGE('',*,*,#15169,.F.) ;
#20463=ORIENTED_EDGE('',*,*,#15586,.T.) ;
#20464=ORIENTED_EDGE('',*,*,#14887,.F.) ;
#20465=ORIENTED_EDGE('',*,*,#15560,.F.) ;
#20466=ORIENTED_EDGE('',*,*,#15190,.F.) ;
#20467=ORIENTED_EDGE('',*,*,#15587,.F.) ;
#20468=ORIENTED_EDGE('',*,*,#14866,.F.) ;
#20469=ORIENTED_EDGE('',*,*,#15588,.F.) ;
#20470=ORIENTED_EDGE('',*,*,#15153,.F.) ;
#20471=ORIENTED_EDGE('',*,*,#15589,.F.) ;
#20472=ORIENTED_EDGE('',*,*,#14903,.F.) ;
#20473=ORIENTED_EDGE('',*,*,#15590,.F.) ;
#20474=ORIENTED_EDGE('',*,*,#15294,.F.) ;
#20475=ORIENTED_EDGE('',*,*,#15591,.F.) ;
#20476=ORIENTED_EDGE('',*,*,#15023,.F.) ;
#20477=ORIENTED_EDGE('',*,*,#15592,.F.) ;
#20478=ORIENTED_EDGE('',*,*,#15298,.F.) ;
#20479=ORIENTED_EDGE('',*,*,#15593,.F.) ;
#20480=ORIENTED_EDGE('',*,*,#15015,.F.) ;
#20481=ORIENTED_EDGE('',*,*,#15594,.F.) ;
#20482=ORIENTED_EDGE('',*,*,#14867,.F.) ;
#20483=ORIENTED_EDGE('',*,*,#15587,.T.) ;
#20484=ORIENTED_EDGE('',*,*,#15189,.F.) ;
#20485=ORIENTED_EDGE('',*,*,#15595,.F.) ;
#20486=ORIENTED_EDGE('',*,*,#15302,.F.) ;
#20487=ORIENTED_EDGE('',*,*,#15596,.F.) ;
#20488=ORIENTED_EDGE('',*,*,#15019,.F.) ;
#20489=ORIENTED_EDGE('',*,*,#15405,.T.) ;
#20490=ORIENTED_EDGE('',*,*,#14986,.F.) ;
#20491=ORIENTED_EDGE('',*,*,#15424,.F.) ;
#20492=ORIENTED_EDGE('',*,*,#15373,.F.) ;
#20493=ORIENTED_EDGE('',*,*,#15597,.F.) ;
#20494=ORIENTED_EDGE('',*,*,#14988,.F.) ;
#20495=ORIENTED_EDGE('',*,*,#15563,.F.) ;
#20496=ORIENTED_EDGE('',*,*,#15274,.F.) ;
#20497=ORIENTED_EDGE('',*,*,#15598,.F.) ;
#20498=ORIENTED_EDGE('',*,*,#15001,.F.) ;
#20499=ORIENTED_EDGE('',*,*,#15565,.F.) ;
#20500=ORIENTED_EDGE('',*,*,#15269,.F.) ;
#20501=ORIENTED_EDGE('',*,*,#15562,.F.) ;
#20502=ORIENTED_EDGE('',*,*,#14904,.F.) ;
#20503=ORIENTED_EDGE('',*,*,#15589,.T.) ;
#20504=ORIENTED_EDGE('',*,*,#15152,.F.) ;
#20505=ORIENTED_EDGE('',*,*,#15599,.F.) ;
#20506=ORIENTED_EDGE('',*,*,#14997,.F.) ;
#20507=ORIENTED_EDGE('',*,*,#15564,.F.) ;
#20508=ORIENTED_EDGE('',*,*,#15265,.F.) ;
#20509=ORIENTED_EDGE('',*,*,#15550,.T.) ;
#20510=ORIENTED_EDGE('',*,*,#14998,.F.) ;
#20511=ORIENTED_EDGE('',*,*,#15599,.T.) ;
#20512=ORIENTED_EDGE('',*,*,#15264,.F.) ;
#20513=ORIENTED_EDGE('',*,*,#14804,.T.) ;
#20514=ORIENTED_EDGE('',*,*,#14939,.F.) ;
#20515=ORIENTED_EDGE('',*,*,#15583,.F.) ;
#20516=ORIENTED_EDGE('',*,*,#15217,.F.) ;
#20517=ORIENTED_EDGE('',*,*,#15581,.T.) ;
#20518=ORIENTED_EDGE('',*,*,#15309,.F.) ;
#20519=ORIENTED_EDGE('',*,*,#15600,.F.) ;
#20520=ORIENTED_EDGE('',*,*,#15004,.F.) ;
#20521=ORIENTED_EDGE('',*,*,#15548,.T.) ;
#20522=ORIENTED_EDGE('',*,*,#15002,.F.) ;
#20523=ORIENTED_EDGE('',*,*,#15598,.T.) ;
#20524=ORIENTED_EDGE('',*,*,#15268,.F.) ;
#20525=ORIENTED_EDGE('',*,*,#15596,.T.) ;
#20526=ORIENTED_EDGE('',*,*,#15301,.F.) ;
#20527=ORIENTED_EDGE('',*,*,#15601,.T.) ;
#20528=ORIENTED_EDGE('',*,*,#15020,.F.) ;
#20529=ORIENTED_EDGE('',*,*,#15594,.T.) ;
#20530=ORIENTED_EDGE('',*,*,#15188,.F.) ;
#20531=ORIENTED_EDGE('',*,*,#15602,.T.) ;
#20532=ORIENTED_EDGE('',*,*,#14868,.F.) ;
#20533=ORIENTED_EDGE('',*,*,#15593,.T.) ;
#20534=ORIENTED_EDGE('',*,*,#15297,.F.) ;
#20535=ORIENTED_EDGE('',*,*,#15603,.T.) ;
#20536=ORIENTED_EDGE('',*,*,#15016,.F.) ;
#20537=ORIENTED_EDGE('',*,*,#15553,.T.) ;
#20538=ORIENTED_EDGE('',*,*,#14989,.F.) ;
#20539=ORIENTED_EDGE('',*,*,#15597,.T.) ;
#20540=ORIENTED_EDGE('',*,*,#15273,.F.) ;
#20541=ORIENTED_EDGE('',*,*,#15588,.T.) ;
#20542=ORIENTED_EDGE('',*,*,#14902,.F.) ;
#20543=ORIENTED_EDGE('',*,*,#15604,.T.) ;
#20544=ORIENTED_EDGE('',*,*,#15154,.F.) ;
#20545=ORIENTED_EDGE('',*,*,#15591,.T.) ;
#20546=ORIENTED_EDGE('',*,*,#15293,.F.) ;
#20547=ORIENTED_EDGE('',*,*,#15605,.T.) ;
#20548=ORIENTED_EDGE('',*,*,#15024,.F.) ;
#20549=ORIENTED_EDGE('',*,*,#15586,.F.) ;
#20550=ORIENTED_EDGE('',*,*,#15168,.F.) ;
#20551=ORIENTED_EDGE('',*,*,#15606,.F.) ;
#20552=ORIENTED_EDGE('',*,*,#14888,.F.) ;
#20553=ORIENTED_EDGE('',*,*,#15584,.F.) ;
#20554=ORIENTED_EDGE('',*,*,#15278,.F.) ;
#20555=ORIENTED_EDGE('',*,*,#15585,.F.) ;
#20556=ORIENTED_EDGE('',*,*,#15012,.F.) ;
#20557=ORIENTED_EDGE('',*,*,#15582,.F.) ;
#20558=ORIENTED_EDGE('',*,*,#15305,.F.) ;
#20559=ORIENTED_EDGE('',*,*,#15607,.F.) ;
#20560=ORIENTED_EDGE('',*,*,#15008,.F.) ;
#20561=ORIENTED_EDGE('',*,*,#15608,.F.) ;
#20562=ORIENTED_EDGE('',*,*,#14889,.F.) ;
#20563=ORIENTED_EDGE('',*,*,#15606,.T.) ;
#20564=ORIENTED_EDGE('',*,*,#15167,.F.) ;
#20565=ORIENTED_EDGE('',*,*,#15609,.F.) ;
#20566=ORIENTED_EDGE('',*,*,#15033,.F.) ;
#20567=ORIENTED_EDGE('',*,*,#15610,.F.) ;
#20568=ORIENTED_EDGE('',*,*,#15285,.F.) ;
#20569=ORIENTED_EDGE('',*,*,#15611,.F.) ;
#20570=ORIENTED_EDGE('',*,*,#15133,.F.) ;
#20571=ORIENTED_EDGE('',*,*,#15612,.F.) ;
#20572=ORIENTED_EDGE('',*,*,#14923,.F.) ;
#20573=ORIENTED_EDGE('',*,*,#15613,.F.) ;
#20574=ORIENTED_EDGE('',*,*,#15037,.F.) ;
#20575=ORIENTED_EDGE('',*,*,#15614,.F.) ;
#20576=ORIENTED_EDGE('',*,*,#15288,.F.) ;
#20577=ORIENTED_EDGE('',*,*,#15595,.T.) ;
#20578=ORIENTED_EDGE('',*,*,#15022,.F.) ;
#20579=ORIENTED_EDGE('',*,*,#15615,.F.) ;
#20580=ORIENTED_EDGE('',*,*,#15299,.F.) ;
#20581=ORIENTED_EDGE('',*,*,#15616,.F.) ;
#20582=ORIENTED_EDGE('',*,*,#14924,.F.) ;
#20583=ORIENTED_EDGE('',*,*,#15612,.T.) ;
#20584=ORIENTED_EDGE('',*,*,#15132,.F.) ;
#20585=ORIENTED_EDGE('',*,*,#15580,.T.) ;
#20586=ORIENTED_EDGE('',*,*,#15005,.F.) ;
#20587=ORIENTED_EDGE('',*,*,#15600,.T.) ;
#20588=ORIENTED_EDGE('',*,*,#15308,.F.) ;
#20589=ORIENTED_EDGE('',*,*,#15613,.T.) ;
#20590=ORIENTED_EDGE('',*,*,#15291,.F.) ;
#20591=ORIENTED_EDGE('',*,*,#15617,.F.) ;
#20592=ORIENTED_EDGE('',*,*,#15034,.F.) ;
#20593=ORIENTED_EDGE('',*,*,#14800,.T.) ;
#20594=ORIENTED_EDGE('',*,*,#14940,.F.) ;
#20595=ORIENTED_EDGE('',*,*,#14845,.T.) ;
#20596=ORIENTED_EDGE('',*,*,#15219,.F.) ;
#20597=ORIENTED_EDGE('',*,*,#15611,.T.) ;
#20598=ORIENTED_EDGE('',*,*,#14922,.F.) ;
#20599=ORIENTED_EDGE('',*,*,#15618,.T.) ;
#20600=ORIENTED_EDGE('',*,*,#15134,.F.) ;
#20601=ORIENTED_EDGE('',*,*,#15571,.T.) ;
#20602=ORIENTED_EDGE('',*,*,#14925,.F.) ;
#20603=ORIENTED_EDGE('',*,*,#15616,.T.) ;
#20604=ORIENTED_EDGE('',*,*,#15131,.F.) ;
#20605=ORIENTED_EDGE('',*,*,#15578,.T.) ;
#20606=ORIENTED_EDGE('',*,*,#15009,.F.) ;
#20607=ORIENTED_EDGE('',*,*,#15607,.T.) ;
#20608=ORIENTED_EDGE('',*,*,#15304,.F.) ;
#20609=ORIENTED_EDGE('',*,*,#15609,.T.) ;
#20610=ORIENTED_EDGE('',*,*,#15287,.F.) ;
#20611=ORIENTED_EDGE('',*,*,#15619,.F.) ;
#20612=ORIENTED_EDGE('',*,*,#15031,.F.) ;
#20613=ORIENTED_EDGE('',*,*,#15608,.T.) ;
#20614=ORIENTED_EDGE('',*,*,#15166,.F.) ;
#20615=ORIENTED_EDGE('',*,*,#15620,.T.) ;
#20616=ORIENTED_EDGE('',*,*,#14890,.F.) ;
#20617=ORIENTED_EDGE('',*,*,#15610,.T.) ;
#20618=ORIENTED_EDGE('',*,*,#15032,.F.) ;
#20619=ORIENTED_EDGE('',*,*,#15619,.T.) ;
#20620=ORIENTED_EDGE('',*,*,#15286,.F.) ;
#20621=ORIENTED_EDGE('',*,*,#15602,.F.) ;
#20622=ORIENTED_EDGE('',*,*,#15187,.F.) ;
#20623=ORIENTED_EDGE('',*,*,#15621,.F.) ;
#20624=ORIENTED_EDGE('',*,*,#14869,.F.) ;
#20625=ORIENTED_EDGE('',*,*,#15615,.T.) ;
#20626=ORIENTED_EDGE('',*,*,#15021,.F.) ;
#20627=ORIENTED_EDGE('',*,*,#15601,.F.) ;
#20628=ORIENTED_EDGE('',*,*,#15300,.F.) ;
#20629=ORIENTED_EDGE('',*,*,#15622,.F.) ;
#20630=ORIENTED_EDGE('',*,*,#15156,.F.) ;
#20631=ORIENTED_EDGE('',*,*,#15623,.F.) ;
#20632=ORIENTED_EDGE('',*,*,#14900,.F.) ;
#20633=ORIENTED_EDGE('',*,*,#15425,.F.) ;
#20634=ORIENTED_EDGE('',*,*,#14870,.F.) ;
#20635=ORIENTED_EDGE('',*,*,#15621,.T.) ;
#20636=ORIENTED_EDGE('',*,*,#15186,.F.) ;
#20637=ORIENTED_EDGE('',*,*,#15624,.F.) ;
#20638=ORIENTED_EDGE('',*,*,#15284,.F.) ;
#20639=ORIENTED_EDGE('',*,*,#15625,.F.) ;
#20640=ORIENTED_EDGE('',*,*,#15026,.F.) ;
#20641=ORIENTED_EDGE('',*,*,#15604,.F.) ;
#20642=ORIENTED_EDGE('',*,*,#14901,.F.) ;
#20643=ORIENTED_EDGE('',*,*,#15623,.T.) ;
#20644=ORIENTED_EDGE('',*,*,#15155,.F.) ;
#20645=ORIENTED_EDGE('',*,*,#15626,.F.) ;
#20646=ORIENTED_EDGE('',*,*,#15017,.F.) ;
#20647=ORIENTED_EDGE('',*,*,#15603,.F.) ;
#20648=ORIENTED_EDGE('',*,*,#15296,.F.) ;
#20649=ORIENTED_EDGE('',*,*,#15592,.T.) ;
#20650=ORIENTED_EDGE('',*,*,#15018,.F.) ;
#20651=ORIENTED_EDGE('',*,*,#15626,.T.) ;
#20652=ORIENTED_EDGE('',*,*,#15295,.F.) ;
#20653=ORIENTED_EDGE('',*,*,#15617,.T.) ;
#20654=ORIENTED_EDGE('',*,*,#15290,.F.) ;
#20655=ORIENTED_EDGE('',*,*,#15627,.F.) ;
#20656=ORIENTED_EDGE('',*,*,#15035,.F.) ;
#20657=ORIENTED_EDGE('',*,*,#15392,.T.) ;
#20658=ORIENTED_EDGE('',*,*,#14982,.F.) ;
#20659=ORIENTED_EDGE('',*,*,#15478,.T.) ;
#20660=ORIENTED_EDGE('',*,*,#15225,.F.) ;
#20661=ORIENTED_EDGE('',*,*,#15625,.T.) ;
#20662=ORIENTED_EDGE('',*,*,#15283,.F.) ;
#20663=ORIENTED_EDGE('',*,*,#15628,.F.) ;
#20664=ORIENTED_EDGE('',*,*,#15027,.F.) ;
#20665=ORIENTED_EDGE('',*,*,#15622,.T.) ;
#20666=ORIENTED_EDGE('',*,*,#14899,.F.) ;
#20667=ORIENTED_EDGE('',*,*,#15629,.T.) ;
#20668=ORIENTED_EDGE('',*,*,#15157,.F.) ;
#20669=ORIENTED_EDGE('',*,*,#15620,.F.) ;
#20670=ORIENTED_EDGE('',*,*,#15165,.F.) ;
#20671=ORIENTED_EDGE('',*,*,#15630,.F.) ;
#20672=ORIENTED_EDGE('',*,*,#14891,.F.) ;
#20673=ORIENTED_EDGE('',*,*,#15389,.F.) ;
#20674=ORIENTED_EDGE('',*,*,#15136,.F.) ;
#20675=ORIENTED_EDGE('',*,*,#15631,.F.) ;
#20676=ORIENTED_EDGE('',*,*,#14920,.F.) ;
#20677=ORIENTED_EDGE('',*,*,#15632,.F.) ;
#20678=ORIENTED_EDGE('',*,*,#14892,.F.) ;
#20679=ORIENTED_EDGE('',*,*,#15630,.T.) ;
#20680=ORIENTED_EDGE('',*,*,#15164,.F.) ;
#20681=ORIENTED_EDGE('',*,*,#15624,.T.) ;
#20682=ORIENTED_EDGE('',*,*,#15030,.F.) ;
#20683=ORIENTED_EDGE('',*,*,#15633,.F.) ;
#20684=ORIENTED_EDGE('',*,*,#15280,.F.) ;
#20685=ORIENTED_EDGE('',*,*,#15618,.F.) ;
#20686=ORIENTED_EDGE('',*,*,#14921,.F.) ;
#20687=ORIENTED_EDGE('',*,*,#15631,.T.) ;
#20688=ORIENTED_EDGE('',*,*,#15135,.F.) ;
#20689=ORIENTED_EDGE('',*,*,#15633,.T.) ;
#20690=ORIENTED_EDGE('',*,*,#15029,.F.) ;
#20691=ORIENTED_EDGE('',*,*,#15634,.F.) ;
#20692=ORIENTED_EDGE('',*,*,#15281,.F.) ;
#20693=ORIENTED_EDGE('',*,*,#15614,.T.) ;
#20694=ORIENTED_EDGE('',*,*,#15036,.F.) ;
#20695=ORIENTED_EDGE('',*,*,#15627,.T.) ;
#20696=ORIENTED_EDGE('',*,*,#15289,.F.) ;
#20697=ORIENTED_EDGE('',*,*,#15632,.T.) ;
#20698=ORIENTED_EDGE('',*,*,#15163,.F.) ;
#20699=ORIENTED_EDGE('',*,*,#15635,.T.) ;
#20700=ORIENTED_EDGE('',*,*,#14893,.F.) ;
#20701=ORIENTED_EDGE('',*,*,#15426,.F.) ;
#20702=ORIENTED_EDGE('',*,*,#15181,.F.) ;
#20703=ORIENTED_EDGE('',*,*,#15636,.F.) ;
#20704=ORIENTED_EDGE('',*,*,#14875,.F.) ;
#20705=ORIENTED_EDGE('',*,*,#15479,.F.) ;
#20706=ORIENTED_EDGE('',*,*,#14876,.F.) ;
#20707=ORIENTED_EDGE('',*,*,#15636,.T.) ;
#20708=ORIENTED_EDGE('',*,*,#15180,.F.) ;
#20709=ORIENTED_EDGE('',*,*,#15524,.T.) ;
#20710=ORIENTED_EDGE('',*,*,#15040,.F.) ;
#20711=ORIENTED_EDGE('',*,*,#15537,.F.) ;
#20712=ORIENTED_EDGE('',*,*,#15245,.F.) ;
#20713=ORIENTED_EDGE('',*,*,#15635,.F.) ;
#20714=ORIENTED_EDGE('',*,*,#15162,.F.) ;
#20715=ORIENTED_EDGE('',*,*,#15637,.F.) ;
#20716=ORIENTED_EDGE('',*,*,#14894,.F.) ;
#20717=ORIENTED_EDGE('',*,*,#15638,.F.) ;
#20718=ORIENTED_EDGE('',*,*,#14895,.F.) ;
#20719=ORIENTED_EDGE('',*,*,#15637,.T.) ;
#20720=ORIENTED_EDGE('',*,*,#15161,.F.) ;
#20721=ORIENTED_EDGE('',*,*,#15638,.T.) ;
#20722=ORIENTED_EDGE('',*,*,#15160,.F.) ;
#20723=ORIENTED_EDGE('',*,*,#15639,.T.) ;
#20724=ORIENTED_EDGE('',*,*,#14896,.F.) ;
#20725=ORIENTED_EDGE('',*,*,#15634,.T.) ;
#20726=ORIENTED_EDGE('',*,*,#15028,.F.) ;
#20727=ORIENTED_EDGE('',*,*,#15628,.T.) ;
#20728=ORIENTED_EDGE('',*,*,#15282,.F.) ;
#20729=ORIENTED_EDGE('',*,*,#15432,.T.) ;
#20730=ORIENTED_EDGE('',*,*,#15117,.F.) ;
#20731=ORIENTED_EDGE('',*,*,#15121,.F.) ;
#20732=ORIENTED_EDGE('',*,*,#15222,.F.) ;
#20733=ORIENTED_EDGE('',*,*,#15639,.F.) ;
#20734=ORIENTED_EDGE('',*,*,#15159,.F.) ;
#20735=ORIENTED_EDGE('',*,*,#15640,.F.) ;
#20736=ORIENTED_EDGE('',*,*,#14897,.F.) ;
#20737=ORIENTED_EDGE('',*,*,#15454,.F.) ;
#20738=ORIENTED_EDGE('',*,*,#15140,.F.) ;
#20739=ORIENTED_EDGE('',*,*,#15641,.F.) ;
#20740=ORIENTED_EDGE('',*,*,#14916,.F.) ;
#20741=ORIENTED_EDGE('',*,*,#15629,.F.) ;
#20742=ORIENTED_EDGE('',*,*,#14898,.F.) ;
#20743=ORIENTED_EDGE('',*,*,#15640,.T.) ;
#20744=ORIENTED_EDGE('',*,*,#15158,.F.) ;
#20745=ORIENTED_EDGE('',*,*,#15590,.T.) ;
#20746=ORIENTED_EDGE('',*,*,#15025,.F.) ;
#20747=ORIENTED_EDGE('',*,*,#15605,.F.) ;
#20748=ORIENTED_EDGE('',*,*,#15292,.F.) ;
#20749=ORIENTED_EDGE('',*,*,#15388,.F.) ;
#20750=ORIENTED_EDGE('',*,*,#14917,.F.) ;
#20751=ORIENTED_EDGE('',*,*,#15641,.T.) ;
#20752=ORIENTED_EDGE('',*,*,#15139,.F.) ;
#26659=CYLINDRICAL_SURFACE('',#29354,51.5) ;
#26660=CYLINDRICAL_SURFACE('',#29357,51.5) ;
#26661=CYLINDRICAL_SURFACE('',#29360,50.5) ;
#26662=CYLINDRICAL_SURFACE('',#29417,50.5) ;
#26663=CYLINDRICAL_SURFACE('',#29464,51.5) ;
#26664=CYLINDRICAL_SURFACE('',#29465,51.5) ;
#26665=CYLINDRICAL_SURFACE('',#29483,50.5) ;
#26666=CYLINDRICAL_SURFACE('',#29484,51.5) ;
#26667=CYLINDRICAL_SURFACE('',#29490,50.5) ;
#26668=CYLINDRICAL_SURFACE('',#29491,51.5) ;
#26669=CYLINDRICAL_SURFACE('',#29492,51.5) ;
#26670=CYLINDRICAL_SURFACE('',#29510,51.5) ;
#26671=CYLINDRICAL_SURFACE('',#29519,51.5) ;
#26672=CYLINDRICAL_SURFACE('',#29539,50.5) ;
#26673=CYLINDRICAL_SURFACE('',#29540,51.5) ;
#26674=CYLINDRICAL_SURFACE('',#29542,51.5) ;
#26675=CYLINDRICAL_SURFACE('',#29543,51.5) ;
#26676=CYLINDRICAL_SURFACE('',#29566,51.5) ;
#26677=CYLINDRICAL_SURFACE('',#29567,51.5) ;
#26678=CYLINDRICAL_SURFACE('',#29568,50.5) ;
#26679=CYLINDRICAL_SURFACE('',#29569,50.5) ;
#26680=CYLINDRICAL_SURFACE('',#29594,50.5) ;
#26681=CYLINDRICAL_SURFACE('',#29595,50.5) ;
#26682=CYLINDRICAL_SURFACE('',#29596,51.5) ;
#26683=CYLINDRICAL_SURFACE('',#29603,50.5) ;
#26684=CYLINDRICAL_SURFACE('',#29604,51.5) ;
#26685=CYLINDRICAL_SURFACE('',#29623,50.5) ;
#26686=CYLINDRICAL_SURFACE('',#29624,51.5) ;
#26687=CYLINDRICAL_SURFACE('',#29627,51.5) ;
#26688=CYLINDRICAL_SURFACE('',#29628,51.5) ;
#26689=CYLINDRICAL_SURFACE('',#29629,50.5) ;
#26690=CYLINDRICAL_SURFACE('',#29652,50.5) ;
#26691=CYLINDRICAL_SURFACE('',#29655,50.5) ;
#26692=CYLINDRICAL_SURFACE('',#29656,50.5) ;
#26693=CYLINDRICAL_SURFACE('',#29657,51.5) ;
#26694=CYLINDRICAL_SURFACE('',#29674,51.5) ;
#26695=CYLINDRICAL_SURFACE('',#29677,51.5) ;
#26696=CYLINDRICAL_SURFACE('',#29678,50.5) ;
#26697=CYLINDRICAL_SURFACE('',#29690,50.5) ;
#26698=CYLINDRICAL_SURFACE('',#29691,51.5) ;
#26699=CYLINDRICAL_SURFACE('',#29692,51.5) ;
#26700=CYLINDRICAL_SURFACE('',#29695,51.5) ;
#26701=CYLINDRICAL_SURFACE('',#29696,50.5) ;
#26702=CYLINDRICAL_SURFACE('',#29706,50.5) ;
#26703=CYLINDRICAL_SURFACE('',#29708,51.5) ;
#26704=CYLINDRICAL_SURFACE('',#29716,51.5) ;
#26705=CYLINDRICAL_SURFACE('',#29722,51.5) ;
#26706=CYLINDRICAL_SURFACE('',#29723,50.5) ;
#27160=ADVANCED_FACE('',(#2425),#1483,.F.) ;
#27161=ADVANCED_FACE('',(#2426),#1484,.F.) ;
#27162=ADVANCED_FACE('',(#2427),#1485,.F.) ;
#27163=ADVANCED_FACE('',(#2428),#1486,.F.) ;
#27164=ADVANCED_FACE('',(#2429),#1487,.F.) ;
#27165=ADVANCED_FACE('',(#2430),#1488,.F.) ;
#27166=ADVANCED_FACE('',(#2431),#1489,.F.) ;
#27167=ADVANCED_FACE('',(#2432),#1490,.F.) ;
#27168=ADVANCED_FACE('',(#2433),#1491,.F.) ;
#27169=ADVANCED_FACE('',(#2434),#1492,.F.) ;
#27170=ADVANCED_FACE('',(#2435),#1493,.F.) ;
#27171=ADVANCED_FACE('',(#2436),#1494,.F.) ;
#27172=ADVANCED_FACE('',(#2437),#1495,.F.) ;
#27173=ADVANCED_FACE('',(#2438),#1496,.F.) ;
#27174=ADVANCED_FACE('',(#2439),#26659,.T.) ;
#27175=ADVANCED_FACE('',(#2440),#26660,.T.) ;
#27176=ADVANCED_FACE('',(#2441),#26661,.F.) ;
#27177=ADVANCED_FACE('',(#2442),#1497,.F.) ;
#27178=ADVANCED_FACE('',(#2443),#1498,.F.) ;
#27179=ADVANCED_FACE('',(#2444),#1499,.F.) ;
#27180=ADVANCED_FACE('',(#2445),#1500,.F.) ;
#27181=ADVANCED_FACE('',(#2446),#1501,.F.) ;
#27182=ADVANCED_FACE('',(#2447),#1502,.F.) ;
#27183=ADVANCED_FACE('',(#2448),#1503,.F.) ;
#27184=ADVANCED_FACE('',(#2449),#1504,.F.) ;
#27185=ADVANCED_FACE('',(#2450,#1130,#1131,#1132,#1133,#1134,#1135,#1136,
#1137,#1138,#1139,#1140,#1141,#1142,#1143,#1144,#1145,#1146,#1147,#1148,
#1149,#1150,#1151,#1152,#1153,#1154,#1155,#1156,#1157,#1158,#1159,#1160,
#1161,#1162,#1163,#1164,#1165,#1166,#1167,#1168,#1169,#1170,#1171,#1172,
#1173,#1174,#1175,#1176,#1177,#1178,#1179,#1180,#1181),#1505,.T.) ;
#27186=ADVANCED_FACE('',(#2451),#26662,.F.) ;
#27187=ADVANCED_FACE('',(#2452,#1182,#1183,#1184,#1185,#1186,#1187,#1188,
#1189,#1190,#1191,#1192,#1193,#1194,#1195,#1196,#1197,#1198,#1199,#1200,
#1201,#1202,#1203,#1204,#1205,#1206,#1207,#1208,#1209,#1210,#1211,#1212,
#1213,#1214,#1215,#1216,#1217,#1218,#1219,#1220,#1221,#1222,#1223,#1224,
#1225,#1226,#1227,#1228,#1229,#1230,#1231,#1232,#1233),#1506,.T.) ;
#27188=ADVANCED_FACE('',(#2453),#26663,.T.) ;
#27189=ADVANCED_FACE('',(#2454),#26664,.T.) ;
#27190=ADVANCED_FACE('',(#2455),#1507,.F.) ;
#27191=ADVANCED_FACE('',(#2456),#1508,.F.) ;
#27192=ADVANCED_FACE('',(#2457),#1509,.F.) ;
#27193=ADVANCED_FACE('',(#2458),#1510,.F.) ;
#27194=ADVANCED_FACE('',(#2459),#1511,.F.) ;
#27195=ADVANCED_FACE('',(#2460),#1512,.F.) ;
#27196=ADVANCED_FACE('',(#2461),#1513,.F.) ;
#27197=ADVANCED_FACE('',(#2462),#1514,.F.) ;
#27198=ADVANCED_FACE('',(#2463),#1515,.F.) ;
#27199=ADVANCED_FACE('',(#2464),#1516,.F.) ;
#27200=ADVANCED_FACE('',(#2465),#1517,.F.) ;
#27201=ADVANCED_FACE('',(#2466),#1518,.F.) ;
#27202=ADVANCED_FACE('',(#2467),#1519,.F.) ;
#27203=ADVANCED_FACE('',(#2468),#1520,.F.) ;
#27204=ADVANCED_FACE('',(#2469),#1521,.F.) ;
#27205=ADVANCED_FACE('',(#2470),#1522,.F.) ;
#27206=ADVANCED_FACE('',(#2471),#1523,.F.) ;
#27207=ADVANCED_FACE('',(#2472),#26665,.F.) ;
#27208=ADVANCED_FACE('',(#2473),#26666,.T.) ;
#27209=ADVANCED_FACE('',(#2474),#1524,.F.) ;
#27210=ADVANCED_FACE('',(#2475),#1525,.F.) ;
#27211=ADVANCED_FACE('',(#2476),#1526,.F.) ;
#27212=ADVANCED_FACE('',(#2477),#1527,.F.) ;
#27213=ADVANCED_FACE('',(#2478),#1528,.F.) ;
#27214=ADVANCED_FACE('',(#2479),#26667,.F.) ;
#27215=ADVANCED_FACE('',(#2480),#26668,.T.) ;
#27216=ADVANCED_FACE('',(#2481),#26669,.T.) ;
#27217=ADVANCED_FACE('',(#2482),#1529,.F.) ;
#27218=ADVANCED_FACE('',(#2483),#1530,.F.) ;
#27219=ADVANCED_FACE('',(#2484),#1531,.F.) ;
#27220=ADVANCED_FACE('',(#2485),#1532,.F.) ;
#27221=ADVANCED_FACE('',(#2486),#1533,.F.) ;
#27222=ADVANCED_FACE('',(#2487),#1534,.F.) ;
#27223=ADVANCED_FACE('',(#2488),#1535,.F.) ;
#27224=ADVANCED_FACE('',(#2489),#1536,.F.) ;
#27225=ADVANCED_FACE('',(#2490),#1537,.F.) ;
#27226=ADVANCED_FACE('',(#2491),#1538,.F.) ;
#27227=ADVANCED_FACE('',(#2492),#1539,.F.) ;
#27228=ADVANCED_FACE('',(#2493),#1540,.F.) ;
#27229=ADVANCED_FACE('',(#2494),#1541,.F.) ;
#27230=ADVANCED_FACE('',(#2495),#1542,.F.) ;
#27231=ADVANCED_FACE('',(#2496),#1543,.F.) ;
#27232=ADVANCED_FACE('',(#2497),#1544,.F.) ;
#27233=ADVANCED_FACE('',(#2498),#1545,.F.) ;
#27234=ADVANCED_FACE('',(#2499),#26670,.T.) ;
#27235=ADVANCED_FACE('',(#2500),#1546,.F.) ;
#27236=ADVANCED_FACE('',(#2501),#1547,.F.) ;
#27237=ADVANCED_FACE('',(#2502),#1548,.F.) ;
#27238=ADVANCED_FACE('',(#2503),#1549,.F.) ;
#27239=ADVANCED_FACE('',(#2504),#1550,.F.) ;
#27240=ADVANCED_FACE('',(#2505),#1551,.F.) ;
#27241=ADVANCED_FACE('',(#2506),#1552,.F.) ;
#27242=ADVANCED_FACE('',(#2507),#1553,.F.) ;
#27243=ADVANCED_FACE('',(#2508),#26671,.T.) ;
#27244=ADVANCED_FACE('',(#2509),#1554,.F.) ;
#27245=ADVANCED_FACE('',(#2510),#1555,.F.) ;
#27246=ADVANCED_FACE('',(#2511),#1556,.F.) ;
#27247=ADVANCED_FACE('',(#2512),#1557,.F.) ;
#27248=ADVANCED_FACE('',(#2513),#1558,.F.) ;
#27249=ADVANCED_FACE('',(#2514),#1559,.F.) ;
#27250=ADVANCED_FACE('',(#2515),#1560,.F.) ;
#27251=ADVANCED_FACE('',(#2516),#1561,.F.) ;
#27252=ADVANCED_FACE('',(#2517),#1562,.F.) ;
#27253=ADVANCED_FACE('',(#2518),#1563,.F.) ;
#27254=ADVANCED_FACE('',(#2519),#1564,.F.) ;
#27255=ADVANCED_FACE('',(#2520),#1565,.F.) ;
#27256=ADVANCED_FACE('',(#2521),#1566,.F.) ;
#27257=ADVANCED_FACE('',(#2522),#1567,.F.) ;
#27258=ADVANCED_FACE('',(#2523),#1568,.F.) ;
#27259=ADVANCED_FACE('',(#2524),#1569,.F.) ;
#27260=ADVANCED_FACE('',(#2525),#1570,.F.) ;
#27261=ADVANCED_FACE('',(#2526),#1571,.F.) ;
#27262=ADVANCED_FACE('',(#2527),#1572,.F.) ;
#27263=ADVANCED_FACE('',(#2528),#26672,.F.) ;
#27264=ADVANCED_FACE('',(#2529),#26673,.T.) ;
#27265=ADVANCED_FACE('',(#2530),#1573,.F.) ;
#27266=ADVANCED_FACE('',(#2531),#26674,.T.) ;
#27267=ADVANCED_FACE('',(#2532),#26675,.T.) ;
#27268=ADVANCED_FACE('',(#2533),#1574,.F.) ;
#27269=ADVANCED_FACE('',(#2534),#1575,.F.) ;
#27270=ADVANCED_FACE('',(#2535),#1576,.F.) ;
#27271=ADVANCED_FACE('',(#2536),#1577,.F.) ;
#27272=ADVANCED_FACE('',(#2537),#1578,.F.) ;
#27273=ADVANCED_FACE('',(#2538),#1579,.F.) ;
#27274=ADVANCED_FACE('',(#2539),#1580,.F.) ;
#27275=ADVANCED_FACE('',(#2540),#1581,.F.) ;
#27276=ADVANCED_FACE('',(#2541),#1582,.F.) ;
#27277=ADVANCED_FACE('',(#2542),#1583,.F.) ;
#27278=ADVANCED_FACE('',(#2543),#1584,.F.) ;
#27279=ADVANCED_FACE('',(#2544),#1585,.F.) ;
#27280=ADVANCED_FACE('',(#2545),#1586,.F.) ;
#27281=ADVANCED_FACE('',(#2546),#1587,.F.) ;
#27282=ADVANCED_FACE('',(#2547),#1588,.F.) ;
#27283=ADVANCED_FACE('',(#2548),#1589,.F.) ;
#27284=ADVANCED_FACE('',(#2549),#1590,.F.) ;
#27285=ADVANCED_FACE('',(#2550),#1591,.F.) ;
#27286=ADVANCED_FACE('',(#2551),#1592,.F.) ;
#27287=ADVANCED_FACE('',(#2552),#1593,.F.) ;
#27288=ADVANCED_FACE('',(#2553),#1594,.F.) ;
#27289=ADVANCED_FACE('',(#2554),#1595,.F.) ;
#27290=ADVANCED_FACE('',(#2555),#26676,.T.) ;
#27291=ADVANCED_FACE('',(#2556),#26677,.T.) ;
#27292=ADVANCED_FACE('',(#2557),#26678,.F.) ;
#27293=ADVANCED_FACE('',(#2558),#26679,.F.) ;
#27294=ADVANCED_FACE('',(#2559),#1596,.F.) ;
#27295=ADVANCED_FACE('',(#2560),#1597,.F.) ;
#27296=ADVANCED_FACE('',(#2561),#1598,.F.) ;
#27297=ADVANCED_FACE('',(#2562),#1599,.F.) ;
#27298=ADVANCED_FACE('',(#2563),#1600,.F.) ;
#27299=ADVANCED_FACE('',(#2564),#1601,.F.) ;
#27300=ADVANCED_FACE('',(#2565),#1602,.F.) ;
#27301=ADVANCED_FACE('',(#2566),#1603,.F.) ;
#27302=ADVANCED_FACE('',(#2567),#1604,.F.) ;
#27303=ADVANCED_FACE('',(#2568),#1605,.F.) ;
#27304=ADVANCED_FACE('',(#2569),#1606,.F.) ;
#27305=ADVANCED_FACE('',(#2570),#1607,.F.) ;
#27306=ADVANCED_FACE('',(#2571),#1608,.F.) ;
#27307=ADVANCED_FACE('',(#2572),#1609,.F.) ;
#27308=ADVANCED_FACE('',(#2573),#1610,.F.) ;
#27309=ADVANCED_FACE('',(#2574),#1611,.F.) ;
#27310=ADVANCED_FACE('',(#2575),#1612,.F.) ;
#27311=ADVANCED_FACE('',(#2576),#1613,.F.) ;
#27312=ADVANCED_FACE('',(#2577),#1614,.F.) ;
#27313=ADVANCED_FACE('',(#2578),#1615,.F.) ;
#27314=ADVANCED_FACE('',(#2579),#1616,.F.) ;
#27315=ADVANCED_FACE('',(#2580),#1617,.F.) ;
#27316=ADVANCED_FACE('',(#2581),#1618,.F.) ;
#27317=ADVANCED_FACE('',(#2582),#1619,.F.) ;
#27318=ADVANCED_FACE('',(#2583),#26680,.F.) ;
#27319=ADVANCED_FACE('',(#2584),#26681,.F.) ;
#27320=ADVANCED_FACE('',(#2585),#26682,.T.) ;
#27321=ADVANCED_FACE('',(#2586),#1620,.F.) ;
#27322=ADVANCED_FACE('',(#2587),#1621,.F.) ;
#27323=ADVANCED_FACE('',(#2588),#1622,.F.) ;
#27324=ADVANCED_FACE('',(#2589),#1623,.F.) ;
#27325=ADVANCED_FACE('',(#2590),#1624,.F.) ;
#27326=ADVANCED_FACE('',(#2591),#1625,.F.) ;
#27327=ADVANCED_FACE('',(#2592),#26683,.F.) ;
#27328=ADVANCED_FACE('',(#2593),#26684,.T.) ;
#27329=ADVANCED_FACE('',(#2594),#1626,.F.) ;
#27330=ADVANCED_FACE('',(#2595),#1627,.F.) ;
#27331=ADVANCED_FACE('',(#2596),#1628,.F.) ;
#27332=ADVANCED_FACE('',(#2597),#1629,.F.) ;
#27333=ADVANCED_FACE('',(#2598),#1630,.F.) ;
#27334=ADVANCED_FACE('',(#2599),#1631,.F.) ;
#27335=ADVANCED_FACE('',(#2600),#1632,.F.) ;
#27336=ADVANCED_FACE('',(#2601),#1633,.F.) ;
#27337=ADVANCED_FACE('',(#2602),#1634,.F.) ;
#27338=ADVANCED_FACE('',(#2603),#1635,.F.) ;
#27339=ADVANCED_FACE('',(#2604),#1636,.F.) ;
#27340=ADVANCED_FACE('',(#2605),#1637,.F.) ;
#27341=ADVANCED_FACE('',(#2606),#1638,.F.) ;
#27342=ADVANCED_FACE('',(#2607),#1639,.F.) ;
#27343=ADVANCED_FACE('',(#2608),#1640,.F.) ;
#27344=ADVANCED_FACE('',(#2609),#1641,.F.) ;
#27345=ADVANCED_FACE('',(#2610),#1642,.F.) ;
#27346=ADVANCED_FACE('',(#2611),#1643,.F.) ;
#27347=ADVANCED_FACE('',(#2612),#26685,.F.) ;
#27348=ADVANCED_FACE('',(#2613),#26686,.T.) ;
#27349=ADVANCED_FACE('',(#2614),#1644,.F.) ;
#27350=ADVANCED_FACE('',(#2615),#1645,.F.) ;
#27351=ADVANCED_FACE('',(#2616),#26687,.T.) ;
#27352=ADVANCED_FACE('',(#2617),#26688,.T.) ;
#27353=ADVANCED_FACE('',(#2618),#26689,.F.) ;
#27354=ADVANCED_FACE('',(#2619),#1646,.F.) ;
#27355=ADVANCED_FACE('',(#2620),#1647,.F.) ;
#27356=ADVANCED_FACE('',(#2621),#1648,.F.) ;
#27357=ADVANCED_FACE('',(#2622),#1649,.F.) ;
#27358=ADVANCED_FACE('',(#2623),#1650,.F.) ;
#27359=ADVANCED_FACE('',(#2624),#1651,.F.) ;
#27360=ADVANCED_FACE('',(#2625),#1652,.F.) ;
#27361=ADVANCED_FACE('',(#2626),#1653,.F.) ;
#27362=ADVANCED_FACE('',(#2627),#1654,.F.) ;
#27363=ADVANCED_FACE('',(#2628),#1655,.F.) ;
#27364=ADVANCED_FACE('',(#2629),#1656,.F.) ;
#27365=ADVANCED_FACE('',(#2630),#1657,.F.) ;
#27366=ADVANCED_FACE('',(#2631),#1658,.F.) ;
#27367=ADVANCED_FACE('',(#2632),#1659,.F.) ;
#27368=ADVANCED_FACE('',(#2633),#1660,.F.) ;
#27369=ADVANCED_FACE('',(#2634),#1661,.F.) ;
#27370=ADVANCED_FACE('',(#2635),#1662,.F.) ;
#27371=ADVANCED_FACE('',(#2636),#1663,.F.) ;
#27372=ADVANCED_FACE('',(#2637),#1664,.F.) ;
#27373=ADVANCED_FACE('',(#2638),#1665,.F.) ;
#27374=ADVANCED_FACE('',(#2639),#1666,.F.) ;
#27375=ADVANCED_FACE('',(#2640),#1667,.F.) ;
#27376=ADVANCED_FACE('',(#2641),#26690,.F.) ;
#27377=ADVANCED_FACE('',(#2642),#1668,.F.) ;
#27378=ADVANCED_FACE('',(#2643),#1669,.F.) ;
#27379=ADVANCED_FACE('',(#2644),#26691,.F.) ;
#27380=ADVANCED_FACE('',(#2645),#26692,.F.) ;
#27381=ADVANCED_FACE('',(#2646),#26693,.T.) ;
#27382=ADVANCED_FACE('',(#2647),#1670,.F.) ;
#27383=ADVANCED_FACE('',(#2648),#1671,.F.) ;
#27384=ADVANCED_FACE('',(#2649),#1672,.F.) ;
#27385=ADVANCED_FACE('',(#2650),#1673,.F.) ;
#27386=ADVANCED_FACE('',(#2651),#1674,.F.) ;
#27387=ADVANCED_FACE('',(#2652),#1675,.F.) ;
#27388=ADVANCED_FACE('',(#2653),#1676,.F.) ;
#27389=ADVANCED_FACE('',(#2654),#1677,.F.) ;
#27390=ADVANCED_FACE('',(#2655),#1678,.F.) ;
#27391=ADVANCED_FACE('',(#2656),#1679,.F.) ;
#27392=ADVANCED_FACE('',(#2657),#1680,.F.) ;
#27393=ADVANCED_FACE('',(#2658),#1681,.F.) ;
#27394=ADVANCED_FACE('',(#2659),#1682,.F.) ;
#27395=ADVANCED_FACE('',(#2660),#1683,.F.) ;
#27396=ADVANCED_FACE('',(#2661),#1684,.F.) ;
#27397=ADVANCED_FACE('',(#2662),#1685,.F.) ;
#27398=ADVANCED_FACE('',(#2663),#26694,.T.) ;
#27399=ADVANCED_FACE('',(#2664),#1686,.F.) ;
#27400=ADVANCED_FACE('',(#2665),#1687,.F.) ;
#27401=ADVANCED_FACE('',(#2666),#26695,.T.) ;
#27402=ADVANCED_FACE('',(#2667),#26696,.F.) ;
#27403=ADVANCED_FACE('',(#2668),#1688,.F.) ;
#27404=ADVANCED_FACE('',(#2669),#1689,.F.) ;
#27405=ADVANCED_FACE('',(#2670),#1690,.F.) ;
#27406=ADVANCED_FACE('',(#2671),#1691,.F.) ;
#27407=ADVANCED_FACE('',(#2672),#1692,.F.) ;
#27408=ADVANCED_FACE('',(#2673),#1693,.F.) ;
#27409=ADVANCED_FACE('',(#2674),#1694,.F.) ;
#27410=ADVANCED_FACE('',(#2675),#1695,.F.) ;
#27411=ADVANCED_FACE('',(#2676),#1696,.F.) ;
#27412=ADVANCED_FACE('',(#2677),#1697,.F.) ;
#27413=ADVANCED_FACE('',(#2678),#1698,.F.) ;
#27414=ADVANCED_FACE('',(#2679),#26697,.F.) ;
#27415=ADVANCED_FACE('',(#2680),#26698,.T.) ;
#27416=ADVANCED_FACE('',(#2681),#26699,.T.) ;
#27417=ADVANCED_FACE('',(#2682),#1699,.F.) ;
#27418=ADVANCED_FACE('',(#2683),#1700,.F.) ;
#27419=ADVANCED_FACE('',(#2684),#26700,.T.) ;
#27420=ADVANCED_FACE('',(#2685),#26701,.F.) ;
#27421=ADVANCED_FACE('',(#2686),#1701,.F.) ;
#27422=ADVANCED_FACE('',(#2687),#1702,.F.) ;
#27423=ADVANCED_FACE('',(#2688),#1703,.F.) ;
#27424=ADVANCED_FACE('',(#2689),#1704,.F.) ;
#27425=ADVANCED_FACE('',(#2690),#1705,.F.) ;
#27426=ADVANCED_FACE('',(#2691),#1706,.F.) ;
#27427=ADVANCED_FACE('',(#2692),#1707,.F.) ;
#27428=ADVANCED_FACE('',(#2693),#1708,.F.) ;
#27429=ADVANCED_FACE('',(#2694),#1709,.F.) ;
#27430=ADVANCED_FACE('',(#2695),#26702,.F.) ;
#27431=ADVANCED_FACE('',(#2696),#1710,.F.) ;
#27432=ADVANCED_FACE('',(#2697),#26703,.T.) ;
#27433=ADVANCED_FACE('',(#2698),#1711,.F.) ;
#27434=ADVANCED_FACE('',(#2699),#1712,.F.) ;
#27435=ADVANCED_FACE('',(#2700),#1713,.F.) ;
#27436=ADVANCED_FACE('',(#2701),#1714,.F.) ;
#27437=ADVANCED_FACE('',(#2702),#1715,.F.) ;
#27438=ADVANCED_FACE('',(#2703),#1716,.F.) ;
#27439=ADVANCED_FACE('',(#2704),#1717,.F.) ;
#27440=ADVANCED_FACE('',(#2705),#26704,.T.) ;
#27441=ADVANCED_FACE('',(#2706),#1718,.F.) ;
#27442=ADVANCED_FACE('',(#2707),#1719,.F.) ;
#27443=ADVANCED_FACE('',(#2708),#1720,.F.) ;
#27444=ADVANCED_FACE('',(#2709),#1721,.F.) ;
#27445=ADVANCED_FACE('',(#2710),#1722,.F.) ;
#27446=ADVANCED_FACE('',(#2711),#26705,.T.) ;
#27447=ADVANCED_FACE('',(#2712),#26706,.F.) ;
#27448=ADVANCED_FACE('',(#2713),#1723,.F.) ;
#27449=ADVANCED_FACE('',(#2714),#1724,.F.) ;
#27450=ADVANCED_FACE('',(#2715),#1725,.F.) ;
#27451=ADVANCED_FACE('',(#2716),#1726,.F.) ;
#27452=ADVANCED_FACE('',(#2717),#1727,.F.) ;
#27453=ADVANCED_FACE('',(#2718),#1728,.F.) ;
#28632=CLOSED_SHELL('',(#27160,#27161,#27162,#27163,#27164,#27165,#27166,
#27167,#27168,#27169,#27170,#27171,#27172,#27173,#27174,#27175,#27176,#27177,
#27178,#27179,#27180,#27181,#27182,#27183,#27184,#27185,#27186,#27187,#27188,
#27189,#27190,#27191,#27192,#27193,#27194,#27195,#27196,#27197,#27198,#27199,
#27200,#27201,#27202,#27203,#27204,#27205,#27206,#27207,#27208,#27209,#27210,
#27211,#27212,#27213,#27214,#27215,#27216,#27217,#27218,#27219,#27220,#27221,
#27222,#27223,#27224,#27225,#27226,#27227,#27228,#27229,#27230,#27231,#27232,
#27233,#27234,#27235,#27236,#27237,#27238,#27239,#27240,#27241,#27242,#27243,
#27244,#27245,#27246,#27247,#27248,#27249,#27250,#27251,#27252,#27253,#27254,
#27255,#27256,#27257,#27258,#27259,#27260,#27261,#27262,#27263,#27264,#27265,
#27266,#27267,#27268,#27269,#27270,#27271,#27272,#27273,#27274,#27275,#27276,
#27277,#27278,#27279,#27280,#27281,#27282,#27283,#27284,#27285,#27286,#27287,
#27288,#27289,#27290,#27291,#27292,#27293,#27294,#27295,#27296,#27297,#27298,
#27299,#27300,#27301,#27302,#27303,#27304,#27305,#27306,#27307,#27308,#27309,
#27310,#27311,#27312,#27313,#27314,#27315,#27316,#27317,#27318,#27319,#27320,
#27321,#27322,#27323,#27324,#27325,#27326,#27327,#27328,#27329,#27330,#27331,
#27332,#27333,#27334,#27335,#27336,#27337,#27338,#27339,#27340,#27341,#27342,
#27343,#27344,#27345,#27346,#27347,#27348,#27349,#27350,#27351,#27352,#27353,
#27354,#27355,#27356,#27357,#27358,#27359,#27360,#27361,#27362,#27363,#27364,
#27365,#27366,#27367,#27368,#27369,#27370,#27371,#27372,#27373,#27374,#27375,
#27376,#27377,#27378,#27379,#27380,#27381,#27382,#27383,#27384,#27385,#27386,
#27387,#27388,#27389,#27390,#27391,#27392,#27393,#27394,#27395,#27396,#27397,
#27398,#27399,#27400,#27401,#27402,#27403,#27404,#27405,#27406,#27407,#27408,
#27409,#27410,#27411,#27412,#27413,#27414,#27415,#27416,#27417,#27418,#27419,
#27420,#27421,#27422,#27423,#27424,#27425,#27426,#27427,#27428,#27429,#27430,
#27431,#27432,#27433,#27434,#27435,#27436,#27437,#27438,#27439,#27440,#27441,
#27442,#27443,#27444,#27445,#27446,#27447,#27448,#27449,#27450,#27451,#27452,
#27453)) ;
#29339=AXIS2_PLACEMENT_3D('',#41686,#32798,#32799) ;
#29340=AXIS2_PLACEMENT_3D('',#41687,#32800,#32801) ;
#29341=AXIS2_PLACEMENT_3D('',#41696,#32806,#32807) ;
#29342=AXIS2_PLACEMENT_3D('',#41705,#32812,#32813) ;
#29343=AXIS2_PLACEMENT_3D('',#41714,#32818,#32819) ;
#29344=AXIS2_PLACEMENT_3D('',#41723,#32824,#32825) ;
#29345=AXIS2_PLACEMENT_3D('',#41732,#32830,#32831) ;
#29346=AXIS2_PLACEMENT_3D('',#41741,#32836,#32837) ;
#29347=AXIS2_PLACEMENT_3D('',#41750,#32842,#32843) ;
#29348=AXIS2_PLACEMENT_3D('',#41759,#32848,#32849) ;
#29349=AXIS2_PLACEMENT_3D('',#41768,#32854,#32855) ;
#29350=AXIS2_PLACEMENT_3D('',#41777,#32860,#32861) ;
#29351=AXIS2_PLACEMENT_3D('',#41786,#32866,#32867) ;
#29352=AXIS2_PLACEMENT_3D('',#41795,#32872,#32873) ;
#29353=AXIS2_PLACEMENT_3D('',#41801,#32877,#32878) ;
#29354=AXIS2_PLACEMENT_3D('',#41807,#32882,#32883) ;
#29355=AXIS2_PLACEMENT_3D('',#41809,#32884,#32885) ;
#29356=AXIS2_PLACEMENT_3D('',#41812,#32887,#32888) ;
#29357=AXIS2_PLACEMENT_3D('',#41813,#32889,#32890) ;
#29358=AXIS2_PLACEMENT_3D('',#41815,#32891,#32892) ;
#29359=AXIS2_PLACEMENT_3D('',#41818,#32894,#32895) ;
#29360=AXIS2_PLACEMENT_3D('',#41819,#32896,#32897) ;
#29361=AXIS2_PLACEMENT_3D('',#41821,#32898,#32899) ;
#29362=AXIS2_PLACEMENT_3D('',#41824,#32901,#32902) ;
#29363=AXIS2_PLACEMENT_3D('',#41825,#32903,#32904) ;
#29364=AXIS2_PLACEMENT_3D('',#41831,#32908,#32909) ;
#29365=AXIS2_PLACEMENT_3D('',#41837,#32913,#32914) ;
#29366=AXIS2_PLACEMENT_3D('',#41843,#32918,#32919) ;
#29367=AXIS2_PLACEMENT_3D('',#41849,#32923,#32924) ;
#29368=AXIS2_PLACEMENT_3D('',#41855,#32928,#32929) ;
#29369=AXIS2_PLACEMENT_3D('',#41861,#32933,#32934) ;
#29370=AXIS2_PLACEMENT_3D('',#41867,#32938,#32939) ;
#29371=AXIS2_PLACEMENT_3D('',#41873,#32943,#32944) ;
#29372=AXIS2_PLACEMENT_3D('',#41879,#32947,#32948) ;
#29373=AXIS2_PLACEMENT_3D('',#41885,#32951,#32952) ;
#29374=AXIS2_PLACEMENT_3D('',#41891,#32955,#32956) ;
#29375=AXIS2_PLACEMENT_3D('',#41899,#32960,#32961) ;
#29376=AXIS2_PLACEMENT_3D('',#41905,#32964,#32965) ;
#29377=AXIS2_PLACEMENT_3D('',#41911,#32968,#32969) ;
#29378=AXIS2_PLACEMENT_3D('',#41917,#32972,#32973) ;
#29379=AXIS2_PLACEMENT_3D('',#41923,#32976,#32977) ;
#29380=AXIS2_PLACEMENT_3D('',#41929,#32980,#32981) ;
#29381=AXIS2_PLACEMENT_3D('',#41935,#32984,#32985) ;
#29382=AXIS2_PLACEMENT_3D('',#41943,#32989,#32990) ;
#29383=AXIS2_PLACEMENT_3D('',#41949,#32993,#32994) ;
#29384=AXIS2_PLACEMENT_3D('',#41955,#32997,#32998) ;
#29385=AXIS2_PLACEMENT_3D('',#41961,#33001,#33002) ;
#29386=AXIS2_PLACEMENT_3D('',#41967,#33005,#33006) ;
#29387=AXIS2_PLACEMENT_3D('',#41973,#33009,#33010) ;
#29388=AXIS2_PLACEMENT_3D('',#41979,#33013,#33014) ;
#29389=AXIS2_PLACEMENT_3D('',#41987,#33018,#33019) ;
#29390=AXIS2_PLACEMENT_3D('',#41993,#33022,#33023) ;
#29391=AXIS2_PLACEMENT_3D('',#41999,#33026,#33027) ;
#29392=AXIS2_PLACEMENT_3D('',#42004,#33030,#33031) ;
#29393=AXIS2_PLACEMENT_3D('',#42006,#33032,#33033) ;
#29394=AXIS2_PLACEMENT_3D('',#42012,#33036,#33037) ;
#29395=AXIS2_PLACEMENT_3D('',#42018,#33040,#33041) ;
#29396=AXIS2_PLACEMENT_3D('',#42026,#33045,#33046) ;
#29397=AXIS2_PLACEMENT_3D('',#42032,#33049,#33050) ;
#29398=AXIS2_PLACEMENT_3D('',#42038,#33054,#33055) ;
#29399=AXIS2_PLACEMENT_3D('',#42041,#33057,#33058) ;
#29400=AXIS2_PLACEMENT_3D('',#42043,#33060,#33061) ;
#29401=AXIS2_PLACEMENT_3D('',#42060,#33072,#33073) ;
#29402=AXIS2_PLACEMENT_3D('',#42065,#33075,#33076) ;
#29403=AXIS2_PLACEMENT_3D('',#42105,#33096,#33097) ;
#29404=AXIS2_PLACEMENT_3D('',#42113,#33101,#33102) ;
#29405=AXIS2_PLACEMENT_3D('',#42123,#33107,#33108) ;
#29406=AXIS2_PLACEMENT_3D('',#42129,#33111,#33112) ;
#29407=AXIS2_PLACEMENT_3D('',#42133,#33114,#33115) ;
#29408=AXIS2_PLACEMENT_3D('',#42185,#33141,#33142) ;
#29409=AXIS2_PLACEMENT_3D('',#42207,#33153,#33154) ;
#29410=AXIS2_PLACEMENT_3D('',#42215,#33158,#33159) ;
#29411=AXIS2_PLACEMENT_3D('',#42223,#33163,#33164) ;
#29412=AXIS2_PLACEMENT_3D('',#42237,#33171,#33172) ;
#29413=AXIS2_PLACEMENT_3D('',#42245,#33176,#33177) ;
#29414=AXIS2_PLACEMENT_3D('',#42300,#33205,#33206) ;
#29415=AXIS2_PLACEMENT_3D('',#42311,#33211,#33212) ;
#29416=AXIS2_PLACEMENT_3D('',#42390,#33252,#33253) ;
#29417=AXIS2_PLACEMENT_3D('',#42396,#33257,#33258) ;
#29418=AXIS2_PLACEMENT_3D('',#42398,#33259,#33260) ;
#29419=AXIS2_PLACEMENT_3D('',#42400,#33262,#33263) ;
#29420=AXIS2_PLACEMENT_3D('',#42406,#33266,#33267) ;
#29421=AXIS2_PLACEMENT_3D('',#42412,#33270,#33271) ;
#29422=AXIS2_PLACEMENT_3D('',#42420,#33275,#33276) ;
#29423=AXIS2_PLACEMENT_3D('',#42426,#33279,#33280) ;
#29424=AXIS2_PLACEMENT_3D('',#42431,#33283,#33284) ;
#29425=AXIS2_PLACEMENT_3D('',#42433,#33285,#33286) ;
#29426=AXIS2_PLACEMENT_3D('',#42439,#33289,#33290) ;
#29427=AXIS2_PLACEMENT_3D('',#42445,#33293,#33294) ;
#29428=AXIS2_PLACEMENT_3D('',#42451,#33297,#33298) ;
#29429=AXIS2_PLACEMENT_3D('',#42459,#33302,#33303) ;
#29430=AXIS2_PLACEMENT_3D('',#42465,#33306,#33307) ;
#29431=AXIS2_PLACEMENT_3D('',#42471,#33310,#33311) ;
#29432=AXIS2_PLACEMENT_3D('',#42477,#33314,#33315) ;
#29433=AXIS2_PLACEMENT_3D('',#42483,#33318,#33319) ;
#29434=AXIS2_PLACEMENT_3D('',#42489,#33322,#33323) ;
#29435=AXIS2_PLACEMENT_3D('',#42495,#33326,#33327) ;
#29436=AXIS2_PLACEMENT_3D('',#42503,#33331,#33332) ;
#29437=AXIS2_PLACEMENT_3D('',#42509,#33335,#33336) ;
#29438=AXIS2_PLACEMENT_3D('',#42515,#33339,#33340) ;
#29439=AXIS2_PLACEMENT_3D('',#42521,#33343,#33344) ;
#29440=AXIS2_PLACEMENT_3D('',#42527,#33347,#33348) ;
#29441=AXIS2_PLACEMENT_3D('',#42533,#33351,#33352) ;
#29442=AXIS2_PLACEMENT_3D('',#42539,#33355,#33356) ;
#29443=AXIS2_PLACEMENT_3D('',#42547,#33360,#33361) ;
#29444=AXIS2_PLACEMENT_3D('',#42553,#33364,#33365) ;
#29445=AXIS2_PLACEMENT_3D('',#42559,#33368,#33369) ;
#29446=AXIS2_PLACEMENT_3D('',#42576,#33380,#33381) ;
#29447=AXIS2_PLACEMENT_3D('',#42582,#33385,#33386) ;
#29448=AXIS2_PLACEMENT_3D('',#42585,#33388,#33389) ;
#29449=AXIS2_PLACEMENT_3D('',#42586,#33390,#33391) ;
#29450=AXIS2_PLACEMENT_3D('',#42597,#33397,#33398) ;
#29451=AXIS2_PLACEMENT_3D('',#42639,#33419,#33420) ;
#29452=AXIS2_PLACEMENT_3D('',#42696,#33449,#33450) ;
#29453=AXIS2_PLACEMENT_3D('',#42701,#33452,#33453) ;
#29454=AXIS2_PLACEMENT_3D('',#42711,#33458,#33459) ;
#29455=AXIS2_PLACEMENT_3D('',#42719,#33463,#33464) ;
#29456=AXIS2_PLACEMENT_3D('',#42733,#33471,#33472) ;
#29457=AXIS2_PLACEMENT_3D('',#42771,#33491,#33492) ;
#29458=AXIS2_PLACEMENT_3D('',#42782,#33498,#33499) ;
#29459=AXIS2_PLACEMENT_3D('',#42809,#33512,#33513) ;
#29460=AXIS2_PLACEMENT_3D('',#42889,#33553,#33554) ;
#29461=AXIS2_PLACEMENT_3D('',#42895,#33557,#33558) ;
#29462=AXIS2_PLACEMENT_3D('',#42901,#33561,#33562) ;
#29463=AXIS2_PLACEMENT_3D('',#42909,#33566,#33567) ;
#29464=AXIS2_PLACEMENT_3D('',#42921,#33574,#33575) ;
#29465=AXIS2_PLACEMENT_3D('',#42923,#33577,#33578) ;
#29466=AXIS2_PLACEMENT_3D('',#42925,#33580,#33581) ;
#29467=AXIS2_PLACEMENT_3D('',#42927,#33583,#33584) ;
#29468=AXIS2_PLACEMENT_3D('',#42930,#33587,#33588) ;
#29469=AXIS2_PLACEMENT_3D('',#42933,#33591,#33592) ;
#29470=AXIS2_PLACEMENT_3D('',#42936,#33595,#33596) ;
#29471=AXIS2_PLACEMENT_3D('',#42939,#33599,#33600) ;
#29472=AXIS2_PLACEMENT_3D('',#42942,#33603,#33604) ;
#29473=AXIS2_PLACEMENT_3D('',#42945,#33607,#33608) ;
#29474=AXIS2_PLACEMENT_3D('',#42948,#33611,#33612) ;
#29475=AXIS2_PLACEMENT_3D('',#42951,#33615,#33616) ;
#29476=AXIS2_PLACEMENT_3D('',#42954,#33619,#33620) ;
#29477=AXIS2_PLACEMENT_3D('',#42957,#33623,#33624) ;
#29478=AXIS2_PLACEMENT_3D('',#42959,#33626,#33627) ;
#29479=AXIS2_PLACEMENT_3D('',#42961,#33629,#33630) ;
#29480=AXIS2_PLACEMENT_3D('',#42964,#33633,#33634) ;
#29481=AXIS2_PLACEMENT_3D('',#42966,#33636,#33637) ;
#29482=AXIS2_PLACEMENT_3D('',#42968,#33639,#33640) ;
#29483=AXIS2_PLACEMENT_3D('',#42970,#33642,#33643) ;
#29484=AXIS2_PLACEMENT_3D('',#42971,#33644,#33645) ;
#29485=AXIS2_PLACEMENT_3D('',#42973,#33647,#33648) ;
#29486=AXIS2_PLACEMENT_3D('',#42975,#33650,#33651) ;
#29487=AXIS2_PLACEMENT_3D('',#42977,#33653,#33654) ;
#29488=AXIS2_PLACEMENT_3D('',#42979,#33656,#33657) ;
#29489=AXIS2_PLACEMENT_3D('',#42981,#33659,#33660) ;
#29490=AXIS2_PLACEMENT_3D('',#42983,#33662,#33663) ;
#29491=AXIS2_PLACEMENT_3D('',#42985,#33665,#33666) ;
#29492=AXIS2_PLACEMENT_3D('',#42987,#33668,#33669) ;
#29493=AXIS2_PLACEMENT_3D('',#42989,#33671,#33672) ;
#29494=AXIS2_PLACEMENT_3D('',#42992,#33675,#33676) ;
#29495=AXIS2_PLACEMENT_3D('',#42994,#33678,#33679) ;
#29496=AXIS2_PLACEMENT_3D('',#42996,#33681,#33682) ;
#29497=AXIS2_PLACEMENT_3D('',#42999,#33685,#33686) ;
#29498=AXIS2_PLACEMENT_3D('',#43001,#33688,#33689) ;
#29499=AXIS2_PLACEMENT_3D('',#43003,#33691,#33692) ;
#29500=AXIS2_PLACEMENT_3D('',#43005,#33694,#33695) ;
#29501=AXIS2_PLACEMENT_3D('',#43006,#33696,#33697) ;
#29502=AXIS2_PLACEMENT_3D('',#43009,#33700,#33701) ;
#29503=AXIS2_PLACEMENT_3D('',#43012,#33704,#33705) ;
#29504=AXIS2_PLACEMENT_3D('',#43015,#33708,#33709) ;
#29505=AXIS2_PLACEMENT_3D('',#43018,#33712,#33713) ;
#29506=AXIS2_PLACEMENT_3D('',#43021,#33716,#33717) ;
#29507=AXIS2_PLACEMENT_3D('',#43023,#33719,#33720) ;
#29508=AXIS2_PLACEMENT_3D('',#43025,#33722,#33723) ;
#29509=AXIS2_PLACEMENT_3D('',#43026,#33724,#33725) ;
#29510=AXIS2_PLACEMENT_3D('',#43028,#33727,#33728) ;
#29511=AXIS2_PLACEMENT_3D('',#43030,#33730,#33731) ;
#29512=AXIS2_PLACEMENT_3D('',#43031,#33732,#33733) ;
#29513=AXIS2_PLACEMENT_3D('',#43033,#33735,#33736) ;
#29514=AXIS2_PLACEMENT_3D('',#43034,#33737,#33738) ;
#29515=AXIS2_PLACEMENT_3D('',#43036,#33740,#33741) ;
#29516=AXIS2_PLACEMENT_3D('',#43037,#33742,#33743) ;
#29517=AXIS2_PLACEMENT_3D('',#43039,#33745,#33746) ;
#29518=AXIS2_PLACEMENT_3D('',#43040,#33747,#33748) ;
#29519=AXIS2_PLACEMENT_3D('',#43042,#33750,#33751) ;
#29520=AXIS2_PLACEMENT_3D('',#43044,#33753,#33754) ;
#29521=AXIS2_PLACEMENT_3D('',#43046,#33756,#33757) ;
#29522=AXIS2_PLACEMENT_3D('',#43049,#33760,#33761) ;
#29523=AXIS2_PLACEMENT_3D('',#43052,#33764,#33765) ;
#29524=AXIS2_PLACEMENT_3D('',#43054,#33767,#33768) ;
#29525=AXIS2_PLACEMENT_3D('',#43056,#33770,#33771) ;
#29526=AXIS2_PLACEMENT_3D('',#43058,#33773,#33774) ;
#29527=AXIS2_PLACEMENT_3D('',#43059,#33775,#33776) ;
#29528=AXIS2_PLACEMENT_3D('',#43061,#33778,#33779) ;
#29529=AXIS2_PLACEMENT_3D('',#43064,#33782,#33783) ;
#29530=AXIS2_PLACEMENT_3D('',#43067,#33786,#33787) ;
#29531=AXIS2_PLACEMENT_3D('',#43069,#33789,#33790) ;
#29532=AXIS2_PLACEMENT_3D('',#43072,#33793,#33794) ;
#29533=AXIS2_PLACEMENT_3D('',#43075,#33797,#33798) ;
#29534=AXIS2_PLACEMENT_3D('',#43077,#33800,#33801) ;
#29535=AXIS2_PLACEMENT_3D('',#43078,#33802,#33803) ;
#29536=AXIS2_PLACEMENT_3D('',#43080,#33805,#33806) ;
#29537=AXIS2_PLACEMENT_3D('',#43082,#33808,#33809) ;
#29538=AXIS2_PLACEMENT_3D('',#43083,#33810,#33811) ;
#29539=AXIS2_PLACEMENT_3D('',#43085,#33813,#33814) ;
#29540=AXIS2_PLACEMENT_3D('',#43086,#33815,#33816) ;
#29541=AXIS2_PLACEMENT_3D('',#43088,#33818,#33819) ;
#29542=AXIS2_PLACEMENT_3D('',#43090,#33821,#33822) ;
#29543=AXIS2_PLACEMENT_3D('',#43092,#33824,#33825) ;
#29544=AXIS2_PLACEMENT_3D('',#43094,#33827,#33828) ;
#29545=AXIS2_PLACEMENT_3D('',#43095,#33829,#33830) ;
#29546=AXIS2_PLACEMENT_3D('',#43097,#33832,#33833) ;
#29547=AXIS2_PLACEMENT_3D('',#43098,#33834,#33835) ;
#29548=AXIS2_PLACEMENT_3D('',#43100,#33837,#33838) ;
#29549=AXIS2_PLACEMENT_3D('',#43103,#33841,#33842) ;
#29550=AXIS2_PLACEMENT_3D('',#43105,#33844,#33845) ;
#29551=AXIS2_PLACEMENT_3D('',#43108,#33848,#33849) ;
#29552=AXIS2_PLACEMENT_3D('',#43110,#33851,#33852) ;
#29553=AXIS2_PLACEMENT_3D('',#43112,#33854,#33855) ;
#29554=AXIS2_PLACEMENT_3D('',#43114,#33857,#33858) ;
#29555=AXIS2_PLACEMENT_3D('',#43116,#33860,#33861) ;
#29556=AXIS2_PLACEMENT_3D('',#43117,#33862,#33863) ;
#29557=AXIS2_PLACEMENT_3D('',#43120,#33866,#33867) ;
#29558=AXIS2_PLACEMENT_3D('',#43123,#33870,#33871) ;
#29559=AXIS2_PLACEMENT_3D('',#43126,#33874,#33875) ;
#29560=AXIS2_PLACEMENT_3D('',#43129,#33878,#33879) ;
#29561=AXIS2_PLACEMENT_3D('',#43132,#33882,#33883) ;
#29562=AXIS2_PLACEMENT_3D('',#43134,#33885,#33886) ;
#29563=AXIS2_PLACEMENT_3D('',#43136,#33888,#33889) ;
#29564=AXIS2_PLACEMENT_3D('',#43137,#33890,#33891) ;
#29565=AXIS2_PLACEMENT_3D('',#43138,#33892,#33893) ;
#29566=AXIS2_PLACEMENT_3D('',#43140,#33895,#33896) ;
#29567=AXIS2_PLACEMENT_3D('',#43142,#33898,#33899) ;
#29568=AXIS2_PLACEMENT_3D('',#43143,#33900,#33901) ;
#29569=AXIS2_PLACEMENT_3D('',#43145,#33903,#33904) ;
#29570=AXIS2_PLACEMENT_3D('',#43147,#33906,#33907) ;
#29571=AXIS2_PLACEMENT_3D('',#43148,#33908,#33909) ;
#29572=AXIS2_PLACEMENT_3D('',#43150,#33911,#33912) ;
#29573=AXIS2_PLACEMENT_3D('',#43151,#33913,#33914) ;
#29574=AXIS2_PLACEMENT_3D('',#43153,#33916,#33917) ;
#29575=AXIS2_PLACEMENT_3D('',#43154,#33918,#33919) ;
#29576=AXIS2_PLACEMENT_3D('',#43156,#33921,#33922) ;
#29577=AXIS2_PLACEMENT_3D('',#43157,#33923,#33924) ;
#29578=AXIS2_PLACEMENT_3D('',#43159,#33926,#33927) ;
#29579=AXIS2_PLACEMENT_3D('',#43162,#33930,#33931) ;
#29580=AXIS2_PLACEMENT_3D('',#43165,#33934,#33935) ;
#29581=AXIS2_PLACEMENT_3D('',#43168,#33938,#33939) ;
#29582=AXIS2_PLACEMENT_3D('',#43171,#33942,#33943) ;
#29583=AXIS2_PLACEMENT_3D('',#43173,#33945,#33946) ;
#29584=AXIS2_PLACEMENT_3D('',#43176,#33949,#33950) ;
#29585=AXIS2_PLACEMENT_3D('',#43178,#33952,#33953) ;
#29586=AXIS2_PLACEMENT_3D('',#43181,#33956,#33957) ;
#29587=AXIS2_PLACEMENT_3D('',#43183,#33959,#33960) ;
#29588=AXIS2_PLACEMENT_3D('',#43185,#33962,#33963) ;
#29589=AXIS2_PLACEMENT_3D('',#43187,#33965,#33966) ;
#29590=AXIS2_PLACEMENT_3D('',#43188,#33967,#33968) ;
#29591=AXIS2_PLACEMENT_3D('',#43190,#33970,#33971) ;
#29592=AXIS2_PLACEMENT_3D('',#43191,#33972,#33973) ;
#29593=AXIS2_PLACEMENT_3D('',#43193,#33975,#33976) ;
#29594=AXIS2_PLACEMENT_3D('',#43195,#33978,#33979) ;
#29595=AXIS2_PLACEMENT_3D('',#43196,#33980,#33981) ;
#29596=AXIS2_PLACEMENT_3D('',#43198,#33983,#33984) ;
#29597=AXIS2_PLACEMENT_3D('',#43200,#33986,#33987) ;
#29598=AXIS2_PLACEMENT_3D('',#43201,#33988,#33989) ;
#29599=AXIS2_PLACEMENT_3D('',#43203,#33991,#33992) ;
#29600=AXIS2_PLACEMENT_3D('',#43204,#33993,#33994) ;
#29601=AXIS2_PLACEMENT_3D('',#43206,#33996,#33997) ;
#29602=AXIS2_PLACEMENT_3D('',#43207,#33998,#33999) ;
#29603=AXIS2_PLACEMENT_3D('',#43209,#34001,#34002) ;
#29604=AXIS2_PLACEMENT_3D('',#43211,#34004,#34005) ;
#29605=AXIS2_PLACEMENT_3D('',#43213,#34007,#34008) ;
#29606=AXIS2_PLACEMENT_3D('',#43215,#34010,#34011) ;
#29607=AXIS2_PLACEMENT_3D('',#43217,#34013,#34014) ;
#29608=AXIS2_PLACEMENT_3D('',#43219,#34016,#34017) ;
#29609=AXIS2_PLACEMENT_3D('',#43222,#34020,#34021) ;
#29610=AXIS2_PLACEMENT_3D('',#43224,#34023,#34024) ;
#29611=AXIS2_PLACEMENT_3D('',#43225,#34025,#34026) ;
#29612=AXIS2_PLACEMENT_3D('',#43227,#34028,#34029) ;
#29613=AXIS2_PLACEMENT_3D('',#43230,#34032,#34033) ;
#29614=AXIS2_PLACEMENT_3D('',#43233,#34036,#34037) ;
#29615=AXIS2_PLACEMENT_3D('',#43236,#34040,#34041) ;
#29616=AXIS2_PLACEMENT_3D('',#43239,#34044,#34045) ;
#29617=AXIS2_PLACEMENT_3D('',#43242,#34048,#34049) ;
#29618=AXIS2_PLACEMENT_3D('',#43245,#34052,#34053) ;
#29619=AXIS2_PLACEMENT_3D('',#43246,#34054,#34055) ;
#29620=AXIS2_PLACEMENT_3D('',#43247,#34056,#34057) ;
#29621=AXIS2_PLACEMENT_3D('',#43249,#34059,#34060) ;
#29622=AXIS2_PLACEMENT_3D('',#43251,#34062,#34063) ;
#29623=AXIS2_PLACEMENT_3D('',#43252,#34064,#34065) ;
#29624=AXIS2_PLACEMENT_3D('',#43253,#34066,#34067) ;
#29625=AXIS2_PLACEMENT_3D('',#43255,#34069,#34070) ;
#29626=AXIS2_PLACEMENT_3D('',#43256,#34071,#34072) ;
#29627=AXIS2_PLACEMENT_3D('',#43258,#34074,#34075) ;
#29628=AXIS2_PLACEMENT_3D('',#43259,#34076,#34077) ;
#29629=AXIS2_PLACEMENT_3D('',#43261,#34079,#34080) ;
#29630=AXIS2_PLACEMENT_3D('',#43263,#34082,#34083) ;
#29631=AXIS2_PLACEMENT_3D('',#43264,#34084,#34085) ;
#29632=AXIS2_PLACEMENT_3D('',#43266,#34087,#34088) ;
#29633=AXIS2_PLACEMENT_3D('',#43267,#34089,#34090) ;
#29634=AXIS2_PLACEMENT_3D('',#43269,#34092,#34093) ;
#29635=AXIS2_PLACEMENT_3D('',#43271,#34095,#34096) ;
#29636=AXIS2_PLACEMENT_3D('',#43273,#34098,#34099) ;
#29637=AXIS2_PLACEMENT_3D('',#43275,#34101,#34102) ;
#29638=AXIS2_PLACEMENT_3D('',#43277,#34104,#34105) ;
#29639=AXIS2_PLACEMENT_3D('',#43279,#34107,#34108) ;
#29640=AXIS2_PLACEMENT_3D('',#43280,#34109,#34110) ;
#29641=AXIS2_PLACEMENT_3D('',#43283,#34113,#34114) ;
#29642=AXIS2_PLACEMENT_3D('',#43286,#34117,#34118) ;
#29643=AXIS2_PLACEMENT_3D('',#43289,#34121,#34122) ;
#29644=AXIS2_PLACEMENT_3D('',#43292,#34125,#34126) ;
#29645=AXIS2_PLACEMENT_3D('',#43295,#34129,#34130) ;
#29646=AXIS2_PLACEMENT_3D('',#43296,#34131,#34132) ;
#29647=AXIS2_PLACEMENT_3D('',#43297,#34133,#34134) ;
#29648=AXIS2_PLACEMENT_3D('',#43299,#34136,#34137) ;
#29649=AXIS2_PLACEMENT_3D('',#43300,#34138,#34139) ;
#29650=AXIS2_PLACEMENT_3D('',#43301,#34140,#34141) ;
#29651=AXIS2_PLACEMENT_3D('',#43302,#34142,#34143) ;
#29652=AXIS2_PLACEMENT_3D('',#43304,#34145,#34146) ;
#29653=AXIS2_PLACEMENT_3D('',#43306,#34148,#34149) ;
#29654=AXIS2_PLACEMENT_3D('',#43307,#34150,#34151) ;
#29655=AXIS2_PLACEMENT_3D('',#43309,#34153,#34154) ;
#29656=AXIS2_PLACEMENT_3D('',#43311,#34156,#34157) ;
#29657=AXIS2_PLACEMENT_3D('',#43312,#34158,#34159) ;
#29658=AXIS2_PLACEMENT_3D('',#43314,#34161,#34162) ;
#29659=AXIS2_PLACEMENT_3D('',#43316,#34164,#34165) ;
#29660=AXIS2_PLACEMENT_3D('',#43319,#34168,#34169) ;
#29661=AXIS2_PLACEMENT_3D('',#43322,#34172,#34173) ;
#29662=AXIS2_PLACEMENT_3D('',#43325,#34176,#34177) ;
#29663=AXIS2_PLACEMENT_3D('',#43327,#34179,#34180) ;
#29664=AXIS2_PLACEMENT_3D('',#43330,#34183,#34184) ;
#29665=AXIS2_PLACEMENT_3D('',#43331,#34185,#34186) ;
#29666=AXIS2_PLACEMENT_3D('',#43333,#34188,#34189) ;
#29667=AXIS2_PLACEMENT_3D('',#43335,#34191,#34192) ;
#29668=AXIS2_PLACEMENT_3D('',#43336,#34193,#34194) ;
#29669=AXIS2_PLACEMENT_3D('',#43338,#34196,#34197) ;
#29670=AXIS2_PLACEMENT_3D('',#43339,#34198,#34199) ;
#29671=AXIS2_PLACEMENT_3D('',#43340,#34200,#34201) ;
#29672=AXIS2_PLACEMENT_3D('',#43342,#34203,#34204) ;
#29673=AXIS2_PLACEMENT_3D('',#43343,#34205,#34206) ;
#29674=AXIS2_PLACEMENT_3D('',#43345,#34208,#34209) ;
#29675=AXIS2_PLACEMENT_3D('',#43347,#34211,#34212) ;
#29676=AXIS2_PLACEMENT_3D('',#43349,#34214,#34215) ;
#29677=AXIS2_PLACEMENT_3D('',#43350,#34216,#34217) ;
#29678=AXIS2_PLACEMENT_3D('',#43352,#34219,#34220) ;
#29679=AXIS2_PLACEMENT_3D('',#43354,#34222,#34223) ;
#29680=AXIS2_PLACEMENT_3D('',#43356,#34225,#34226) ;
#29681=AXIS2_PLACEMENT_3D('',#43357,#34227,#34228) ;
#29682=AXIS2_PLACEMENT_3D('',#43359,#34230,#34231) ;
#29683=AXIS2_PLACEMENT_3D('',#43361,#34233,#34234) ;
#29684=AXIS2_PLACEMENT_3D('',#43364,#34237,#34238) ;
#29685=AXIS2_PLACEMENT_3D('',#43367,#34241,#34242) ;
#29686=AXIS2_PLACEMENT_3D('',#43370,#34245,#34246) ;
#29687=AXIS2_PLACEMENT_3D('',#43372,#34248,#34249) ;
#29688=AXIS2_PLACEMENT_3D('',#43374,#34251,#34252) ;
#29689=AXIS2_PLACEMENT_3D('',#43375,#34253,#34254) ;
#29690=AXIS2_PLACEMENT_3D('',#43377,#34256,#34257) ;
#29691=AXIS2_PLACEMENT_3D('',#43378,#34258,#34259) ;
#29692=AXIS2_PLACEMENT_3D('',#43380,#34261,#34262) ;
#29693=AXIS2_PLACEMENT_3D('',#43381,#34263,#34264) ;
#29694=AXIS2_PLACEMENT_3D('',#43382,#34265,#34266) ;
#29695=AXIS2_PLACEMENT_3D('',#43384,#34268,#34269) ;
#29696=AXIS2_PLACEMENT_3D('',#43386,#34271,#34272) ;
#29697=AXIS2_PLACEMENT_3D('',#43387,#34273,#34274) ;
#29698=AXIS2_PLACEMENT_3D('',#43389,#34276,#34277) ;
#29699=AXIS2_PLACEMENT_3D('',#43390,#34278,#34279) ;
#29700=AXIS2_PLACEMENT_3D('',#43393,#34282,#34283) ;
#29701=AXIS2_PLACEMENT_3D('',#43394,#34284,#34285) ;
#29702=AXIS2_PLACEMENT_3D('',#43397,#34288,#34289) ;
#29703=AXIS2_PLACEMENT_3D('',#43398,#34290,#34291) ;
#29704=AXIS2_PLACEMENT_3D('',#43400,#34293,#34294) ;
#29705=AXIS2_PLACEMENT_3D('',#43401,#34295,#34296) ;
#29706=AXIS2_PLACEMENT_3D('',#43403,#34298,#34299) ;
#29707=AXIS2_PLACEMENT_3D('',#43404,#34300,#34301) ;
#29708=AXIS2_PLACEMENT_3D('',#43406,#34303,#34304) ;
#29709=AXIS2_PLACEMENT_3D('',#43408,#34306,#34307) ;
#29710=AXIS2_PLACEMENT_3D('',#43410,#34309,#34310) ;
#29711=AXIS2_PLACEMENT_3D('',#43412,#34312,#34313) ;
#29712=AXIS2_PLACEMENT_3D('',#43414,#34315,#34316) ;
#29713=AXIS2_PLACEMENT_3D('',#43416,#34318,#34319) ;
#29714=AXIS2_PLACEMENT_3D('',#43417,#34320,#34321) ;
#29715=AXIS2_PLACEMENT_3D('',#43419,#34323,#34324) ;
#29716=AXIS2_PLACEMENT_3D('',#43420,#34325,#34326) ;
#29717=AXIS2_PLACEMENT_3D('',#43422,#34328,#34329) ;
#29718=AXIS2_PLACEMENT_3D('',#43424,#34331,#34332) ;
#29719=AXIS2_PLACEMENT_3D('',#43425,#34333,#34334) ;
#29720=AXIS2_PLACEMENT_3D('',#43426,#34335,#34336) ;
#29721=AXIS2_PLACEMENT_3D('',#43428,#34338,#34339) ;
#29722=AXIS2_PLACEMENT_3D('',#43430,#34341,#34342) ;
#29723=AXIS2_PLACEMENT_3D('',#43432,#34344,#34345) ;
#29724=AXIS2_PLACEMENT_3D('',#43433,#34346,#34347) ;
#29725=AXIS2_PLACEMENT_3D('',#43434,#34348,#34349) ;
#29726=AXIS2_PLACEMENT_3D('',#43436,#34351,#34352) ;
#29727=AXIS2_PLACEMENT_3D('',#43438,#34354,#34355) ;
#29728=AXIS2_PLACEMENT_3D('',#43439,#34356,#34357) ;
#29729=AXIS2_PLACEMENT_3D('',#43440,#34358,#34359) ;
#32798=DIRECTION('axis',(0.,0.,1.)) ;
#32799=DIRECTION('refdir',(1.,0.,0.)) ;
#32800=DIRECTION('center_axis',(1.,0.,0.)) ;
#32801=DIRECTION('ref_axis',(0.,0.,-1.)) ;
#32802=DIRECTION('',(0.,0.,1.)) ;
#32803=DIRECTION('',(0.,1.,0.)) ;
#32804=DIRECTION('',(0.,0.,-1.)) ;
#32805=DIRECTION('',(0.,-1.,0.)) ;
#32806=DIRECTION('center_axis',(1.,0.,0.)) ;
#32807=DIRECTION('ref_axis',(0.,0.,-1.)) ;
#32808=DIRECTION('',(0.,0.,1.)) ;
#32809=DIRECTION('',(0.,1.,0.)) ;
#32810=DIRECTION('',(0.,0.,-1.)) ;
#32811=DIRECTION('',(0.,-1.,0.)) ;
#32812=DIRECTION('center_axis',(1.,0.,0.)) ;
#32813=DIRECTION('ref_axis',(0.,0.,-1.)) ;
#32814=DIRECTION('',(0.,0.,1.)) ;
#32815=DIRECTION('',(0.,1.,0.)) ;
#32816=DIRECTION('',(0.,0.,-1.)) ;
#32817=DIRECTION('',(0.,-1.,0.)) ;
#32818=DIRECTION('center_axis',(1.,0.,0.)) ;
#32819=DIRECTION('ref_axis',(0.,0.,-1.)) ;
#32820=DIRECTION('',(0.,0.,1.)) ;
#32821=DIRECTION('',(0.,1.,0.)) ;
#32822=DIRECTION('',(0.,0.,-1.)) ;
#32823=DIRECTION('',(0.,-1.,0.)) ;
#32824=DIRECTION('center_axis',(1.,0.,0.)) ;
#32825=DIRECTION('ref_axis',(0.,0.,-1.)) ;
#32826=DIRECTION('',(0.,0.,1.)) ;
#32827=DIRECTION('',(0.,1.,0.)) ;
#32828=DIRECTION('',(0.,0.,-1.)) ;
#32829=DIRECTION('',(0.,-1.,0.)) ;
#32830=DIRECTION('center_axis',(1.,0.,0.)) ;
#32831=DIRECTION('ref_axis',(0.,0.,-1.)) ;
#32832=DIRECTION('',(0.,0.,1.)) ;
#32833=DIRECTION('',(0.,1.,0.)) ;
#32834=DIRECTION('',(0.,0.,-1.)) ;
#32835=DIRECTION('',(0.,-1.,0.)) ;
#32836=DIRECTION('center_axis',(-1.,0.,0.)) ;
#32837=DIRECTION('ref_axis',(0.,0.,1.)) ;
#32838=DIRECTION('',(0.,0.,1.)) ;
#32839=DIRECTION('',(0.,-1.,0.)) ;
#32840=DIRECTION('',(0.,0.,-1.)) ;
#32841=DIRECTION('',(0.,1.,0.)) ;
#32842=DIRECTION('center_axis',(-1.,0.,0.)) ;
#32843=DIRECTION('ref_axis',(0.,0.,1.)) ;
#32844=DIRECTION('',(0.,0.,-1.)) ;
#32845=DIRECTION('',(0.,1.,0.)) ;
#32846=DIRECTION('',(0.,0.,-1.)) ;
#32847=DIRECTION('',(0.,-1.,0.)) ;
#32848=DIRECTION('center_axis',(-1.,0.,0.)) ;
#32849=DIRECTION('ref_axis',(0.,0.,1.)) ;
#32850=DIRECTION('',(0.,0.,-1.)) ;
#32851=DIRECTION('',(0.,1.,0.)) ;
#32852=DIRECTION('',(0.,0.,1.)) ;
#32853=DIRECTION('',(0.,-1.,0.)) ;
#32854=DIRECTION('center_axis',(-1.,0.,0.)) ;
#32855=DIRECTION('ref_axis',(0.,0.,1.)) ;
#32856=DIRECTION('',(0.,0.,-1.)) ;
#32857=DIRECTION('',(0.,1.,0.)) ;
#32858=DIRECTION('',(0.,0.,1.)) ;
#32859=DIRECTION('',(0.,-1.,0.)) ;
#32860=DIRECTION('center_axis',(-1.,0.,0.)) ;
#32861=DIRECTION('ref_axis',(0.,0.,1.)) ;
#32862=DIRECTION('',(0.,0.,-1.)) ;
#32863=DIRECTION('',(0.,1.,0.)) ;
#32864=DIRECTION('',(0.,0.,1.)) ;
#32865=DIRECTION('',(0.,-1.,0.)) ;
#32866=DIRECTION('center_axis',(-1.,0.,0.)) ;
#32867=DIRECTION('ref_axis',(0.,0.,1.)) ;
#32868=DIRECTION('',(0.,0.,-1.)) ;
#32869=DIRECTION('',(0.,1.,0.)) ;
#32870=DIRECTION('',(0.,0.,1.)) ;
#32871=DIRECTION('',(0.,-1.,0.)) ;
#32872=DIRECTION('center_axis',(0.,1.,0.)) ;
#32873=DIRECTION('ref_axis',(0.,0.,1.)) ;
#32874=DIRECTION('',(0.,0.,1.)) ;
#32875=DIRECTION('',(-1.,0.,0.)) ;
#32876=DIRECTION('',(1.,0.,0.)) ;
#32877=DIRECTION('center_axis',(0.,-1.,0.)) ;
#32878=DIRECTION('ref_axis',(0.,0.,-1.)) ;
#32879=DIRECTION('',(0.,0.,-1.)) ;
#32880=DIRECTION('',(-1.,0.,0.)) ;
#32881=DIRECTION('',(1.,0.,0.)) ;
#32882=DIRECTION('center_axis',(0.,0.,1.)) ;
#32883=DIRECTION('ref_axis',(1.,0.,0.)) ;
#32884=DIRECTION('center_axis',(0.,0.,1.)) ;
#32885=DIRECTION('ref_axis',(1.,0.,0.)) ;
#32886=DIRECTION('',(0.,0.,-1.)) ;
#32887=DIRECTION('center_axis',(0.,0.,-1.)) ;
#32888=DIRECTION('ref_axis',(1.,0.,0.)) ;
#32889=DIRECTION('center_axis',(0.,0.,1.)) ;
#32890=DIRECTION('ref_axis',(1.,0.,0.)) ;
#32891=DIRECTION('center_axis',(0.,0.,-1.)) ;
#32892=DIRECTION('ref_axis',(1.,0.,0.)) ;
#32893=DIRECTION('',(0.,0.,1.)) ;
#32894=DIRECTION('center_axis',(0.,0.,1.)) ;
#32895=DIRECTION('ref_axis',(1.,0.,0.)) ;
#32896=DIRECTION('center_axis',(0.,0.,1.)) ;
#32897=DIRECTION('ref_axis',(1.,0.,0.)) ;
#32898=DIRECTION('center_axis',(0.,0.,1.)) ;
#32899=DIRECTION('ref_axis',(1.,0.,0.)) ;
#32900=DIRECTION('',(0.,0.,1.)) ;
#32901=DIRECTION('center_axis',(0.,0.,-1.)) ;
#32902=DIRECTION('ref_axis',(1.,0.,0.)) ;
#32903=DIRECTION('center_axis',(0.,-1.,0.)) ;
#32904=DIRECTION('ref_axis',(0.,0.,-1.)) ;
#32905=DIRECTION('',(1.,0.,0.)) ;
#32906=DIRECTION('',(0.,0.,1.)) ;
#32907=DIRECTION('',(-1.,0.,0.)) ;
#32908=DIRECTION('center_axis',(0.,1.,0.)) ;
#32909=DIRECTION('ref_axis',(0.,0.,1.)) ;
#32910=DIRECTION('',(-1.,0.,0.)) ;
#32911=DIRECTION('',(0.,0.,-1.)) ;
#32912=DIRECTION('',(1.,0.,0.)) ;
#32913=DIRECTION('center_axis',(0.,-1.,0.)) ;
#32914=DIRECTION('ref_axis',(0.,0.,-1.)) ;
#32915=DIRECTION('',(1.,0.,0.)) ;
#32916=DIRECTION('',(0.,0.,1.)) ;
#32917=DIRECTION('',(-1.,0.,0.)) ;
#32918=DIRECTION('center_axis',(0.,1.,0.)) ;
#32919=DIRECTION('ref_axis',(0.,0.,1.)) ;
#32920=DIRECTION('',(-1.,0.,0.)) ;
#32921=DIRECTION('',(0.,0.,-1.)) ;
#32922=DIRECTION('',(1.,0.,0.)) ;
#32923=DIRECTION('center_axis',(0.,-1.,0.)) ;
#32924=DIRECTION('ref_axis',(0.,0.,-1.)) ;
#32925=DIRECTION('',(1.,0.,0.)) ;
#32926=DIRECTION('',(0.,0.,1.)) ;
#32927=DIRECTION('',(-1.,0.,0.)) ;
#32928=DIRECTION('center_axis',(0.,1.,0.)) ;
#32929=DIRECTION('ref_axis',(0.,0.,1.)) ;
#32930=DIRECTION('',(-1.,0.,0.)) ;
#32931=DIRECTION('',(0.,0.,-1.)) ;
#32932=DIRECTION('',(1.,0.,0.)) ;
#32933=DIRECTION('center_axis',(0.,-1.,0.)) ;
#32934=DIRECTION('ref_axis',(0.,0.,-1.)) ;
#32935=DIRECTION('',(1.,0.,0.)) ;
#32936=DIRECTION('',(0.,0.,1.)) ;
#32937=DIRECTION('',(-1.,0.,0.)) ;
#32938=DIRECTION('center_axis',(0.,-1.,0.)) ;
#32939=DIRECTION('ref_axis',(0.,0.,-1.)) ;
#32940=DIRECTION('',(1.,0.,0.)) ;
#32941=DIRECTION('',(0.,0.,1.)) ;
#32942=DIRECTION('',(-1.,0.,0.)) ;
#32943=DIRECTION('center_axis',(0.,0.,1.)) ;
#32944=DIRECTION('ref_axis',(1.,0.,0.)) ;
#32945=DIRECTION('',(0.,1.,0.)) ;
#32946=DIRECTION('',(-1.,0.,0.)) ;
#32947=DIRECTION('center_axis',(0.,0.,1.)) ;
#32948=DIRECTION('ref_axis',(1.,0.,0.)) ;
#32949=DIRECTION('',(0.,1.,0.)) ;
#32950=DIRECTION('',(-1.,0.,0.)) ;
#32951=DIRECTION('center_axis',(0.,0.,1.)) ;
#32952=DIRECTION('ref_axis',(1.,0.,0.)) ;
#32953=DIRECTION('',(0.,1.,0.)) ;
#32954=DIRECTION('',(-1.,0.,0.)) ;
#32955=DIRECTION('center_axis',(0.,0.,1.)) ;
#32956=DIRECTION('ref_axis',(1.,0.,0.)) ;
#32957=DIRECTION('',(0.,1.,0.)) ;
#32958=DIRECTION('',(-1.,0.,0.)) ;
#32959=DIRECTION('',(0.,-1.,0.)) ;
#32960=DIRECTION('center_axis',(0.,0.,1.)) ;
#32961=DIRECTION('ref_axis',(1.,0.,0.)) ;
#32962=DIRECTION('',(-1.,0.,0.)) ;
#32963=DIRECTION('',(0.,-1.,0.)) ;
#32964=DIRECTION('center_axis',(0.,0.,1.)) ;
#32965=DIRECTION('ref_axis',(1.,0.,0.)) ;
#32966=DIRECTION('',(-1.,0.,0.)) ;
#32967=DIRECTION('',(0.,-1.,0.)) ;
#32968=DIRECTION('center_axis',(0.,0.,1.)) ;
#32969=DIRECTION('ref_axis',(1.,0.,0.)) ;
#32970=DIRECTION('',(-1.,0.,0.)) ;
#32971=DIRECTION('',(0.,-1.,0.)) ;
#32972=DIRECTION('center_axis',(0.,0.,1.)) ;
#32973=DIRECTION('ref_axis',(1.,0.,0.)) ;
#32974=DIRECTION('',(-1.,0.,0.)) ;
#32975=DIRECTION('',(0.,-1.,0.)) ;
#32976=DIRECTION('center_axis',(0.,0.,1.)) ;
#32977=DIRECTION('ref_axis',(1.,0.,0.)) ;
#32978=DIRECTION('',(-1.,0.,0.)) ;
#32979=DIRECTION('',(0.,-1.,0.)) ;
#32980=DIRECTION('center_axis',(0.,0.,1.)) ;
#32981=DIRECTION('ref_axis',(1.,0.,0.)) ;
#32982=DIRECTION('',(-1.,0.,0.)) ;
#32983=DIRECTION('',(0.,-1.,0.)) ;
#32984=DIRECTION('center_axis',(0.,0.,1.)) ;
#32985=DIRECTION('ref_axis',(1.,0.,0.)) ;
#32986=DIRECTION('',(-1.,0.,0.)) ;
#32987=DIRECTION('',(0.,-1.,0.)) ;
#32988=DIRECTION('',(1.,0.,0.)) ;
#32989=DIRECTION('center_axis',(0.,0.,1.)) ;
#32990=DIRECTION('ref_axis',(1.,0.,0.)) ;
#32991=DIRECTION('',(0.,-1.,0.)) ;
#32992=DIRECTION('',(1.,0.,0.)) ;
#32993=DIRECTION('center_axis',(0.,0.,1.)) ;
#32994=DIRECTION('ref_axis',(1.,0.,0.)) ;
#32995=DIRECTION('',(0.,-1.,0.)) ;
#32996=DIRECTION('',(1.,0.,0.)) ;
#32997=DIRECTION('center_axis',(0.,0.,1.)) ;
#32998=DIRECTION('ref_axis',(1.,0.,0.)) ;
#32999=DIRECTION('',(0.,-1.,0.)) ;
#33000=DIRECTION('',(1.,0.,0.)) ;
#33001=DIRECTION('center_axis',(0.,0.,1.)) ;
#33002=DIRECTION('ref_axis',(1.,0.,0.)) ;
#33003=DIRECTION('',(0.,-1.,0.)) ;
#33004=DIRECTION('',(1.,0.,0.)) ;
#33005=DIRECTION('center_axis',(0.,0.,1.)) ;
#33006=DIRECTION('ref_axis',(1.,0.,0.)) ;
#33007=DIRECTION('',(0.,-1.,0.)) ;
#33008=DIRECTION('',(1.,0.,0.)) ;
#33009=DIRECTION('center_axis',(0.,0.,1.)) ;
#33010=DIRECTION('ref_axis',(1.,0.,0.)) ;
#33011=DIRECTION('',(0.,-1.,0.)) ;
#33012=DIRECTION('',(1.,0.,0.)) ;
#33013=DIRECTION('center_axis',(0.,0.,1.)) ;
#33014=DIRECTION('ref_axis',(1.,0.,0.)) ;
#33015=DIRECTION('',(0.,-1.,0.)) ;
#33016=DIRECTION('',(1.,0.,0.)) ;
#33017=DIRECTION('',(0.,1.,0.)) ;
#33018=DIRECTION('center_axis',(0.,0.,1.)) ;
#33019=DIRECTION('ref_axis',(1.,0.,0.)) ;
#33020=DIRECTION('',(1.,0.,0.)) ;
#33021=DIRECTION('',(0.,1.,0.)) ;
#33022=DIRECTION('center_axis',(0.,0.,1.)) ;
#33023=DIRECTION('ref_axis',(1.,0.,0.)) ;
#33024=DIRECTION('',(1.,0.,0.)) ;
#33025=DIRECTION('',(0.,1.,0.)) ;
#33026=DIRECTION('center_axis',(0.,0.,1.)) ;
#33027=DIRECTION('ref_axis',(1.,0.,0.)) ;
#33028=DIRECTION('',(1.,0.,0.)) ;
#33029=DIRECTION('',(0.,1.,0.)) ;
#33030=DIRECTION('center_axis',(0.,0.,1.)) ;
#33031=DIRECTION('ref_axis',(1.,0.,0.)) ;
#33032=DIRECTION('center_axis',(0.,0.,1.)) ;
#33033=DIRECTION('ref_axis',(1.,0.,0.)) ;
#33034=DIRECTION('',(1.,0.,0.)) ;
#33035=DIRECTION('',(0.,1.,0.)) ;
#33036=DIRECTION('center_axis',(0.,0.,1.)) ;
#33037=DIRECTION('ref_axis',(1.,0.,0.)) ;
#33038=DIRECTION('',(1.,0.,0.)) ;
#33039=DIRECTION('',(0.,1.,0.)) ;
#33040=DIRECTION('center_axis',(0.,0.,1.)) ;
#33041=DIRECTION('ref_axis',(1.,0.,0.)) ;
#33042=DIRECTION('',(1.,0.,0.)) ;
#33043=DIRECTION('',(0.,1.,0.)) ;
#33044=DIRECTION('',(-1.,0.,0.)) ;
#33045=DIRECTION('center_axis',(0.,0.,1.)) ;
#33046=DIRECTION('ref_axis',(1.,0.,0.)) ;
#33047=DIRECTION('',(0.,1.,0.)) ;
#33048=DIRECTION('',(-1.,0.,0.)) ;
#33049=DIRECTION('center_axis',(0.,0.,1.)) ;
#33050=DIRECTION('ref_axis',(1.,0.,0.)) ;
#33051=DIRECTION('',(0.,1.,0.)) ;
#33052=DIRECTION('',(-1.,0.,0.)) ;
#33053=DIRECTION('',(-1.,0.,0.)) ;
#33054=DIRECTION('center_axis',(0.,0.,-1.)) ;
#33055=DIRECTION('ref_axis',(1.,0.,0.)) ;
#33056=DIRECTION('',(-1.,0.,0.)) ;
#33057=DIRECTION('center_axis',(0.,0.,-1.)) ;
#33058=DIRECTION('ref_axis',(1.,0.,0.)) ;
#33059=DIRECTION('',(-1.,0.,0.)) ;
#33060=DIRECTION('center_axis',(0.,0.,-1.)) ;
#33061=DIRECTION('ref_axis',(1.,0.,0.)) ;
#33062=DIRECTION('',(0.,1.,0.)) ;
#33063=DIRECTION('',(1.,0.,0.)) ;
#33064=DIRECTION('',(0.,1.,0.)) ;
#33065=DIRECTION('',(1.,0.,0.)) ;
#33066=DIRECTION('',(0.,1.,0.)) ;
#33067=DIRECTION('',(1.,0.,0.)) ;
#33068=DIRECTION('',(0.,1.,0.)) ;
#33069=DIRECTION('',(1.,0.,0.)) ;
#33070=DIRECTION('',(0.,1.,0.)) ;
#33071=DIRECTION('',(1.,0.,0.)) ;
#33072=DIRECTION('center_axis',(0.,0.,-1.)) ;
#33073=DIRECTION('ref_axis',(1.,0.,0.)) ;
#33074=DIRECTION('',(0.,1.,0.)) ;
#33075=DIRECTION('center_axis',(0.,0.,-1.)) ;
#33076=DIRECTION('ref_axis',(1.,0.,0.)) ;
#33077=DIRECTION('',(-1.,0.,0.)) ;
#33078=DIRECTION('',(0.,-1.,0.)) ;
#33079=DIRECTION('',(-1.,0.,0.)) ;
#33080=DIRECTION('',(0.,1.,0.)) ;
#33081=DIRECTION('',(1.,0.,0.)) ;
#33082=DIRECTION('',(0.,-1.,0.)) ;
#33083=DIRECTION('',(-1.,0.,0.)) ;
#33084=DIRECTION('',(0.,1.,0.)) ;
#33085=DIRECTION('',(1.,0.,0.)) ;
#33086=DIRECTION('',(0.,-1.,0.)) ;
#33087=DIRECTION('',(-1.,0.,0.)) ;
#33088=DIRECTION('',(0.,1.,0.)) ;
#33089=DIRECTION('',(1.,0.,0.)) ;
#33090=DIRECTION('',(1.,0.,0.)) ;
#33091=DIRECTION('',(0.,-1.,0.)) ;
#33092=DIRECTION('',(-1.,0.,0.)) ;
#33093=DIRECTION('',(0.,1.,0.)) ;
#33094=DIRECTION('',(-1.,0.,0.)) ;
#33095=DIRECTION('',(0.,1.,0.)) ;
#33096=DIRECTION('center_axis',(0.,0.,-1.)) ;
#33097=DIRECTION('ref_axis',(1.,0.,0.)) ;
#33098=DIRECTION('',(0.,-1.,0.)) ;
#33099=DIRECTION('',(-1.,0.,0.)) ;
#33100=DIRECTION('',(0.,1.,0.)) ;
#33101=DIRECTION('center_axis',(0.,0.,-1.)) ;
#33102=DIRECTION('ref_axis',(1.,0.,0.)) ;
#33103=DIRECTION('',(0.,-1.,0.)) ;
#33104=DIRECTION('',(0.,-1.,0.)) ;
#33105=DIRECTION('',(-1.,0.,0.)) ;
#33106=DIRECTION('',(0.,1.,0.)) ;
#33107=DIRECTION('center_axis',(0.,0.,-1.)) ;
#33108=DIRECTION('ref_axis',(1.,0.,0.)) ;
#33109=DIRECTION('',(1.,0.,0.)) ;
#33110=DIRECTION('',(-1.,0.,0.)) ;
#33111=DIRECTION('center_axis',(0.,0.,-1.)) ;
#33112=DIRECTION('ref_axis',(1.,0.,0.)) ;
#33113=DIRECTION('',(0.,-1.,0.)) ;
#33114=DIRECTION('center_axis',(0.,0.,-1.)) ;
#33115=DIRECTION('ref_axis',(1.,0.,0.)) ;
#33116=DIRECTION('',(0.,1.,0.)) ;
#33117=DIRECTION('',(1.,0.,0.)) ;
#33118=DIRECTION('',(0.,-1.,0.)) ;
#33119=DIRECTION('',(0.,-1.,0.)) ;
#33120=DIRECTION('',(-1.,0.,0.)) ;
#33121=DIRECTION('',(0.,1.,0.)) ;
#33122=DIRECTION('',(1.,0.,0.)) ;
#33123=DIRECTION('',(0.,-1.,0.)) ;
#33124=DIRECTION('',(-1.,0.,0.)) ;
#33125=DIRECTION('',(0.,1.,0.)) ;
#33126=DIRECTION('',(1.,0.,0.)) ;
#33127=DIRECTION('',(0.,-1.,0.)) ;
#33128=DIRECTION('',(-1.,0.,0.)) ;
#33129=DIRECTION('',(0.,1.,0.)) ;
#33130=DIRECTION('',(1.,0.,0.)) ;
#33131=DIRECTION('',(0.,-1.,0.)) ;
#33132=DIRECTION('',(-1.,0.,0.)) ;
#33133=DIRECTION('',(0.,1.,0.)) ;
#33134=DIRECTION('',(1.,0.,0.)) ;
#33135=DIRECTION('',(0.,-1.,0.)) ;
#33136=DIRECTION('',(-1.,0.,0.)) ;
#33137=DIRECTION('',(0.,1.,0.)) ;
#33138=DIRECTION('',(1.,0.,0.)) ;
#33139=DIRECTION('',(0.,-1.,0.)) ;
#33140=DIRECTION('',(-1.,0.,0.)) ;
#33141=DIRECTION('center_axis',(0.,0.,-1.)) ;
#33142=DIRECTION('ref_axis',(1.,0.,0.)) ;
#33143=DIRECTION('',(1.,0.,0.)) ;
#33144=DIRECTION('',(0.,-1.,0.)) ;
#33145=DIRECTION('',(-1.,0.,0.)) ;
#33146=DIRECTION('',(0.,1.,0.)) ;
#33147=DIRECTION('',(1.,0.,0.)) ;
#33148=DIRECTION('',(0.,-1.,0.)) ;
#33149=DIRECTION('',(-1.,0.,0.)) ;
#33150=DIRECTION('',(0.,1.,0.)) ;
#33151=DIRECTION('',(1.,0.,0.)) ;
#33152=DIRECTION('',(0.,-1.,0.)) ;
#33153=DIRECTION('center_axis',(0.,0.,-1.)) ;
#33154=DIRECTION('ref_axis',(1.,0.,0.)) ;
#33155=DIRECTION('',(1.,0.,0.)) ;
#33156=DIRECTION('',(0.,-1.,0.)) ;
#33157=DIRECTION('',(-1.,0.,0.)) ;
#33158=DIRECTION('center_axis',(0.,0.,-1.)) ;
#33159=DIRECTION('ref_axis',(1.,0.,0.)) ;
#33160=DIRECTION('',(0.,1.,0.)) ;
#33161=DIRECTION('',(1.,0.,0.)) ;
#33162=DIRECTION('',(0.,-1.,0.)) ;
#33163=DIRECTION('center_axis',(0.,0.,-1.)) ;
#33164=DIRECTION('ref_axis',(1.,0.,0.)) ;
#33165=DIRECTION('',(1.,0.,0.)) ;
#33166=DIRECTION('',(0.,-1.,0.)) ;
#33167=DIRECTION('',(-1.,0.,0.)) ;
#33168=DIRECTION('',(0.,1.,0.)) ;
#33169=DIRECTION('',(1.,0.,0.)) ;
#33170=DIRECTION('',(-1.,0.,0.)) ;
#33171=DIRECTION('center_axis',(0.,0.,-1.)) ;
#33172=DIRECTION('ref_axis',(1.,0.,0.)) ;
#33173=DIRECTION('',(0.,-1.,0.)) ;
#33174=DIRECTION('',(0.,-1.,0.)) ;
#33175=DIRECTION('',(-1.,0.,0.)) ;
#33176=DIRECTION('center_axis',(0.,0.,-1.)) ;
#33177=DIRECTION('ref_axis',(1.,0.,0.)) ;
#33178=DIRECTION('',(1.,0.,0.)) ;
#33179=DIRECTION('',(0.,-1.,0.)) ;
#33180=DIRECTION('',(-1.,0.,0.)) ;
#33181=DIRECTION('',(0.,1.,0.)) ;
#33182=DIRECTION('',(1.,0.,0.)) ;
#33183=DIRECTION('',(0.,-1.,0.)) ;
#33184=DIRECTION('',(-1.,0.,0.)) ;
#33185=DIRECTION('',(0.,1.,0.)) ;
#33186=DIRECTION('',(1.,0.,0.)) ;
#33187=DIRECTION('',(0.,-1.,0.)) ;
#33188=DIRECTION('',(-1.,0.,0.)) ;
#33189=DIRECTION('',(0.,1.,0.)) ;
#33190=DIRECTION('',(1.,0.,0.)) ;
#33191=DIRECTION('',(0.,-1.,0.)) ;
#33192=DIRECTION('',(-1.,0.,0.)) ;
#33193=DIRECTION('',(0.,1.,0.)) ;
#33194=DIRECTION('',(1.,0.,0.)) ;
#33195=DIRECTION('',(0.,-1.,0.)) ;
#33196=DIRECTION('',(-1.,0.,0.)) ;
#33197=DIRECTION('',(0.,1.,0.)) ;
#33198=DIRECTION('',(1.,0.,0.)) ;
#33199=DIRECTION('',(0.,-1.,0.)) ;
#33200=DIRECTION('',(-1.,0.,0.)) ;
#33201=DIRECTION('',(0.,1.,0.)) ;
#33202=DIRECTION('',(1.,0.,0.)) ;
#33203=DIRECTION('',(0.,1.,0.)) ;
#33204=DIRECTION('',(1.,0.,0.)) ;
#33205=DIRECTION('center_axis',(0.,0.,-1.)) ;
#33206=DIRECTION('ref_axis',(1.,0.,0.)) ;
#33207=DIRECTION('',(0.,-1.,0.)) ;
#33208=DIRECTION('',(-1.,0.,0.)) ;
#33209=DIRECTION('',(0.,1.,0.)) ;
#33210=DIRECTION('',(1.,0.,0.)) ;
#33211=DIRECTION('center_axis',(0.,0.,-1.)) ;
#33212=DIRECTION('ref_axis',(1.,0.,0.)) ;
#33213=DIRECTION('',(0.,1.,0.)) ;
#33214=DIRECTION('',(1.,0.,0.)) ;
#33215=DIRECTION('',(0.,-1.,0.)) ;
#33216=DIRECTION('',(1.,0.,0.)) ;
#33217=DIRECTION('',(0.,-1.,0.)) ;
#33218=DIRECTION('',(-1.,0.,0.)) ;
#33219=DIRECTION('',(0.,1.,0.)) ;
#33220=DIRECTION('',(0.,-1.,0.)) ;
#33221=DIRECTION('',(-1.,0.,0.)) ;
#33222=DIRECTION('',(0.,1.,0.)) ;
#33223=DIRECTION('',(1.,0.,0.)) ;
#33224=DIRECTION('',(0.,-1.,0.)) ;
#33225=DIRECTION('',(-1.,0.,0.)) ;
#33226=DIRECTION('',(0.,1.,0.)) ;
#33227=DIRECTION('',(1.,0.,0.)) ;
#33228=DIRECTION('',(0.,-1.,0.)) ;
#33229=DIRECTION('',(-1.,0.,0.)) ;
#33230=DIRECTION('',(0.,1.,0.)) ;
#33231=DIRECTION('',(1.,0.,0.)) ;
#33232=DIRECTION('',(0.,-1.,0.)) ;
#33233=DIRECTION('',(-1.,0.,0.)) ;
#33234=DIRECTION('',(0.,1.,0.)) ;
#33235=DIRECTION('',(1.,0.,0.)) ;
#33236=DIRECTION('',(0.,-1.,0.)) ;
#33237=DIRECTION('',(-1.,0.,0.)) ;
#33238=DIRECTION('',(0.,1.,0.)) ;
#33239=DIRECTION('',(1.,0.,0.)) ;
#33240=DIRECTION('',(0.,-1.,0.)) ;
#33241=DIRECTION('',(-1.,0.,0.)) ;
#33242=DIRECTION('',(0.,1.,0.)) ;
#33243=DIRECTION('',(1.,0.,0.)) ;
#33244=DIRECTION('',(0.,-1.,0.)) ;
#33245=DIRECTION('',(-1.,0.,0.)) ;
#33246=DIRECTION('',(0.,1.,0.)) ;
#33247=DIRECTION('',(1.,0.,0.)) ;
#33248=DIRECTION('',(0.,-1.,0.)) ;
#33249=DIRECTION('',(-1.,0.,0.)) ;
#33250=DIRECTION('',(0.,1.,0.)) ;
#33251=DIRECTION('',(1.,0.,0.)) ;
#33252=DIRECTION('center_axis',(0.,0.,-1.)) ;
#33253=DIRECTION('ref_axis',(1.,0.,0.)) ;
#33254=DIRECTION('',(-1.,0.,0.)) ;
#33255=DIRECTION('',(0.,1.,0.)) ;
#33256=DIRECTION('',(1.,0.,0.)) ;
#33257=DIRECTION('center_axis',(0.,0.,1.)) ;
#33258=DIRECTION('ref_axis',(1.,0.,0.)) ;
#33259=DIRECTION('center_axis',(0.,0.,1.)) ;
#33260=DIRECTION('ref_axis',(1.,0.,0.)) ;
#33261=DIRECTION('',(0.,0.,1.)) ;
#33262=DIRECTION('center_axis',(0.,0.,-1.)) ;
#33263=DIRECTION('ref_axis',(-1.,0.,0.)) ;
#33264=DIRECTION('',(1.,0.,0.)) ;
#33265=DIRECTION('',(0.,-1.,0.)) ;
#33266=DIRECTION('center_axis',(0.,0.,-1.)) ;
#33267=DIRECTION('ref_axis',(1.,0.,0.)) ;
#33268=DIRECTION('',(1.,0.,0.)) ;
#33269=DIRECTION('',(0.,-1.,0.)) ;
#33270=DIRECTION('center_axis',(0.,0.,-1.)) ;
#33271=DIRECTION('ref_axis',(1.,0.,0.)) ;
#33272=DIRECTION('',(1.,0.,0.)) ;
#33273=DIRECTION('',(0.,-1.,0.)) ;
#33274=DIRECTION('',(-1.,0.,0.)) ;
#33275=DIRECTION('center_axis',(0.,0.,-1.)) ;
#33276=DIRECTION('ref_axis',(1.,0.,0.)) ;
#33277=DIRECTION('',(0.,-1.,0.)) ;
#33278=DIRECTION('',(-1.,0.,0.)) ;
#33279=DIRECTION('center_axis',(0.,0.,-1.)) ;
#33280=DIRECTION('ref_axis',(1.,0.,0.)) ;
#33281=DIRECTION('',(0.,-1.,0.)) ;
#33282=DIRECTION('',(-1.,0.,0.)) ;
#33283=DIRECTION('center_axis',(0.,0.,-1.)) ;
#33284=DIRECTION('ref_axis',(1.,0.,0.)) ;
#33285=DIRECTION('center_axis',(0.,0.,-1.)) ;
#33286=DIRECTION('ref_axis',(1.,0.,0.)) ;
#33287=DIRECTION('',(0.,-1.,0.)) ;
#33288=DIRECTION('',(-1.,0.,0.)) ;
#33289=DIRECTION('center_axis',(0.,0.,-1.)) ;
#33290=DIRECTION('ref_axis',(1.,0.,0.)) ;
#33291=DIRECTION('',(0.,-1.,0.)) ;
#33292=DIRECTION('',(-1.,0.,0.)) ;
#33293=DIRECTION('center_axis',(0.,0.,-1.)) ;
#33294=DIRECTION('ref_axis',(1.,0.,0.)) ;
#33295=DIRECTION('',(0.,-1.,0.)) ;
#33296=DIRECTION('',(-1.,0.,0.)) ;
#33297=DIRECTION('center_axis',(0.,0.,-1.)) ;
#33298=DIRECTION('ref_axis',(1.,0.,0.)) ;
#33299=DIRECTION('',(0.,-1.,0.)) ;
#33300=DIRECTION('',(-1.,0.,0.)) ;
#33301=DIRECTION('',(0.,1.,0.)) ;
#33302=DIRECTION('center_axis',(0.,0.,-1.)) ;
#33303=DIRECTION('ref_axis',(1.,0.,0.)) ;
#33304=DIRECTION('',(-1.,0.,0.)) ;
#33305=DIRECTION('',(0.,1.,0.)) ;
#33306=DIRECTION('center_axis',(0.,0.,-1.)) ;
#33307=DIRECTION('ref_axis',(1.,0.,0.)) ;
#33308=DIRECTION('',(-1.,0.,0.)) ;
#33309=DIRECTION('',(0.,1.,0.)) ;
#33310=DIRECTION('center_axis',(0.,0.,-1.)) ;
#33311=DIRECTION('ref_axis',(1.,0.,0.)) ;
#33312=DIRECTION('',(-1.,0.,0.)) ;
#33313=DIRECTION('',(0.,1.,0.)) ;
#33314=DIRECTION('center_axis',(0.,0.,-1.)) ;
#33315=DIRECTION('ref_axis',(1.,0.,0.)) ;
#33316=DIRECTION('',(-1.,0.,0.)) ;
#33317=DIRECTION('',(0.,1.,0.)) ;
#33318=DIRECTION('center_axis',(0.,0.,-1.)) ;
#33319=DIRECTION('ref_axis',(1.,0.,0.)) ;
#33320=DIRECTION('',(-1.,0.,0.)) ;
#33321=DIRECTION('',(0.,1.,0.)) ;
#33322=DIRECTION('center_axis',(0.,0.,-1.)) ;
#33323=DIRECTION('ref_axis',(1.,0.,0.)) ;
#33324=DIRECTION('',(-1.,0.,0.)) ;
#33325=DIRECTION('',(0.,1.,0.)) ;
#33326=DIRECTION('center_axis',(0.,0.,-1.)) ;
#33327=DIRECTION('ref_axis',(1.,0.,0.)) ;
#33328=DIRECTION('',(-1.,0.,0.)) ;
#33329=DIRECTION('',(0.,1.,0.)) ;
#33330=DIRECTION('',(1.,0.,0.)) ;
#33331=DIRECTION('center_axis',(0.,0.,-1.)) ;
#33332=DIRECTION('ref_axis',(1.,0.,0.)) ;
#33333=DIRECTION('',(0.,1.,0.)) ;
#33334=DIRECTION('',(1.,0.,0.)) ;
#33335=DIRECTION('center_axis',(0.,0.,-1.)) ;
#33336=DIRECTION('ref_axis',(1.,0.,0.)) ;
#33337=DIRECTION('',(0.,1.,0.)) ;
#33338=DIRECTION('',(1.,0.,0.)) ;
#33339=DIRECTION('center_axis',(0.,0.,-1.)) ;
#33340=DIRECTION('ref_axis',(1.,0.,0.)) ;
#33341=DIRECTION('',(0.,1.,0.)) ;
#33342=DIRECTION('',(1.,0.,0.)) ;
#33343=DIRECTION('center_axis',(0.,0.,-1.)) ;
#33344=DIRECTION('ref_axis',(1.,0.,0.)) ;
#33345=DIRECTION('',(0.,1.,0.)) ;
#33346=DIRECTION('',(1.,0.,0.)) ;
#33347=DIRECTION('center_axis',(0.,0.,-1.)) ;
#33348=DIRECTION('ref_axis',(1.,0.,0.)) ;
#33349=DIRECTION('',(0.,1.,0.)) ;
#33350=DIRECTION('',(1.,0.,0.)) ;
#33351=DIRECTION('center_axis',(0.,0.,-1.)) ;
#33352=DIRECTION('ref_axis',(1.,0.,0.)) ;
#33353=DIRECTION('',(0.,1.,0.)) ;
#33354=DIRECTION('',(1.,0.,0.)) ;
#33355=DIRECTION('center_axis',(0.,0.,-1.)) ;
#33356=DIRECTION('ref_axis',(1.,0.,0.)) ;
#33357=DIRECTION('',(0.,1.,0.)) ;
#33358=DIRECTION('',(1.,0.,0.)) ;
#33359=DIRECTION('',(0.,-1.,0.)) ;
#33360=DIRECTION('center_axis',(0.,0.,-1.)) ;
#33361=DIRECTION('ref_axis',(1.,0.,0.)) ;
#33362=DIRECTION('',(1.,0.,0.)) ;
#33363=DIRECTION('',(0.,-1.,0.)) ;
#33364=DIRECTION('center_axis',(0.,0.,-1.)) ;
#33365=DIRECTION('ref_axis',(1.,0.,0.)) ;
#33366=DIRECTION('',(1.,0.,0.)) ;
#33367=DIRECTION('',(0.,-1.,0.)) ;
#33368=DIRECTION('center_axis',(0.,0.,-1.)) ;
#33369=DIRECTION('ref_axis',(1.,0.,0.)) ;
#33370=DIRECTION('',(1.,0.,0.)) ;
#33371=DIRECTION('',(0.,-1.,0.)) ;
#33372=DIRECTION('',(-1.,0.,0.)) ;
#33373=DIRECTION('',(0.,-1.,0.)) ;
#33374=DIRECTION('',(-1.,0.,0.)) ;
#33375=DIRECTION('',(0.,-1.,0.)) ;
#33376=DIRECTION('',(-1.,0.,0.)) ;
#33377=DIRECTION('',(0.,-1.,0.)) ;
#33378=DIRECTION('',(-1.,0.,0.)) ;
#33379=DIRECTION('',(0.,-1.,0.)) ;
#33380=DIRECTION('center_axis',(0.,0.,1.)) ;
#33381=DIRECTION('ref_axis',(1.,0.,0.)) ;
#33382=DIRECTION('',(-1.,0.,0.)) ;
#33383=DIRECTION('',(0.,-1.,0.)) ;
#33384=DIRECTION('',(1.,0.,0.)) ;
#33385=DIRECTION('center_axis',(0.,0.,1.)) ;
#33386=DIRECTION('ref_axis',(1.,0.,0.)) ;
#33387=DIRECTION('',(1.,0.,0.)) ;
#33388=DIRECTION('center_axis',(0.,0.,1.)) ;
#33389=DIRECTION('ref_axis',(1.,0.,0.)) ;
#33390=DIRECTION('center_axis',(0.,0.,1.)) ;
#33391=DIRECTION('ref_axis',(1.,0.,0.)) ;
#33392=DIRECTION('',(-1.,0.,0.)) ;
#33393=DIRECTION('',(0.,-1.,0.)) ;
#33394=DIRECTION('',(1.,0.,0.)) ;
#33395=DIRECTION('',(1.,0.,0.)) ;
#33396=DIRECTION('',(-1.,0.,0.)) ;
#33397=DIRECTION('center_axis',(0.,0.,1.)) ;
#33398=DIRECTION('ref_axis',(1.,0.,0.)) ;
#33399=DIRECTION('',(0.,-1.,0.)) ;
#33400=DIRECTION('',(1.,0.,0.)) ;
#33401=DIRECTION('',(0.,1.,0.)) ;
#33402=DIRECTION('',(0.,-1.,0.)) ;
#33403=DIRECTION('',(1.,0.,0.)) ;
#33404=DIRECTION('',(0.,1.,0.)) ;
#33405=DIRECTION('',(-1.,0.,0.)) ;
#33406=DIRECTION('',(-1.,0.,0.)) ;
#33407=DIRECTION('',(0.,-1.,0.)) ;
#33408=DIRECTION('',(1.,0.,0.)) ;
#33409=DIRECTION('',(0.,1.,0.)) ;
#33410=DIRECTION('',(-1.,0.,0.)) ;
#33411=DIRECTION('',(0.,-1.,0.)) ;
#33412=DIRECTION('',(1.,0.,0.)) ;
#33413=DIRECTION('',(0.,1.,0.)) ;
#33414=DIRECTION('',(-1.,0.,0.)) ;
#33415=DIRECTION('',(0.,-1.,0.)) ;
#33416=DIRECTION('',(1.,0.,0.)) ;
#33417=DIRECTION('',(0.,1.,0.)) ;
#33418=DIRECTION('',(0.,1.,0.)) ;
#33419=DIRECTION('center_axis',(0.,0.,1.)) ;
#33420=DIRECTION('ref_axis',(1.,0.,0.)) ;
#33421=DIRECTION('',(1.,0.,0.)) ;
#33422=DIRECTION('',(-1.,0.,0.)) ;
#33423=DIRECTION('',(0.,-1.,0.)) ;
#33424=DIRECTION('',(1.,0.,0.)) ;
#33425=DIRECTION('',(0.,1.,0.)) ;
#33426=DIRECTION('',(-1.,0.,0.)) ;
#33427=DIRECTION('',(0.,-1.,0.)) ;
#33428=DIRECTION('',(1.,0.,0.)) ;
#33429=DIRECTION('',(0.,1.,0.)) ;
#33430=DIRECTION('',(-1.,0.,0.)) ;
#33431=DIRECTION('',(0.,-1.,0.)) ;
#33432=DIRECTION('',(1.,0.,0.)) ;
#33433=DIRECTION('',(0.,1.,0.)) ;
#33434=DIRECTION('',(-1.,0.,0.)) ;
#33435=DIRECTION('',(0.,-1.,0.)) ;
#33436=DIRECTION('',(1.,0.,0.)) ;
#33437=DIRECTION('',(0.,1.,0.)) ;
#33438=DIRECTION('',(-1.,0.,0.)) ;
#33439=DIRECTION('',(0.,-1.,0.)) ;
#33440=DIRECTION('',(1.,0.,0.)) ;
#33441=DIRECTION('',(0.,1.,0.)) ;
#33442=DIRECTION('',(-1.,0.,0.)) ;
#33443=DIRECTION('',(0.,-1.,0.)) ;
#33444=DIRECTION('',(1.,0.,0.)) ;
#33445=DIRECTION('',(0.,1.,0.)) ;
#33446=DIRECTION('',(0.,1.,0.)) ;
#33447=DIRECTION('',(-1.,0.,0.)) ;
#33448=DIRECTION('',(0.,-1.,0.)) ;
#33449=DIRECTION('center_axis',(0.,0.,1.)) ;
#33450=DIRECTION('ref_axis',(1.,0.,0.)) ;
#33451=DIRECTION('',(-1.,0.,0.)) ;
#33452=DIRECTION('center_axis',(0.,0.,1.)) ;
#33453=DIRECTION('ref_axis',(1.,0.,0.)) ;
#33454=DIRECTION('',(1.,0.,0.)) ;
#33455=DIRECTION('',(0.,1.,0.)) ;
#33456=DIRECTION('',(-1.,0.,0.)) ;
#33457=DIRECTION('',(0.,-1.,0.)) ;
#33458=DIRECTION('center_axis',(0.,0.,1.)) ;
#33459=DIRECTION('ref_axis',(1.,0.,0.)) ;
#33460=DIRECTION('',(1.,0.,0.)) ;
#33461=DIRECTION('',(0.,1.,0.)) ;
#33462=DIRECTION('',(-1.,0.,0.)) ;
#33463=DIRECTION('center_axis',(0.,0.,1.)) ;
#33464=DIRECTION('ref_axis',(1.,0.,0.)) ;
#33465=DIRECTION('',(0.,1.,0.)) ;
#33466=DIRECTION('',(-1.,0.,0.)) ;
#33467=DIRECTION('',(0.,-1.,0.)) ;
#33468=DIRECTION('',(1.,0.,0.)) ;
#33469=DIRECTION('',(0.,1.,0.)) ;
#33470=DIRECTION('',(-1.,0.,0.)) ;
#33471=DIRECTION('center_axis',(0.,0.,1.)) ;
#33472=DIRECTION('ref_axis',(1.,0.,0.)) ;
#33473=DIRECTION('',(0.,1.,0.)) ;
#33474=DIRECTION('',(-1.,0.,0.)) ;
#33475=DIRECTION('',(0.,-1.,0.)) ;
#33476=DIRECTION('',(1.,0.,0.)) ;
#33477=DIRECTION('',(0.,1.,0.)) ;
#33478=DIRECTION('',(-1.,0.,0.)) ;
#33479=DIRECTION('',(0.,-1.,0.)) ;
#33480=DIRECTION('',(1.,0.,0.)) ;
#33481=DIRECTION('',(0.,1.,0.)) ;
#33482=DIRECTION('',(-1.,0.,0.)) ;
#33483=DIRECTION('',(0.,-1.,0.)) ;
#33484=DIRECTION('',(1.,0.,0.)) ;
#33485=DIRECTION('',(0.,1.,0.)) ;
#33486=DIRECTION('',(-1.,0.,0.)) ;
#33487=DIRECTION('',(0.,-1.,0.)) ;
#33488=DIRECTION('',(1.,0.,0.)) ;
#33489=DIRECTION('',(0.,1.,0.)) ;
#33490=DIRECTION('',(-1.,0.,0.)) ;
#33491=DIRECTION('center_axis',(0.,0.,1.)) ;
#33492=DIRECTION('ref_axis',(1.,0.,0.)) ;
#33493=DIRECTION('',(1.,0.,0.)) ;
#33494=DIRECTION('',(0.,1.,0.)) ;
#33495=DIRECTION('',(0.,1.,0.)) ;
#33496=DIRECTION('',(-1.,0.,0.)) ;
#33497=DIRECTION('',(0.,-1.,0.)) ;
#33498=DIRECTION('center_axis',(0.,0.,1.)) ;
#33499=DIRECTION('ref_axis',(1.,0.,0.)) ;
#33500=DIRECTION('',(-1.,0.,0.)) ;
#33501=DIRECTION('',(0.,-1.,0.)) ;
#33502=DIRECTION('',(1.,0.,0.)) ;
#33503=DIRECTION('',(0.,1.,0.)) ;
#33504=DIRECTION('',(-1.,0.,0.)) ;
#33505=DIRECTION('',(0.,-1.,0.)) ;
#33506=DIRECTION('',(1.,0.,0.)) ;
#33507=DIRECTION('',(0.,1.,0.)) ;
#33508=DIRECTION('',(-1.,0.,0.)) ;
#33509=DIRECTION('',(0.,-1.,0.)) ;
#33510=DIRECTION('',(1.,0.,0.)) ;
#33511=DIRECTION('',(0.,1.,0.)) ;
#33512=DIRECTION('center_axis',(0.,0.,1.)) ;
#33513=DIRECTION('ref_axis',(1.,0.,0.)) ;
#33514=DIRECTION('',(-1.,0.,0.)) ;
#33515=DIRECTION('',(0.,-1.,0.)) ;
#33516=DIRECTION('',(-1.,0.,0.)) ;
#33517=DIRECTION('',(0.,-1.,0.)) ;
#33518=DIRECTION('',(1.,0.,0.)) ;
#33519=DIRECTION('',(0.,1.,0.)) ;
#33520=DIRECTION('',(-1.,0.,0.)) ;
#33521=DIRECTION('',(0.,-1.,0.)) ;
#33522=DIRECTION('',(1.,0.,0.)) ;
#33523=DIRECTION('',(0.,1.,0.)) ;
#33524=DIRECTION('',(-1.,0.,0.)) ;
#33525=DIRECTION('',(0.,-1.,0.)) ;
#33526=DIRECTION('',(1.,0.,0.)) ;
#33527=DIRECTION('',(0.,1.,0.)) ;
#33528=DIRECTION('',(-1.,0.,0.)) ;
#33529=DIRECTION('',(0.,-1.,0.)) ;
#33530=DIRECTION('',(1.,0.,0.)) ;
#33531=DIRECTION('',(0.,1.,0.)) ;
#33532=DIRECTION('',(-1.,0.,0.)) ;
#33533=DIRECTION('',(0.,-1.,0.)) ;
#33534=DIRECTION('',(1.,0.,0.)) ;
#33535=DIRECTION('',(0.,1.,0.)) ;
#33536=DIRECTION('',(-1.,0.,0.)) ;
#33537=DIRECTION('',(0.,-1.,0.)) ;
#33538=DIRECTION('',(1.,0.,0.)) ;
#33539=DIRECTION('',(0.,1.,0.)) ;
#33540=DIRECTION('',(-1.,0.,0.)) ;
#33541=DIRECTION('',(0.,-1.,0.)) ;
#33542=DIRECTION('',(1.,0.,0.)) ;
#33543=DIRECTION('',(0.,1.,0.)) ;
#33544=DIRECTION('',(-1.,0.,0.)) ;
#33545=DIRECTION('',(0.,-1.,0.)) ;
#33546=DIRECTION('',(1.,0.,0.)) ;
#33547=DIRECTION('',(0.,1.,0.)) ;
#33548=DIRECTION('',(-1.,0.,0.)) ;
#33549=DIRECTION('',(0.,-1.,0.)) ;
#33550=DIRECTION('',(1.,0.,0.)) ;
#33551=DIRECTION('',(0.,1.,0.)) ;
#33552=DIRECTION('',(1.,0.,0.)) ;
#33553=DIRECTION('center_axis',(0.,0.,1.)) ;
#33554=DIRECTION('ref_axis',(1.,0.,0.)) ;
#33555=DIRECTION('',(0.,-1.,0.)) ;
#33556=DIRECTION('',(0.,1.,0.)) ;
#33557=DIRECTION('center_axis',(0.,0.,1.)) ;
#33558=DIRECTION('ref_axis',(1.,0.,0.)) ;
#33559=DIRECTION('',(1.,0.,0.)) ;
#33560=DIRECTION('',(0.,1.,0.)) ;
#33561=DIRECTION('center_axis',(0.,0.,1.)) ;
#33562=DIRECTION('ref_axis',(1.,0.,0.)) ;
#33563=DIRECTION('',(0.,-1.,0.)) ;
#33564=DIRECTION('',(1.,0.,0.)) ;
#33565=DIRECTION('',(0.,1.,0.)) ;
#33566=DIRECTION('center_axis',(0.,0.,1.)) ;
#33567=DIRECTION('ref_axis',(1.,0.,0.)) ;
#33568=DIRECTION('',(0.,-1.,0.)) ;
#33569=DIRECTION('',(1.,0.,0.)) ;
#33570=DIRECTION('',(0.,-1.,0.)) ;
#33571=DIRECTION('',(1.,0.,0.)) ;
#33572=DIRECTION('',(0.,1.,0.)) ;
#33573=DIRECTION('',(-1.,0.,0.)) ;
#33574=DIRECTION('center_axis',(0.,0.,1.)) ;
#33575=DIRECTION('ref_axis',(1.,0.,0.)) ;
#33576=DIRECTION('',(0.,0.,-1.)) ;
#33577=DIRECTION('center_axis',(0.,0.,1.)) ;
#33578=DIRECTION('ref_axis',(1.,0.,0.)) ;
#33579=DIRECTION('',(0.,0.,1.)) ;
#33580=DIRECTION('center_axis',(-1.,0.,0.)) ;
#33581=DIRECTION('ref_axis',(0.,0.,1.)) ;
#33582=DIRECTION('',(0.,0.,-1.)) ;
#33583=DIRECTION('center_axis',(0.,1.,0.)) ;
#33584=DIRECTION('ref_axis',(0.,0.,1.)) ;
#33585=DIRECTION('',(0.,0.,-1.)) ;
#33586=DIRECTION('',(0.,0.,1.)) ;
#33587=DIRECTION('center_axis',(0.,1.,0.)) ;
#33588=DIRECTION('ref_axis',(0.,0.,1.)) ;
#33589=DIRECTION('',(0.,0.,-1.)) ;
#33590=DIRECTION('',(0.,0.,1.)) ;
#33591=DIRECTION('center_axis',(0.,1.,0.)) ;
#33592=DIRECTION('ref_axis',(0.,0.,1.)) ;
#33593=DIRECTION('',(0.,0.,-1.)) ;
#33594=DIRECTION('',(0.,0.,1.)) ;
#33595=DIRECTION('center_axis',(0.,1.,0.)) ;
#33596=DIRECTION('ref_axis',(0.,0.,1.)) ;
#33597=DIRECTION('',(0.,0.,1.)) ;
#33598=DIRECTION('',(0.,0.,-1.)) ;
#33599=DIRECTION('center_axis',(0.,1.,0.)) ;
#33600=DIRECTION('ref_axis',(0.,0.,1.)) ;
#33601=DIRECTION('',(0.,0.,1.)) ;
#33602=DIRECTION('',(0.,0.,-1.)) ;
#33603=DIRECTION('center_axis',(0.,1.,0.)) ;
#33604=DIRECTION('ref_axis',(0.,0.,1.)) ;
#33605=DIRECTION('',(0.,0.,-1.)) ;
#33606=DIRECTION('',(0.,0.,1.)) ;
#33607=DIRECTION('center_axis',(0.,-1.,0.)) ;
#33608=DIRECTION('ref_axis',(0.,0.,-1.)) ;
#33609=DIRECTION('',(0.,0.,1.)) ;
#33610=DIRECTION('',(0.,0.,-1.)) ;
#33611=DIRECTION('center_axis',(0.,-1.,0.)) ;
#33612=DIRECTION('ref_axis',(0.,0.,-1.)) ;
#33613=DIRECTION('',(0.,0.,1.)) ;
#33614=DIRECTION('',(0.,0.,-1.)) ;
#33615=DIRECTION('center_axis',(0.,-1.,0.)) ;
#33616=DIRECTION('ref_axis',(0.,0.,-1.)) ;
#33617=DIRECTION('',(0.,0.,1.)) ;
#33618=DIRECTION('',(0.,0.,-1.)) ;
#33619=DIRECTION('center_axis',(0.,-1.,0.)) ;
#33620=DIRECTION('ref_axis',(0.,0.,-1.)) ;
#33621=DIRECTION('',(0.,0.,1.)) ;
#33622=DIRECTION('',(0.,0.,-1.)) ;
#33623=DIRECTION('center_axis',(0.,-1.,0.)) ;
#33624=DIRECTION('ref_axis',(0.,0.,-1.)) ;
#33625=DIRECTION('',(0.,0.,-1.)) ;
#33626=DIRECTION('center_axis',(1.,0.,0.)) ;
#33627=DIRECTION('ref_axis',(0.,0.,-1.)) ;
#33628=DIRECTION('',(0.,0.,-1.)) ;
#33629=DIRECTION('center_axis',(0.,-1.,0.)) ;
#33630=DIRECTION('ref_axis',(0.,0.,-1.)) ;
#33631=DIRECTION('',(0.,0.,-1.)) ;
#33632=DIRECTION('',(0.,0.,1.)) ;
#33633=DIRECTION('center_axis',(-1.,0.,0.)) ;
#33634=DIRECTION('ref_axis',(0.,0.,1.)) ;
#33635=DIRECTION('',(0.,0.,-1.)) ;
#33636=DIRECTION('center_axis',(1.,0.,0.)) ;
#33637=DIRECTION('ref_axis',(0.,0.,-1.)) ;
#33638=DIRECTION('',(0.,0.,1.)) ;
#33639=DIRECTION('center_axis',(1.,0.,0.)) ;
#33640=DIRECTION('ref_axis',(0.,0.,-1.)) ;
#33641=DIRECTION('',(0.,0.,-1.)) ;
#33642=DIRECTION('center_axis',(0.,0.,1.)) ;
#33643=DIRECTION('ref_axis',(1.,0.,0.)) ;
#33644=DIRECTION('center_axis',(0.,0.,1.)) ;
#33645=DIRECTION('ref_axis',(1.,0.,0.)) ;
#33646=DIRECTION('',(0.,0.,1.)) ;
#33647=DIRECTION('center_axis',(-1.,0.,0.)) ;
#33648=DIRECTION('ref_axis',(0.,0.,1.)) ;
#33649=DIRECTION('',(0.,0.,-1.)) ;
#33650=DIRECTION('center_axis',(1.,0.,0.)) ;
#33651=DIRECTION('ref_axis',(0.,0.,-1.)) ;
#33652=DIRECTION('',(0.,0.,1.)) ;
#33653=DIRECTION('center_axis',(-1.,0.,0.)) ;
#33654=DIRECTION('ref_axis',(0.,0.,1.)) ;
#33655=DIRECTION('',(0.,0.,-1.)) ;
#33656=DIRECTION('center_axis',(1.,0.,0.)) ;
#33657=DIRECTION('ref_axis',(0.,0.,-1.)) ;
#33658=DIRECTION('',(0.,0.,1.)) ;
#33659=DIRECTION('center_axis',(1.,0.,0.)) ;
#33660=DIRECTION('ref_axis',(0.,0.,-1.)) ;
#33661=DIRECTION('',(0.,0.,1.)) ;
#33662=DIRECTION('center_axis',(0.,0.,1.)) ;
#33663=DIRECTION('ref_axis',(1.,0.,0.)) ;
#33664=DIRECTION('',(0.,0.,1.)) ;
#33665=DIRECTION('center_axis',(0.,0.,1.)) ;
#33666=DIRECTION('ref_axis',(1.,0.,0.)) ;
#33667=DIRECTION('',(0.,0.,-1.)) ;
#33668=DIRECTION('center_axis',(0.,0.,1.)) ;
#33669=DIRECTION('ref_axis',(1.,0.,0.)) ;
#33670=DIRECTION('',(0.,0.,1.)) ;
#33671=DIRECTION('center_axis',(0.,1.,0.)) ;
#33672=DIRECTION('ref_axis',(0.,0.,1.)) ;
#33673=DIRECTION('',(0.,0.,1.)) ;
#33674=DIRECTION('',(0.,0.,-1.)) ;
#33675=DIRECTION('center_axis',(-1.,0.,0.)) ;
#33676=DIRECTION('ref_axis',(0.,0.,1.)) ;
#33677=DIRECTION('',(0.,0.,-1.)) ;
#33678=DIRECTION('center_axis',(-1.,0.,0.)) ;
#33679=DIRECTION('ref_axis',(0.,0.,1.)) ;
#33680=DIRECTION('',(0.,0.,-1.)) ;
#33681=DIRECTION('center_axis',(-1.,0.,0.)) ;
#33682=DIRECTION('ref_axis',(0.,0.,1.)) ;
#33683=DIRECTION('',(0.,0.,-1.)) ;
#33684=DIRECTION('',(0.,0.,1.)) ;
#33685=DIRECTION('center_axis',(-1.,0.,0.)) ;
#33686=DIRECTION('ref_axis',(0.,0.,1.)) ;
#33687=DIRECTION('',(0.,0.,-1.)) ;
#33688=DIRECTION('center_axis',(-1.,0.,0.)) ;
#33689=DIRECTION('ref_axis',(0.,0.,1.)) ;
#33690=DIRECTION('',(0.,0.,-1.)) ;
#33691=DIRECTION('center_axis',(-1.,0.,0.)) ;
#33692=DIRECTION('ref_axis',(0.,0.,1.)) ;
#33693=DIRECTION('',(0.,0.,-1.)) ;
#33694=DIRECTION('center_axis',(-1.,0.,0.)) ;
#33695=DIRECTION('ref_axis',(0.,0.,1.)) ;
#33696=DIRECTION('center_axis',(1.,0.,0.)) ;
#33697=DIRECTION('ref_axis',(0.,0.,-1.)) ;
#33698=DIRECTION('',(0.,0.,1.)) ;
#33699=DIRECTION('',(0.,0.,-1.)) ;
#33700=DIRECTION('center_axis',(1.,0.,0.)) ;
#33701=DIRECTION('ref_axis',(0.,0.,-1.)) ;
#33702=DIRECTION('',(0.,0.,1.)) ;
#33703=DIRECTION('',(0.,0.,-1.)) ;
#33704=DIRECTION('center_axis',(1.,0.,0.)) ;
#33705=DIRECTION('ref_axis',(0.,0.,-1.)) ;
#33706=DIRECTION('',(0.,0.,1.)) ;
#33707=DIRECTION('',(0.,0.,-1.)) ;
#33708=DIRECTION('center_axis',(1.,0.,0.)) ;
#33709=DIRECTION('ref_axis',(0.,0.,-1.)) ;
#33710=DIRECTION('',(0.,0.,1.)) ;
#33711=DIRECTION('',(0.,0.,-1.)) ;
#33712=DIRECTION('center_axis',(1.,0.,0.)) ;
#33713=DIRECTION('ref_axis',(0.,0.,-1.)) ;
#33714=DIRECTION('',(0.,0.,1.)) ;
#33715=DIRECTION('',(0.,0.,-1.)) ;
#33716=DIRECTION('center_axis',(0.,-1.,0.)) ;
#33717=DIRECTION('ref_axis',(0.,0.,-1.)) ;
#33718=DIRECTION('',(0.,0.,-1.)) ;
#33719=DIRECTION('center_axis',(-1.,0.,0.)) ;
#33720=DIRECTION('ref_axis',(0.,0.,1.)) ;
#33721=DIRECTION('',(0.,0.,-1.)) ;
#33722=DIRECTION('center_axis',(0.,1.,0.)) ;
#33723=DIRECTION('ref_axis',(0.,0.,1.)) ;
#33724=DIRECTION('center_axis',(0.,-1.,0.)) ;
#33725=DIRECTION('ref_axis',(0.,0.,-1.)) ;
#33726=DIRECTION('',(0.,0.,-1.)) ;
#33727=DIRECTION('center_axis',(0.,0.,1.)) ;
#33728=DIRECTION('ref_axis',(1.,0.,0.)) ;
#33729=DIRECTION('',(0.,0.,1.)) ;
#33730=DIRECTION('center_axis',(0.,1.,0.)) ;
#33731=DIRECTION('ref_axis',(0.,0.,1.)) ;
#33732=DIRECTION('center_axis',(0.,-1.,0.)) ;
#33733=DIRECTION('ref_axis',(0.,0.,-1.)) ;
#33734=DIRECTION('',(0.,0.,1.)) ;
#33735=DIRECTION('center_axis',(0.,1.,0.)) ;
#33736=DIRECTION('ref_axis',(0.,0.,1.)) ;
#33737=DIRECTION('center_axis',(0.,-1.,0.)) ;
#33738=DIRECTION('ref_axis',(0.,0.,-1.)) ;
#33739=DIRECTION('',(0.,0.,1.)) ;
#33740=DIRECTION('center_axis',(0.,1.,0.)) ;
#33741=DIRECTION('ref_axis',(0.,0.,1.)) ;
#33742=DIRECTION('center_axis',(0.,-1.,0.)) ;
#33743=DIRECTION('ref_axis',(0.,0.,-1.)) ;
#33744=DIRECTION('',(0.,0.,1.)) ;
#33745=DIRECTION('center_axis',(0.,1.,0.)) ;
#33746=DIRECTION('ref_axis',(0.,0.,1.)) ;
#33747=DIRECTION('center_axis',(0.,-1.,0.)) ;
#33748=DIRECTION('ref_axis',(0.,0.,-1.)) ;
#33749=DIRECTION('',(0.,0.,1.)) ;
#33750=DIRECTION('center_axis',(0.,0.,1.)) ;
#33751=DIRECTION('ref_axis',(1.,0.,0.)) ;
#33752=DIRECTION('',(0.,0.,1.)) ;
#33753=DIRECTION('center_axis',(0.,-1.,0.)) ;
#33754=DIRECTION('ref_axis',(0.,0.,-1.)) ;
#33755=DIRECTION('',(0.,0.,1.)) ;
#33756=DIRECTION('center_axis',(-1.,0.,0.)) ;
#33757=DIRECTION('ref_axis',(0.,0.,1.)) ;
#33758=DIRECTION('',(0.,0.,1.)) ;
#33759=DIRECTION('',(0.,0.,-1.)) ;
#33760=DIRECTION('center_axis',(0.,-1.,0.)) ;
#33761=DIRECTION('ref_axis',(0.,0.,-1.)) ;
#33762=DIRECTION('',(0.,0.,1.)) ;
#33763=DIRECTION('',(0.,0.,-1.)) ;
#33764=DIRECTION('center_axis',(0.,-1.,0.)) ;
#33765=DIRECTION('ref_axis',(0.,0.,-1.)) ;
#33766=DIRECTION('',(0.,0.,-1.)) ;
#33767=DIRECTION('center_axis',(0.,-1.,0.)) ;
#33768=DIRECTION('ref_axis',(0.,0.,-1.)) ;
#33769=DIRECTION('',(0.,0.,-1.)) ;
#33770=DIRECTION('center_axis',(0.,-1.,0.)) ;
#33771=DIRECTION('ref_axis',(0.,0.,-1.)) ;
#33772=DIRECTION('',(0.,0.,-1.)) ;
#33773=DIRECTION('center_axis',(0.,-1.,0.)) ;
#33774=DIRECTION('ref_axis',(0.,0.,-1.)) ;
#33775=DIRECTION('center_axis',(0.,-1.,0.)) ;
#33776=DIRECTION('ref_axis',(0.,0.,-1.)) ;
#33777=DIRECTION('',(0.,0.,-1.)) ;
#33778=DIRECTION('center_axis',(0.,1.,0.)) ;
#33779=DIRECTION('ref_axis',(0.,0.,1.)) ;
#33780=DIRECTION('',(0.,0.,1.)) ;
#33781=DIRECTION('',(0.,0.,-1.)) ;
#33782=DIRECTION('center_axis',(0.,1.,0.)) ;
#33783=DIRECTION('ref_axis',(0.,0.,1.)) ;
#33784=DIRECTION('',(0.,0.,-1.)) ;
#33785=DIRECTION('',(0.,0.,1.)) ;
#33786=DIRECTION('center_axis',(0.,1.,0.)) ;
#33787=DIRECTION('ref_axis',(0.,0.,1.)) ;
#33788=DIRECTION('',(0.,0.,1.)) ;
#33789=DIRECTION('center_axis',(0.,1.,0.)) ;
#33790=DIRECTION('ref_axis',(0.,0.,1.)) ;
#33791=DIRECTION('',(0.,0.,-1.)) ;
#33792=DIRECTION('',(0.,0.,1.)) ;
#33793=DIRECTION('center_axis',(0.,1.,0.)) ;
#33794=DIRECTION('ref_axis',(0.,0.,1.)) ;
#33795=DIRECTION('',(0.,0.,-1.)) ;
#33796=DIRECTION('',(0.,0.,1.)) ;
#33797=DIRECTION('center_axis',(1.,0.,0.)) ;
#33798=DIRECTION('ref_axis',(0.,0.,-1.)) ;
#33799=DIRECTION('',(0.,0.,-1.)) ;
#33800=DIRECTION('center_axis',(-1.,0.,0.)) ;
#33801=DIRECTION('ref_axis',(0.,0.,1.)) ;
#33802=DIRECTION('center_axis',(1.,0.,0.)) ;
#33803=DIRECTION('ref_axis',(0.,0.,-1.)) ;
#33804=DIRECTION('',(0.,0.,1.)) ;
#33805=DIRECTION('center_axis',(1.,0.,0.)) ;
#33806=DIRECTION('ref_axis',(0.,0.,-1.)) ;
#33807=DIRECTION('',(0.,0.,-1.)) ;
#33808=DIRECTION('center_axis',(-1.,0.,0.)) ;
#33809=DIRECTION('ref_axis',(0.,0.,1.)) ;
#33810=DIRECTION('center_axis',(1.,0.,0.)) ;
#33811=DIRECTION('ref_axis',(0.,0.,-1.)) ;
#33812=DIRECTION('',(0.,0.,1.)) ;
#33813=DIRECTION('center_axis',(0.,0.,1.)) ;
#33814=DIRECTION('ref_axis',(1.,0.,0.)) ;
#33815=DIRECTION('center_axis',(0.,0.,1.)) ;
#33816=DIRECTION('ref_axis',(1.,0.,0.)) ;
#33817=DIRECTION('',(0.,0.,-1.)) ;
#33818=DIRECTION('center_axis',(-1.,0.,0.)) ;
#33819=DIRECTION('ref_axis',(0.,0.,1.)) ;
#33820=DIRECTION('',(0.,0.,-1.)) ;
#33821=DIRECTION('center_axis',(0.,0.,1.)) ;
#33822=DIRECTION('ref_axis',(1.,0.,0.)) ;
#33823=DIRECTION('',(0.,0.,-1.)) ;
#33824=DIRECTION('center_axis',(0.,0.,1.)) ;
#33825=DIRECTION('ref_axis',(1.,0.,0.)) ;
#33826=DIRECTION('',(0.,0.,1.)) ;
#33827=DIRECTION('center_axis',(-1.,0.,0.)) ;
#33828=DIRECTION('ref_axis',(0.,0.,1.)) ;
#33829=DIRECTION('center_axis',(1.,0.,0.)) ;
#33830=DIRECTION('ref_axis',(0.,0.,-1.)) ;
#33831=DIRECTION('',(0.,0.,1.)) ;
#33832=DIRECTION('center_axis',(-1.,0.,0.)) ;
#33833=DIRECTION('ref_axis',(0.,0.,1.)) ;
#33834=DIRECTION('center_axis',(1.,0.,0.)) ;
#33835=DIRECTION('ref_axis',(0.,0.,-1.)) ;
#33836=DIRECTION('',(0.,0.,1.)) ;
#33837=DIRECTION('center_axis',(0.,1.,0.)) ;
#33838=DIRECTION('ref_axis',(0.,0.,1.)) ;
#33839=DIRECTION('',(0.,0.,1.)) ;
#33840=DIRECTION('',(0.,0.,-1.)) ;
#33841=DIRECTION('center_axis',(-1.,0.,0.)) ;
#33842=DIRECTION('ref_axis',(0.,0.,1.)) ;
#33843=DIRECTION('',(0.,0.,-1.)) ;
#33844=DIRECTION('center_axis',(-1.,0.,0.)) ;
#33845=DIRECTION('ref_axis',(0.,0.,1.)) ;
#33846=DIRECTION('',(0.,0.,1.)) ;
#33847=DIRECTION('',(0.,0.,-1.)) ;
#33848=DIRECTION('center_axis',(-1.,0.,0.)) ;
#33849=DIRECTION('ref_axis',(0.,0.,1.)) ;
#33850=DIRECTION('',(0.,0.,-1.)) ;
#33851=DIRECTION('center_axis',(-1.,0.,0.)) ;
#33852=DIRECTION('ref_axis',(0.,0.,1.)) ;
#33853=DIRECTION('',(0.,0.,-1.)) ;
#33854=DIRECTION('center_axis',(-1.,0.,0.)) ;
#33855=DIRECTION('ref_axis',(0.,0.,1.)) ;
#33856=DIRECTION('',(0.,0.,-1.)) ;
#33857=DIRECTION('center_axis',(-1.,0.,0.)) ;
#33858=DIRECTION('ref_axis',(0.,0.,1.)) ;
#33859=DIRECTION('',(0.,0.,-1.)) ;
#33860=DIRECTION('center_axis',(-1.,0.,0.)) ;
#33861=DIRECTION('ref_axis',(0.,0.,1.)) ;
#33862=DIRECTION('center_axis',(1.,0.,0.)) ;
#33863=DIRECTION('ref_axis',(0.,0.,-1.)) ;
#33864=DIRECTION('',(0.,0.,1.)) ;
#33865=DIRECTION('',(0.,0.,-1.)) ;
#33866=DIRECTION('center_axis',(1.,0.,0.)) ;
#33867=DIRECTION('ref_axis',(0.,0.,-1.)) ;
#33868=DIRECTION('',(0.,0.,1.)) ;
#33869=DIRECTION('',(0.,0.,-1.)) ;
#33870=DIRECTION('center_axis',(1.,0.,0.)) ;
#33871=DIRECTION('ref_axis',(0.,0.,-1.)) ;
#33872=DIRECTION('',(0.,0.,1.)) ;
#33873=DIRECTION('',(0.,0.,-1.)) ;
#33874=DIRECTION('center_axis',(1.,0.,0.)) ;
#33875=DIRECTION('ref_axis',(0.,0.,-1.)) ;
#33876=DIRECTION('',(0.,0.,1.)) ;
#33877=DIRECTION('',(0.,0.,-1.)) ;
#33878=DIRECTION('center_axis',(1.,0.,0.)) ;
#33879=DIRECTION('ref_axis',(0.,0.,-1.)) ;
#33880=DIRECTION('',(0.,0.,-1.)) ;
#33881=DIRECTION('',(0.,0.,1.)) ;
#33882=DIRECTION('center_axis',(0.,-1.,0.)) ;
#33883=DIRECTION('ref_axis',(0.,0.,-1.)) ;
#33884=DIRECTION('',(0.,0.,-1.)) ;
#33885=DIRECTION('center_axis',(-1.,0.,0.)) ;
#33886=DIRECTION('ref_axis',(0.,0.,1.)) ;
#33887=DIRECTION('',(0.,0.,-1.)) ;
#33888=DIRECTION('center_axis',(0.,1.,0.)) ;
#33889=DIRECTION('ref_axis',(0.,0.,1.)) ;
#33890=DIRECTION('center_axis',(0.,-1.,0.)) ;
#33891=DIRECTION('ref_axis',(0.,0.,-1.)) ;
#33892=DIRECTION('center_axis',(0.,-1.,0.)) ;
#33893=DIRECTION('ref_axis',(0.,0.,-1.)) ;
#33894=DIRECTION('',(0.,0.,-1.)) ;
#33895=DIRECTION('center_axis',(0.,0.,1.)) ;
#33896=DIRECTION('ref_axis',(1.,0.,0.)) ;
#33897=DIRECTION('',(0.,0.,1.)) ;
#33898=DIRECTION('center_axis',(0.,0.,1.)) ;
#33899=DIRECTION('ref_axis',(1.,0.,0.)) ;
#33900=DIRECTION('center_axis',(0.,0.,1.)) ;
#33901=DIRECTION('ref_axis',(1.,0.,0.)) ;
#33902=DIRECTION('',(0.,0.,-1.)) ;
#33903=DIRECTION('center_axis',(0.,0.,1.)) ;
#33904=DIRECTION('ref_axis',(1.,0.,0.)) ;
#33905=DIRECTION('',(0.,0.,1.)) ;
#33906=DIRECTION('center_axis',(0.,1.,0.)) ;
#33907=DIRECTION('ref_axis',(0.,0.,1.)) ;
#33908=DIRECTION('center_axis',(0.,-1.,0.)) ;
#33909=DIRECTION('ref_axis',(0.,0.,-1.)) ;
#33910=DIRECTION('',(0.,0.,1.)) ;
#33911=DIRECTION('center_axis',(0.,1.,0.)) ;
#33912=DIRECTION('ref_axis',(0.,0.,1.)) ;
#33913=DIRECTION('center_axis',(0.,-1.,0.)) ;
#33914=DIRECTION('ref_axis',(0.,0.,-1.)) ;
#33915=DIRECTION('',(0.,0.,1.)) ;
#33916=DIRECTION('center_axis',(0.,1.,0.)) ;
#33917=DIRECTION('ref_axis',(0.,0.,1.)) ;
#33918=DIRECTION('center_axis',(0.,-1.,0.)) ;
#33919=DIRECTION('ref_axis',(0.,0.,-1.)) ;
#33920=DIRECTION('',(0.,0.,1.)) ;
#33921=DIRECTION('center_axis',(0.,1.,0.)) ;
#33922=DIRECTION('ref_axis',(0.,0.,1.)) ;
#33923=DIRECTION('center_axis',(0.,-1.,0.)) ;
#33924=DIRECTION('ref_axis',(0.,0.,-1.)) ;
#33925=DIRECTION('',(0.,0.,1.)) ;
#33926=DIRECTION('center_axis',(-1.,0.,0.)) ;
#33927=DIRECTION('ref_axis',(0.,0.,1.)) ;
#33928=DIRECTION('',(0.,0.,1.)) ;
#33929=DIRECTION('',(0.,0.,-1.)) ;
#33930=DIRECTION('center_axis',(0.,1.,0.)) ;
#33931=DIRECTION('ref_axis',(0.,0.,1.)) ;
#33932=DIRECTION('',(0.,0.,-1.)) ;
#33933=DIRECTION('',(0.,0.,1.)) ;
#33934=DIRECTION('center_axis',(0.,1.,0.)) ;
#33935=DIRECTION('ref_axis',(0.,0.,1.)) ;
#33936=DIRECTION('',(0.,0.,-1.)) ;
#33937=DIRECTION('',(0.,0.,1.)) ;
#33938=DIRECTION('center_axis',(0.,1.,0.)) ;
#33939=DIRECTION('ref_axis',(0.,0.,1.)) ;
#33940=DIRECTION('',(0.,0.,-1.)) ;
#33941=DIRECTION('',(0.,0.,1.)) ;
#33942=DIRECTION('center_axis',(0.,1.,0.)) ;
#33943=DIRECTION('ref_axis',(0.,0.,1.)) ;
#33944=DIRECTION('',(0.,0.,1.)) ;
#33945=DIRECTION('center_axis',(0.,1.,0.)) ;
#33946=DIRECTION('ref_axis',(0.,0.,1.)) ;
#33947=DIRECTION('',(0.,0.,-1.)) ;
#33948=DIRECTION('',(0.,0.,1.)) ;
#33949=DIRECTION('center_axis',(0.,-1.,0.)) ;
#33950=DIRECTION('ref_axis',(0.,0.,-1.)) ;
#33951=DIRECTION('',(0.,0.,-1.)) ;
#33952=DIRECTION('center_axis',(0.,-1.,0.)) ;
#33953=DIRECTION('ref_axis',(0.,0.,-1.)) ;
#33954=DIRECTION('',(0.,0.,1.)) ;
#33955=DIRECTION('',(0.,0.,-1.)) ;
#33956=DIRECTION('center_axis',(0.,-1.,0.)) ;
#33957=DIRECTION('ref_axis',(0.,0.,-1.)) ;
#33958=DIRECTION('',(0.,0.,-1.)) ;
#33959=DIRECTION('center_axis',(0.,-1.,0.)) ;
#33960=DIRECTION('ref_axis',(0.,0.,-1.)) ;
#33961=DIRECTION('',(0.,0.,-1.)) ;
#33962=DIRECTION('center_axis',(0.,-1.,0.)) ;
#33963=DIRECTION('ref_axis',(0.,0.,-1.)) ;
#33964=DIRECTION('',(0.,0.,-1.)) ;
#33965=DIRECTION('center_axis',(0.,-1.,0.)) ;
#33966=DIRECTION('ref_axis',(0.,0.,-1.)) ;
#33967=DIRECTION('center_axis',(1.,0.,0.)) ;
#33968=DIRECTION('ref_axis',(0.,0.,-1.)) ;
#33969=DIRECTION('',(0.,0.,-1.)) ;
#33970=DIRECTION('center_axis',(-1.,0.,0.)) ;
#33971=DIRECTION('ref_axis',(0.,0.,1.)) ;
#33972=DIRECTION('center_axis',(1.,0.,0.)) ;
#33973=DIRECTION('ref_axis',(0.,0.,-1.)) ;
#33974=DIRECTION('',(0.,0.,1.)) ;
#33975=DIRECTION('center_axis',(1.,0.,0.)) ;
#33976=DIRECTION('ref_axis',(0.,0.,-1.)) ;
#33977=DIRECTION('',(0.,0.,-1.)) ;
#33978=DIRECTION('center_axis',(0.,0.,1.)) ;
#33979=DIRECTION('ref_axis',(1.,0.,0.)) ;
#33980=DIRECTION('center_axis',(0.,0.,1.)) ;
#33981=DIRECTION('ref_axis',(1.,0.,0.)) ;
#33982=DIRECTION('',(0.,0.,1.)) ;
#33983=DIRECTION('center_axis',(0.,0.,1.)) ;
#33984=DIRECTION('ref_axis',(1.,0.,0.)) ;
#33985=DIRECTION('',(0.,0.,-1.)) ;
#33986=DIRECTION('center_axis',(-1.,0.,0.)) ;
#33987=DIRECTION('ref_axis',(0.,0.,1.)) ;
#33988=DIRECTION('center_axis',(1.,0.,0.)) ;
#33989=DIRECTION('ref_axis',(0.,0.,-1.)) ;
#33990=DIRECTION('',(0.,0.,1.)) ;
#33991=DIRECTION('center_axis',(-1.,0.,0.)) ;
#33992=DIRECTION('ref_axis',(0.,0.,1.)) ;
#33993=DIRECTION('center_axis',(1.,0.,0.)) ;
#33994=DIRECTION('ref_axis',(0.,0.,-1.)) ;
#33995=DIRECTION('',(0.,0.,1.)) ;
#33996=DIRECTION('center_axis',(-1.,0.,0.)) ;
#33997=DIRECTION('ref_axis',(0.,0.,1.)) ;
#33998=DIRECTION('center_axis',(1.,0.,0.)) ;
#33999=DIRECTION('ref_axis',(0.,0.,-1.)) ;
#34000=DIRECTION('',(0.,0.,1.)) ;
#34001=DIRECTION('center_axis',(0.,0.,1.)) ;
#34002=DIRECTION('ref_axis',(1.,0.,0.)) ;
#34003=DIRECTION('',(0.,0.,1.)) ;
#34004=DIRECTION('center_axis',(0.,0.,1.)) ;
#34005=DIRECTION('ref_axis',(1.,0.,0.)) ;
#34006=DIRECTION('',(0.,0.,1.)) ;
#34007=DIRECTION('center_axis',(-1.,0.,0.)) ;
#34008=DIRECTION('ref_axis',(0.,0.,1.)) ;
#34009=DIRECTION('',(0.,0.,-1.)) ;
#34010=DIRECTION('center_axis',(-1.,0.,0.)) ;
#34011=DIRECTION('ref_axis',(0.,0.,1.)) ;
#34012=DIRECTION('',(0.,0.,-1.)) ;
#34013=DIRECTION('center_axis',(-1.,0.,0.)) ;
#34014=DIRECTION('ref_axis',(0.,0.,1.)) ;
#34015=DIRECTION('',(0.,0.,-1.)) ;
#34016=DIRECTION('center_axis',(-1.,0.,0.)) ;
#34017=DIRECTION('ref_axis',(0.,0.,1.)) ;
#34018=DIRECTION('',(0.,0.,-1.)) ;
#34019=DIRECTION('',(0.,0.,-1.)) ;
#34020=DIRECTION('center_axis',(-1.,0.,0.)) ;
#34021=DIRECTION('ref_axis',(0.,0.,1.)) ;
#34022=DIRECTION('',(0.,0.,-1.)) ;
#34023=DIRECTION('center_axis',(-1.,0.,0.)) ;
#34024=DIRECTION('ref_axis',(0.,0.,1.)) ;
#34025=DIRECTION('center_axis',(-1.,0.,0.)) ;
#34026=DIRECTION('ref_axis',(0.,0.,1.)) ;
#34027=DIRECTION('',(0.,0.,-1.)) ;
#34028=DIRECTION('center_axis',(1.,0.,0.)) ;
#34029=DIRECTION('ref_axis',(0.,0.,-1.)) ;
#34030=DIRECTION('',(0.,0.,1.)) ;
#34031=DIRECTION('',(0.,0.,-1.)) ;
#34032=DIRECTION('center_axis',(1.,0.,0.)) ;
#34033=DIRECTION('ref_axis',(0.,0.,-1.)) ;
#34034=DIRECTION('',(0.,0.,1.)) ;
#34035=DIRECTION('',(0.,0.,-1.)) ;
#34036=DIRECTION('center_axis',(1.,0.,0.)) ;
#34037=DIRECTION('ref_axis',(0.,0.,-1.)) ;
#34038=DIRECTION('',(0.,0.,1.)) ;
#34039=DIRECTION('',(0.,0.,-1.)) ;
#34040=DIRECTION('center_axis',(1.,0.,0.)) ;
#34041=DIRECTION('ref_axis',(0.,0.,-1.)) ;
#34042=DIRECTION('',(0.,0.,-1.)) ;
#34043=DIRECTION('',(0.,0.,1.)) ;
#34044=DIRECTION('center_axis',(1.,0.,0.)) ;
#34045=DIRECTION('ref_axis',(0.,0.,-1.)) ;
#34046=DIRECTION('',(0.,0.,1.)) ;
#34047=DIRECTION('',(0.,0.,-1.)) ;
#34048=DIRECTION('center_axis',(1.,0.,0.)) ;
#34049=DIRECTION('ref_axis',(0.,0.,-1.)) ;
#34050=DIRECTION('',(0.,0.,-1.)) ;
#34051=DIRECTION('',(0.,0.,-1.)) ;
#34052=DIRECTION('center_axis',(0.,1.,0.)) ;
#34053=DIRECTION('ref_axis',(0.,0.,1.)) ;
#34054=DIRECTION('center_axis',(0.,-1.,0.)) ;
#34055=DIRECTION('ref_axis',(0.,0.,-1.)) ;
#34056=DIRECTION('center_axis',(0.,-1.,0.)) ;
#34057=DIRECTION('ref_axis',(0.,0.,-1.)) ;
#34058=DIRECTION('',(0.,0.,-1.)) ;
#34059=DIRECTION('center_axis',(0.,1.,0.)) ;
#34060=DIRECTION('ref_axis',(0.,0.,1.)) ;
#34061=DIRECTION('',(0.,0.,1.)) ;
#34062=DIRECTION('center_axis',(0.,1.,0.)) ;
#34063=DIRECTION('ref_axis',(0.,0.,1.)) ;
#34064=DIRECTION('center_axis',(0.,0.,1.)) ;
#34065=DIRECTION('ref_axis',(1.,0.,0.)) ;
#34066=DIRECTION('center_axis',(0.,0.,1.)) ;
#34067=DIRECTION('ref_axis',(1.,0.,0.)) ;
#34068=DIRECTION('',(0.,0.,1.)) ;
#34069=DIRECTION('center_axis',(0.,1.,0.)) ;
#34070=DIRECTION('ref_axis',(0.,0.,1.)) ;
#34071=DIRECTION('center_axis',(0.,-1.,0.)) ;
#34072=DIRECTION('ref_axis',(0.,0.,-1.)) ;
#34073=DIRECTION('',(0.,0.,1.)) ;
#34074=DIRECTION('center_axis',(0.,0.,1.)) ;
#34075=DIRECTION('ref_axis',(1.,0.,0.)) ;
#34076=DIRECTION('center_axis',(0.,0.,1.)) ;
#34077=DIRECTION('ref_axis',(1.,0.,0.)) ;
#34078=DIRECTION('',(0.,0.,-1.)) ;
#34079=DIRECTION('center_axis',(0.,0.,1.)) ;
#34080=DIRECTION('ref_axis',(1.,0.,0.)) ;
#34081=DIRECTION('',(0.,0.,1.)) ;
#34082=DIRECTION('center_axis',(0.,1.,0.)) ;
#34083=DIRECTION('ref_axis',(0.,0.,1.)) ;
#34084=DIRECTION('center_axis',(0.,-1.,0.)) ;
#34085=DIRECTION('ref_axis',(0.,0.,-1.)) ;
#34086=DIRECTION('',(0.,0.,1.)) ;
#34087=DIRECTION('center_axis',(0.,1.,0.)) ;
#34088=DIRECTION('ref_axis',(0.,0.,1.)) ;
#34089=DIRECTION('center_axis',(0.,-1.,0.)) ;
#34090=DIRECTION('ref_axis',(0.,0.,-1.)) ;
#34091=DIRECTION('',(0.,0.,1.)) ;
#34092=DIRECTION('center_axis',(0.,-1.,0.)) ;
#34093=DIRECTION('ref_axis',(0.,0.,-1.)) ;
#34094=DIRECTION('',(0.,0.,-1.)) ;
#34095=DIRECTION('center_axis',(0.,-1.,0.)) ;
#34096=DIRECTION('ref_axis',(0.,0.,-1.)) ;
#34097=DIRECTION('',(0.,0.,-1.)) ;
#34098=DIRECTION('center_axis',(0.,-1.,0.)) ;
#34099=DIRECTION('ref_axis',(0.,0.,-1.)) ;
#34100=DIRECTION('',(0.,0.,-1.)) ;
#34101=DIRECTION('center_axis',(0.,-1.,0.)) ;
#34102=DIRECTION('ref_axis',(0.,0.,-1.)) ;
#34103=DIRECTION('',(0.,0.,-1.)) ;
#34104=DIRECTION('center_axis',(0.,-1.,0.)) ;
#34105=DIRECTION('ref_axis',(0.,0.,-1.)) ;
#34106=DIRECTION('',(0.,0.,-1.)) ;
#34107=DIRECTION('center_axis',(0.,-1.,0.)) ;
#34108=DIRECTION('ref_axis',(0.,0.,-1.)) ;
#34109=DIRECTION('center_axis',(0.,1.,0.)) ;
#34110=DIRECTION('ref_axis',(0.,0.,1.)) ;
#34111=DIRECTION('',(0.,0.,1.)) ;
#34112=DIRECTION('',(0.,0.,-1.)) ;
#34113=DIRECTION('center_axis',(0.,1.,0.)) ;
#34114=DIRECTION('ref_axis',(0.,0.,1.)) ;
#34115=DIRECTION('',(0.,0.,-1.)) ;
#34116=DIRECTION('',(0.,0.,-1.)) ;
#34117=DIRECTION('center_axis',(0.,1.,0.)) ;
#34118=DIRECTION('ref_axis',(0.,0.,1.)) ;
#34119=DIRECTION('',(0.,0.,-1.)) ;
#34120=DIRECTION('',(0.,0.,1.)) ;
#34121=DIRECTION('center_axis',(0.,1.,0.)) ;
#34122=DIRECTION('ref_axis',(0.,0.,1.)) ;
#34123=DIRECTION('',(0.,0.,-1.)) ;
#34124=DIRECTION('',(0.,0.,1.)) ;
#34125=DIRECTION('center_axis',(0.,1.,0.)) ;
#34126=DIRECTION('ref_axis',(0.,0.,1.)) ;
#34127=DIRECTION('',(0.,0.,-1.)) ;
#34128=DIRECTION('',(0.,0.,1.)) ;
#34129=DIRECTION('center_axis',(1.,0.,0.)) ;
#34130=DIRECTION('ref_axis',(0.,0.,-1.)) ;
#34131=DIRECTION('center_axis',(-1.,0.,0.)) ;
#34132=DIRECTION('ref_axis',(0.,0.,1.)) ;
#34133=DIRECTION('center_axis',(1.,0.,0.)) ;
#34134=DIRECTION('ref_axis',(0.,0.,-1.)) ;
#34135=DIRECTION('',(0.,0.,-1.)) ;
#34136=DIRECTION('center_axis',(-1.,0.,0.)) ;
#34137=DIRECTION('ref_axis',(0.,0.,1.)) ;
#34138=DIRECTION('center_axis',(-1.,0.,0.)) ;
#34139=DIRECTION('ref_axis',(0.,0.,1.)) ;
#34140=DIRECTION('center_axis',(-1.,0.,0.)) ;
#34141=DIRECTION('ref_axis',(0.,0.,1.)) ;
#34142=DIRECTION('center_axis',(1.,0.,0.)) ;
#34143=DIRECTION('ref_axis',(0.,0.,-1.)) ;
#34144=DIRECTION('',(0.,0.,1.)) ;
#34145=DIRECTION('center_axis',(0.,0.,1.)) ;
#34146=DIRECTION('ref_axis',(1.,0.,0.)) ;
#34147=DIRECTION('',(0.,0.,1.)) ;
#34148=DIRECTION('center_axis',(-1.,0.,0.)) ;
#34149=DIRECTION('ref_axis',(0.,0.,1.)) ;
#34150=DIRECTION('center_axis',(1.,0.,0.)) ;
#34151=DIRECTION('ref_axis',(0.,0.,-1.)) ;
#34152=DIRECTION('',(0.,0.,1.)) ;
#34153=DIRECTION('center_axis',(0.,0.,1.)) ;
#34154=DIRECTION('ref_axis',(1.,0.,0.)) ;
#34155=DIRECTION('',(0.,0.,-1.)) ;
#34156=DIRECTION('center_axis',(0.,0.,1.)) ;
#34157=DIRECTION('ref_axis',(1.,0.,0.)) ;
#34158=DIRECTION('center_axis',(0.,0.,1.)) ;
#34159=DIRECTION('ref_axis',(1.,0.,0.)) ;
#34160=DIRECTION('',(0.,0.,1.)) ;
#34161=DIRECTION('center_axis',(0.,-1.,0.)) ;
#34162=DIRECTION('ref_axis',(0.,0.,-1.)) ;
#34163=DIRECTION('',(0.,0.,-1.)) ;
#34164=DIRECTION('center_axis',(1.,0.,0.)) ;
#34165=DIRECTION('ref_axis',(0.,0.,-1.)) ;
#34166=DIRECTION('',(0.,0.,1.)) ;
#34167=DIRECTION('',(0.,0.,-1.)) ;
#34168=DIRECTION('center_axis',(1.,0.,0.)) ;
#34169=DIRECTION('ref_axis',(0.,0.,-1.)) ;
#34170=DIRECTION('',(0.,0.,1.)) ;
#34171=DIRECTION('',(0.,0.,-1.)) ;
#34172=DIRECTION('center_axis',(1.,0.,0.)) ;
#34173=DIRECTION('ref_axis',(0.,0.,-1.)) ;
#34174=DIRECTION('',(0.,0.,1.)) ;
#34175=DIRECTION('',(0.,0.,-1.)) ;
#34176=DIRECTION('center_axis',(1.,0.,0.)) ;
#34177=DIRECTION('ref_axis',(0.,0.,-1.)) ;
#34178=DIRECTION('',(0.,0.,-1.)) ;
#34179=DIRECTION('center_axis',(1.,0.,0.)) ;
#34180=DIRECTION('ref_axis',(0.,0.,-1.)) ;
#34181=DIRECTION('',(0.,0.,1.)) ;
#34182=DIRECTION('',(0.,0.,-1.)) ;
#34183=DIRECTION('center_axis',(1.,0.,0.)) ;
#34184=DIRECTION('ref_axis',(0.,0.,-1.)) ;
#34185=DIRECTION('center_axis',(-1.,0.,0.)) ;
#34186=DIRECTION('ref_axis',(0.,0.,1.)) ;
#34187=DIRECTION('',(0.,0.,-1.)) ;
#34188=DIRECTION('center_axis',(-1.,0.,0.)) ;
#34189=DIRECTION('ref_axis',(0.,0.,1.)) ;
#34190=DIRECTION('',(0.,0.,-1.)) ;
#34191=DIRECTION('center_axis',(0.,1.,0.)) ;
#34192=DIRECTION('ref_axis',(0.,0.,1.)) ;
#34193=DIRECTION('center_axis',(-1.,0.,0.)) ;
#34194=DIRECTION('ref_axis',(0.,0.,1.)) ;
#34195=DIRECTION('',(0.,0.,-1.)) ;
#34196=DIRECTION('center_axis',(0.,1.,0.)) ;
#34197=DIRECTION('ref_axis',(0.,0.,1.)) ;
#34198=DIRECTION('center_axis',(0.,-1.,0.)) ;
#34199=DIRECTION('ref_axis',(0.,0.,-1.)) ;
#34200=DIRECTION('center_axis',(0.,-1.,0.)) ;
#34201=DIRECTION('ref_axis',(0.,0.,-1.)) ;
#34202=DIRECTION('',(0.,0.,-1.)) ;
#34203=DIRECTION('center_axis',(0.,1.,0.)) ;
#34204=DIRECTION('ref_axis',(0.,0.,1.)) ;
#34205=DIRECTION('center_axis',(0.,-1.,0.)) ;
#34206=DIRECTION('ref_axis',(0.,0.,-1.)) ;
#34207=DIRECTION('',(0.,0.,1.)) ;
#34208=DIRECTION('center_axis',(0.,0.,1.)) ;
#34209=DIRECTION('ref_axis',(1.,0.,0.)) ;
#34210=DIRECTION('',(0.,0.,1.)) ;
#34211=DIRECTION('center_axis',(0.,-1.,0.)) ;
#34212=DIRECTION('ref_axis',(0.,0.,-1.)) ;
#34213=DIRECTION('',(0.,0.,1.)) ;
#34214=DIRECTION('center_axis',(0.,1.,0.)) ;
#34215=DIRECTION('ref_axis',(0.,0.,1.)) ;
#34216=DIRECTION('center_axis',(0.,0.,1.)) ;
#34217=DIRECTION('ref_axis',(1.,0.,0.)) ;
#34218=DIRECTION('',(0.,0.,-1.)) ;
#34219=DIRECTION('center_axis',(0.,0.,1.)) ;
#34220=DIRECTION('ref_axis',(1.,0.,0.)) ;
#34221=DIRECTION('',(0.,0.,1.)) ;
#34222=DIRECTION('center_axis',(1.,0.,0.)) ;
#34223=DIRECTION('ref_axis',(0.,0.,-1.)) ;
#34224=DIRECTION('',(0.,0.,-1.)) ;
#34225=DIRECTION('center_axis',(0.,-1.,0.)) ;
#34226=DIRECTION('ref_axis',(0.,0.,-1.)) ;
#34227=DIRECTION('center_axis',(0.,-1.,0.)) ;
#34228=DIRECTION('ref_axis',(0.,0.,-1.)) ;
#34229=DIRECTION('',(0.,0.,-1.)) ;
#34230=DIRECTION('center_axis',(0.,1.,0.)) ;
#34231=DIRECTION('ref_axis',(0.,0.,1.)) ;
#34232=DIRECTION('',(0.,0.,-1.)) ;
#34233=DIRECTION('center_axis',(0.,1.,0.)) ;
#34234=DIRECTION('ref_axis',(0.,0.,1.)) ;
#34235=DIRECTION('',(0.,0.,-1.)) ;
#34236=DIRECTION('',(0.,0.,1.)) ;
#34237=DIRECTION('center_axis',(0.,1.,0.)) ;
#34238=DIRECTION('ref_axis',(0.,0.,1.)) ;
#34239=DIRECTION('',(0.,0.,1.)) ;
#34240=DIRECTION('',(0.,0.,-1.)) ;
#34241=DIRECTION('center_axis',(0.,1.,0.)) ;
#34242=DIRECTION('ref_axis',(0.,0.,1.)) ;
#34243=DIRECTION('',(0.,0.,-1.)) ;
#34244=DIRECTION('',(0.,0.,1.)) ;
#34245=DIRECTION('center_axis',(0.,1.,0.)) ;
#34246=DIRECTION('ref_axis',(0.,0.,1.)) ;
#34247=DIRECTION('',(0.,0.,1.)) ;
#34248=DIRECTION('center_axis',(-1.,0.,0.)) ;
#34249=DIRECTION('ref_axis',(0.,0.,1.)) ;
#34250=DIRECTION('',(0.,0.,-1.)) ;
#34251=DIRECTION('center_axis',(-1.,0.,0.)) ;
#34252=DIRECTION('ref_axis',(0.,0.,1.)) ;
#34253=DIRECTION('center_axis',(1.,0.,0.)) ;
#34254=DIRECTION('ref_axis',(0.,0.,-1.)) ;
#34255=DIRECTION('',(0.,0.,-1.)) ;
#34256=DIRECTION('center_axis',(0.,0.,1.)) ;
#34257=DIRECTION('ref_axis',(1.,0.,0.)) ;
#34258=DIRECTION('center_axis',(0.,0.,1.)) ;
#34259=DIRECTION('ref_axis',(1.,0.,0.)) ;
#34260=DIRECTION('',(0.,0.,-1.)) ;
#34261=DIRECTION('center_axis',(0.,0.,1.)) ;
#34262=DIRECTION('ref_axis',(1.,0.,0.)) ;
#34263=DIRECTION('center_axis',(-1.,0.,0.)) ;
#34264=DIRECTION('ref_axis',(0.,0.,1.)) ;
#34265=DIRECTION('center_axis',(1.,0.,0.)) ;
#34266=DIRECTION('ref_axis',(0.,0.,-1.)) ;
#34267=DIRECTION('',(0.,0.,-1.)) ;
#34268=DIRECTION('center_axis',(0.,0.,1.)) ;
#34269=DIRECTION('ref_axis',(1.,0.,0.)) ;
#34270=DIRECTION('',(0.,0.,1.)) ;
#34271=DIRECTION('center_axis',(0.,0.,1.)) ;
#34272=DIRECTION('ref_axis',(1.,0.,0.)) ;
#34273=DIRECTION('center_axis',(0.,-1.,0.)) ;
#34274=DIRECTION('ref_axis',(0.,0.,-1.)) ;
#34275=DIRECTION('',(0.,0.,-1.)) ;
#34276=DIRECTION('center_axis',(-1.,0.,0.)) ;
#34277=DIRECTION('ref_axis',(0.,0.,1.)) ;
#34278=DIRECTION('center_axis',(1.,0.,0.)) ;
#34279=DIRECTION('ref_axis',(0.,0.,-1.)) ;
#34280=DIRECTION('',(0.,0.,1.)) ;
#34281=DIRECTION('',(0.,0.,-1.)) ;
#34282=DIRECTION('center_axis',(1.,0.,0.)) ;
#34283=DIRECTION('ref_axis',(0.,0.,-1.)) ;
#34284=DIRECTION('center_axis',(1.,0.,0.)) ;
#34285=DIRECTION('ref_axis',(0.,0.,-1.)) ;
#34286=DIRECTION('',(0.,0.,1.)) ;
#34287=DIRECTION('',(0.,0.,-1.)) ;
#34288=DIRECTION('center_axis',(0.,1.,0.)) ;
#34289=DIRECTION('ref_axis',(0.,0.,1.)) ;
#34290=DIRECTION('center_axis',(-1.,0.,0.)) ;
#34291=DIRECTION('ref_axis',(0.,0.,1.)) ;
#34292=DIRECTION('',(0.,0.,-1.)) ;
#34293=DIRECTION('center_axis',(0.,1.,0.)) ;
#34294=DIRECTION('ref_axis',(0.,0.,1.)) ;
#34295=DIRECTION('center_axis',(0.,-1.,0.)) ;
#34296=DIRECTION('ref_axis',(0.,0.,-1.)) ;
#34297=DIRECTION('',(0.,0.,-1.)) ;
#34298=DIRECTION('center_axis',(0.,0.,1.)) ;
#34299=DIRECTION('ref_axis',(1.,0.,0.)) ;
#34300=DIRECTION('center_axis',(0.,-1.,0.)) ;
#34301=DIRECTION('ref_axis',(0.,0.,-1.)) ;
#34302=DIRECTION('',(0.,0.,-1.)) ;
#34303=DIRECTION('center_axis',(0.,0.,1.)) ;
#34304=DIRECTION('ref_axis',(1.,0.,0.)) ;
#34305=DIRECTION('',(0.,0.,-1.)) ;
#34306=DIRECTION('center_axis',(1.,0.,0.)) ;
#34307=DIRECTION('ref_axis',(0.,0.,-1.)) ;
#34308=DIRECTION('',(0.,0.,-1.)) ;
#34309=DIRECTION('center_axis',(0.,1.,0.)) ;
#34310=DIRECTION('ref_axis',(0.,0.,1.)) ;
#34311=DIRECTION('',(0.,0.,-1.)) ;
#34312=DIRECTION('center_axis',(0.,1.,0.)) ;
#34313=DIRECTION('ref_axis',(0.,0.,1.)) ;
#34314=DIRECTION('',(0.,0.,-1.)) ;
#34315=DIRECTION('center_axis',(0.,1.,0.)) ;
#34316=DIRECTION('ref_axis',(0.,0.,1.)) ;
#34317=DIRECTION('',(0.,0.,1.)) ;
#34318=DIRECTION('center_axis',(-1.,0.,0.)) ;
#34319=DIRECTION('ref_axis',(0.,0.,1.)) ;
#34320=DIRECTION('center_axis',(-1.,0.,0.)) ;
#34321=DIRECTION('ref_axis',(0.,0.,1.)) ;
#34322=DIRECTION('',(0.,0.,1.)) ;
#34323=DIRECTION('center_axis',(-1.,0.,0.)) ;
#34324=DIRECTION('ref_axis',(0.,0.,1.)) ;
#34325=DIRECTION('center_axis',(0.,0.,1.)) ;
#34326=DIRECTION('ref_axis',(1.,0.,0.)) ;
#34327=DIRECTION('',(0.,0.,1.)) ;
#34328=DIRECTION('center_axis',(0.,-1.,0.)) ;
#34329=DIRECTION('ref_axis',(0.,0.,-1.)) ;
#34330=DIRECTION('',(0.,0.,-1.)) ;
#34331=DIRECTION('center_axis',(1.,0.,0.)) ;
#34332=DIRECTION('ref_axis',(0.,0.,-1.)) ;
#34333=DIRECTION('center_axis',(1.,0.,0.)) ;
#34334=DIRECTION('ref_axis',(0.,0.,-1.)) ;
#34335=DIRECTION('center_axis',(1.,0.,0.)) ;
#34336=DIRECTION('ref_axis',(0.,0.,-1.)) ;
#34337=DIRECTION('',(0.,0.,-1.)) ;
#34338=DIRECTION('center_axis',(0.,1.,0.)) ;
#34339=DIRECTION('ref_axis',(0.,0.,1.)) ;
#34340=DIRECTION('',(0.,0.,-1.)) ;
#34341=DIRECTION('center_axis',(0.,0.,1.)) ;
#34342=DIRECTION('ref_axis',(1.,0.,0.)) ;
#34343=DIRECTION('',(0.,0.,1.)) ;
#34344=DIRECTION('center_axis',(0.,0.,1.)) ;
#34345=DIRECTION('ref_axis',(1.,0.,0.)) ;
#34346=DIRECTION('center_axis',(0.,-1.,0.)) ;
#34347=DIRECTION('ref_axis',(0.,0.,-1.)) ;
#34348=DIRECTION('center_axis',(1.,0.,0.)) ;
#34349=DIRECTION('ref_axis',(0.,0.,-1.)) ;
#34350=DIRECTION('',(0.,0.,-1.)) ;
#34351=DIRECTION('center_axis',(0.,1.,0.)) ;
#34352=DIRECTION('ref_axis',(0.,0.,1.)) ;
#34353=DIRECTION('',(0.,0.,-1.)) ;
#34354=DIRECTION('center_axis',(0.,1.,0.)) ;
#34355=DIRECTION('ref_axis',(0.,0.,1.)) ;
#34356=DIRECTION('center_axis',(0.,1.,0.)) ;
#34357=DIRECTION('ref_axis',(0.,0.,1.)) ;
#34358=DIRECTION('center_axis',(-1.,0.,0.)) ;
#34359=DIRECTION('ref_axis',(0.,0.,1.)) ;
#41686=CARTESIAN_POINT('',(0.,0.,0.)) ;
#41687=CARTESIAN_POINT('Origin',(41.6,0.,108.3)) ;
#41688=CARTESIAN_POINT('',(41.6,-28.4,108.)) ;
#41689=CARTESIAN_POINT('',(41.6,-28.4,108.6)) ;
#41690=CARTESIAN_POINT('',(41.6,-28.4,108.3)) ;
#41691=CARTESIAN_POINT('',(41.6,-28.6302287800849,108.)) ;
#41692=CARTESIAN_POINT('',(41.6,0.,108.)) ;
#41693=CARTESIAN_POINT('',(41.6,-28.6302287800849,108.6)) ;
#41694=CARTESIAN_POINT('',(41.6,-28.6302287800849,108.3)) ;
#41695=CARTESIAN_POINT('',(41.6,0.,108.6)) ;
#41696=CARTESIAN_POINT('Origin',(41.6,0.,108.3)) ;
#41697=CARTESIAN_POINT('',(41.6,-14.4,108.)) ;
#41698=CARTESIAN_POINT('',(41.6,-14.4,108.6)) ;
#41699=CARTESIAN_POINT('',(41.6,-14.4,108.3)) ;
#41700=CARTESIAN_POINT('',(41.6,-27.6,108.)) ;
#41701=CARTESIAN_POINT('',(41.6,0.,108.)) ;
#41702=CARTESIAN_POINT('',(41.6,-27.6,108.6)) ;
#41703=CARTESIAN_POINT('',(41.6,-27.6,108.3)) ;
#41704=CARTESIAN_POINT('',(41.6,0.,108.6)) ;
#41705=CARTESIAN_POINT('Origin',(41.6,0.,108.3)) ;
#41706=CARTESIAN_POINT('',(41.6,-0.4,108.)) ;
#41707=CARTESIAN_POINT('',(41.6,-0.4,108.6)) ;
#41708=CARTESIAN_POINT('',(41.6,-0.4,108.3)) ;
#41709=CARTESIAN_POINT('',(41.6,-13.6,108.)) ;
#41710=CARTESIAN_POINT('',(41.6,0.,108.)) ;
#41711=CARTESIAN_POINT('',(41.6,-13.6,108.6)) ;
#41712=CARTESIAN_POINT('',(41.6,-13.6,108.3)) ;
#41713=CARTESIAN_POINT('',(41.6,0.,108.6)) ;
#41714=CARTESIAN_POINT('Origin',(41.6,0.,108.3)) ;
#41715=CARTESIAN_POINT('',(41.6,13.6,108.)) ;
#41716=CARTESIAN_POINT('',(41.6,13.6,108.6)) ;
#41717=CARTESIAN_POINT('',(41.6,13.6,108.3)) ;
#41718=CARTESIAN_POINT('',(41.6,0.4,108.)) ;
#41719=CARTESIAN_POINT('',(41.6,0.,108.)) ;
#41720=CARTESIAN_POINT('',(41.6,0.4,108.6)) ;
#41721=CARTESIAN_POINT('',(41.6,0.4,108.3)) ;
#41722=CARTESIAN_POINT('',(41.6,0.,108.6)) ;
#41723=CARTESIAN_POINT('Origin',(41.6,0.,108.3)) ;
#41724=CARTESIAN_POINT('',(41.6,27.6,108.)) ;
#41725=CARTESIAN_POINT('',(41.6,27.6,108.6)) ;
#41726=CARTESIAN_POINT('',(41.6,27.6,108.3)) ;
#41727=CARTESIAN_POINT('',(41.6,14.4,108.)) ;
#41728=CARTESIAN_POINT('',(41.6,0.,108.)) ;
#41729=CARTESIAN_POINT('',(41.6,14.4,108.6)) ;
#41730=CARTESIAN_POINT('',(41.6,14.4,108.3)) ;
#41731=CARTESIAN_POINT('',(41.6,0.,108.6)) ;
#41732=CARTESIAN_POINT('Origin',(41.6,0.,108.3)) ;
#41733=CARTESIAN_POINT('',(41.6,28.6302287800849,108.)) ;
#41734=CARTESIAN_POINT('',(41.6,28.6302287800849,108.6)) ;
#41735=CARTESIAN_POINT('',(41.6,28.6302287800849,108.3)) ;
#41736=CARTESIAN_POINT('',(41.6,28.4,108.)) ;
#41737=CARTESIAN_POINT('',(41.6,0.,108.)) ;
#41738=CARTESIAN_POINT('',(41.6,28.4,108.6)) ;
#41739=CARTESIAN_POINT('',(41.6,28.4,108.3)) ;
#41740=CARTESIAN_POINT('',(41.6,0.,108.6)) ;
#41741=CARTESIAN_POINT('Origin',(42.4,0.,108.3)) ;
#41742=CARTESIAN_POINT('',(42.4,29.2316609175736,108.)) ;
#41743=CARTESIAN_POINT('',(42.4,29.2316609175736,108.6)) ;
#41744=CARTESIAN_POINT('',(42.4,29.2316609175736,108.3)) ;
#41745=CARTESIAN_POINT('',(42.4,29.8035232816525,108.)) ;
#41746=CARTESIAN_POINT('',(42.4,0.,108.)) ;
#41747=CARTESIAN_POINT('',(42.4,29.8035232816525,108.6)) ;
#41748=CARTESIAN_POINT('',(42.4,29.8035232816525,108.3)) ;
#41749=CARTESIAN_POINT('',(42.4,0.,108.6)) ;
#41750=CARTESIAN_POINT('Origin',(42.4,0.,108.3)) ;
#41751=CARTESIAN_POINT('',(42.4,-29.2316609175736,108.6)) ;
#41752=CARTESIAN_POINT('',(42.4,-29.2316609175736,108.)) ;
#41753=CARTESIAN_POINT('',(42.4,-29.2316609175736,108.3)) ;
#41754=CARTESIAN_POINT('',(42.4,-29.8035232816525,108.6)) ;
#41755=CARTESIAN_POINT('',(42.4,0.,108.6)) ;
#41756=CARTESIAN_POINT('',(42.4,-29.8035232816525,108.)) ;
#41757=CARTESIAN_POINT('',(42.4,-29.8035232816525,108.3)) ;
#41758=CARTESIAN_POINT('',(42.4,0.,108.)) ;
#41759=CARTESIAN_POINT('Origin',(42.4,0.,108.3)) ;
#41760=CARTESIAN_POINT('',(42.4,-14.4,108.6)) ;
#41761=CARTESIAN_POINT('',(42.4,-14.4,108.)) ;
#41762=CARTESIAN_POINT('',(42.4,-14.4,108.3)) ;
#41763=CARTESIAN_POINT('',(42.4,-27.4315511774307,108.6)) ;
#41764=CARTESIAN_POINT('',(42.4,0.,108.6)) ;
#41765=CARTESIAN_POINT('',(42.4,-27.4315511774307,108.)) ;
#41766=CARTESIAN_POINT('',(42.4,-27.4315511774307,108.3)) ;
#41767=CARTESIAN_POINT('',(42.4,0.,108.)) ;
#41768=CARTESIAN_POINT('Origin',(42.4,0.,108.3)) ;
#41769=CARTESIAN_POINT('',(42.4,-0.4,108.6)) ;
#41770=CARTESIAN_POINT('',(42.4,-0.4,108.)) ;
#41771=CARTESIAN_POINT('',(42.4,-0.4,108.3)) ;
#41772=CARTESIAN_POINT('',(42.4,-13.6,108.6)) ;
#41773=CARTESIAN_POINT('',(42.4,0.,108.6)) ;
#41774=CARTESIAN_POINT('',(42.4,-13.6,108.)) ;
#41775=CARTESIAN_POINT('',(42.4,-13.6,108.3)) ;
#41776=CARTESIAN_POINT('',(42.4,0.,108.)) ;
#41777=CARTESIAN_POINT('Origin',(42.4,0.,108.3)) ;
#41778=CARTESIAN_POINT('',(42.4,13.6,108.6)) ;
#41779=CARTESIAN_POINT('',(42.4,13.6,108.)) ;
#41780=CARTESIAN_POINT('',(42.4,13.6,108.3)) ;
#41781=CARTESIAN_POINT('',(42.4,0.4,108.6)) ;
#41782=CARTESIAN_POINT('',(42.4,0.,108.6)) ;
#41783=CARTESIAN_POINT('',(42.4,0.4,108.)) ;
#41784=CARTESIAN_POINT('',(42.4,0.4,108.3)) ;
#41785=CARTESIAN_POINT('',(42.4,0.,108.)) ;
#41786=CARTESIAN_POINT('Origin',(42.4,0.,108.3)) ;
#41787=CARTESIAN_POINT('',(42.4,27.4315511774307,108.6)) ;
#41788=CARTESIAN_POINT('',(42.4,27.4315511774307,108.)) ;
#41789=CARTESIAN_POINT('',(42.4,27.4315511774307,108.3)) ;
#41790=CARTESIAN_POINT('',(42.4,14.4,108.6)) ;
#41791=CARTESIAN_POINT('',(42.4,0.,108.6)) ;
#41792=CARTESIAN_POINT('',(42.4,14.4,108.)) ;
#41793=CARTESIAN_POINT('',(42.4,14.4,108.3)) ;
#41794=CARTESIAN_POINT('',(42.4,0.,108.)) ;
#41795=CARTESIAN_POINT('Origin',(42.,-29.8035232816525,108.3)) ;
#41796=CARTESIAN_POINT('',(42.,-29.8035232816525,108.)) ;
#41797=CARTESIAN_POINT('',(42.,-29.8035232816525,108.6)) ;
#41798=CARTESIAN_POINT('',(42.,-29.8035232816525,108.3)) ;
#41799=CARTESIAN_POINT('',(42.,-29.8035232816525,108.)) ;
#41800=CARTESIAN_POINT('',(42.,-29.8035232816525,108.6)) ;
#41801=CARTESIAN_POINT('Origin',(42.,29.8035232816525,108.3)) ;
#41802=CARTESIAN_POINT('',(42.,29.8035232816525,108.6)) ;
#41803=CARTESIAN_POINT('',(42.,29.8035232816525,108.)) ;
#41804=CARTESIAN_POINT('',(42.,29.8035232816525,108.3)) ;
#41805=CARTESIAN_POINT('',(42.,29.8035232816525,108.6)) ;
#41806=CARTESIAN_POINT('',(42.,29.8035232816525,108.)) ;
#41807=CARTESIAN_POINT('Origin',(0.,0.,108.3)) ;
#41808=CARTESIAN_POINT('',(42.9614943874163,28.4,108.6)) ;
#41809=CARTESIAN_POINT('Origin',(0.,0.,108.6)) ;
#41810=CARTESIAN_POINT('',(42.9614943874163,28.4,108.)) ;
#41811=CARTESIAN_POINT('',(42.9614943874163,28.4,108.3)) ;
#41812=CARTESIAN_POINT('Origin',(0.,0.,108.)) ;
#41813=CARTESIAN_POINT('Origin',(0.,0.,108.3)) ;
#41814=CARTESIAN_POINT('',(29.8035232816525,42.,108.)) ;
#41815=CARTESIAN_POINT('Origin',(0.,0.,108.)) ;
#41816=CARTESIAN_POINT('',(29.8035232816525,42.,108.6)) ;
#41817=CARTESIAN_POINT('',(29.8035232816525,42.,108.3)) ;
#41818=CARTESIAN_POINT('Origin',(0.,0.,108.6)) ;
#41819=CARTESIAN_POINT('Origin',(0.,0.,108.3)) ;
#41820=CARTESIAN_POINT('',(48.4034089708566,14.4,108.)) ;
#41821=CARTESIAN_POINT('Origin',(0.,0.,108.)) ;
#41822=CARTESIAN_POINT('',(48.4034089708566,14.4,108.6)) ;
#41823=CARTESIAN_POINT('',(48.4034089708566,14.4,108.3)) ;
#41824=CARTESIAN_POINT('Origin',(0.,0.,108.6)) ;
#41825=CARTESIAN_POINT('Origin',(0.,28.4,108.3)) ;
#41826=CARTESIAN_POINT('',(28.4,28.4,108.)) ;
#41827=CARTESIAN_POINT('',(0.,28.4,108.)) ;
#41828=CARTESIAN_POINT('',(28.4,28.4,108.6)) ;
#41829=CARTESIAN_POINT('',(28.4,28.4,108.3)) ;
#41830=CARTESIAN_POINT('',(0.,28.4,108.6)) ;
#41831=CARTESIAN_POINT('Origin',(0.,13.6,108.3)) ;
#41832=CARTESIAN_POINT('',(48.6342471926933,13.6,108.)) ;
#41833=CARTESIAN_POINT('',(0.,13.6,108.)) ;
#41834=CARTESIAN_POINT('',(48.6342471926933,13.6,108.6)) ;
#41835=CARTESIAN_POINT('',(48.6342471926933,13.6,108.3)) ;
#41836=CARTESIAN_POINT('',(0.,13.6,108.6)) ;
#41837=CARTESIAN_POINT('Origin',(0.,14.4,108.3)) ;
#41838=CARTESIAN_POINT('',(28.4,14.4,108.)) ;
#41839=CARTESIAN_POINT('',(0.,14.4,108.)) ;
#41840=CARTESIAN_POINT('',(28.4,14.4,108.6)) ;
#41841=CARTESIAN_POINT('',(28.4,14.4,108.3)) ;
#41842=CARTESIAN_POINT('',(0.,14.4,108.6)) ;
#41843=CARTESIAN_POINT('Origin',(0.,-0.4,108.3)) ;
#41844=CARTESIAN_POINT('',(50.4984158167363,-0.4,108.)) ;
#41845=CARTESIAN_POINT('',(0.,-0.4,108.)) ;
#41846=CARTESIAN_POINT('',(50.4984158167363,-0.4,108.6)) ;
#41847=CARTESIAN_POINT('',(50.4984158167363,-0.4,108.3)) ;
#41848=CARTESIAN_POINT('',(0.,-0.4,108.6)) ;
#41849=CARTESIAN_POINT('Origin',(0.,0.4,108.3)) ;
#41850=CARTESIAN_POINT('',(28.4,0.4,108.)) ;
#41851=CARTESIAN_POINT('',(0.,0.4,108.)) ;
#41852=CARTESIAN_POINT('',(28.4,0.4,108.6)) ;
#41853=CARTESIAN_POINT('',(28.4,0.4,108.3)) ;
#41854=CARTESIAN_POINT('',(0.,0.4,108.6)) ;
#41855=CARTESIAN_POINT('Origin',(0.,-14.4,108.3)) ;
#41856=CARTESIAN_POINT('',(48.4034089708566,-14.4,108.)) ;
#41857=CARTESIAN_POINT('',(0.,-14.4,108.)) ;
#41858=CARTESIAN_POINT('',(48.4034089708566,-14.4,108.6)) ;
#41859=CARTESIAN_POINT('',(48.4034089708566,-14.4,108.3)) ;
#41860=CARTESIAN_POINT('',(0.,-14.4,108.6)) ;
#41861=CARTESIAN_POINT('Origin',(0.,-13.6,108.3)) ;
#41862=CARTESIAN_POINT('',(28.4,-13.6,108.)) ;
#41863=CARTESIAN_POINT('',(0.,-13.6,108.)) ;
#41864=CARTESIAN_POINT('',(28.4,-13.6,108.6)) ;
#41865=CARTESIAN_POINT('',(28.4,-13.6,108.3)) ;
#41866=CARTESIAN_POINT('',(0.,-13.6,108.6)) ;
#41867=CARTESIAN_POINT('Origin',(0.,-27.6,108.3)) ;
#41868=CARTESIAN_POINT('',(28.4,-27.6,108.)) ;
#41869=CARTESIAN_POINT('',(0.,-27.6,108.)) ;
#41870=CARTESIAN_POINT('',(28.4,-27.6,108.6)) ;
#41871=CARTESIAN_POINT('',(28.4,-27.6,108.3)) ;
#41872=CARTESIAN_POINT('',(0.,-27.6,108.6)) ;
#41873=CARTESIAN_POINT('Origin',(0.,0.,108.6)) ;
#41874=CARTESIAN_POINT('',(29.8035232816525,42.4,108.6)) ;
#41875=CARTESIAN_POINT('',(29.8035232816525,42.,108.6)) ;
#41876=CARTESIAN_POINT('',(29.2316609175736,42.4,108.6)) ;
#41877=CARTESIAN_POINT('',(0.,42.4,108.6)) ;
#41878=CARTESIAN_POINT('',(28.4,42.9614943874163,108.6)) ;
#41879=CARTESIAN_POINT('Origin',(0.,0.,108.6)) ;
#41880=CARTESIAN_POINT('',(28.4,43.2232576282723,108.6)) ;
#41881=CARTESIAN_POINT('',(28.4,0.,108.6)) ;
#41882=CARTESIAN_POINT('',(28.,43.2232576282723,108.6)) ;
#41883=CARTESIAN_POINT('',(28.,43.2232576282723,108.6)) ;
#41884=CARTESIAN_POINT('',(14.4,49.4458289444115,108.6)) ;
#41885=CARTESIAN_POINT('Origin',(0.,0.,108.6)) ;
#41886=CARTESIAN_POINT('',(14.4,49.5605690039975,108.6)) ;
#41887=CARTESIAN_POINT('',(14.4,0.,108.6)) ;
#41888=CARTESIAN_POINT('',(14.,49.5605690039975,108.6)) ;
#41889=CARTESIAN_POINT('',(14.,49.5605690039975,108.6)) ;
#41890=CARTESIAN_POINT('',(0.4,51.4984465785134,108.6)) ;
#41891=CARTESIAN_POINT('Origin',(0.,0.,108.6)) ;
#41892=CARTESIAN_POINT('',(0.4,51.5,108.6)) ;
#41893=CARTESIAN_POINT('',(0.4,0.,108.6)) ;
#41894=CARTESIAN_POINT('',(-0.4,51.5,108.6)) ;
#41895=CARTESIAN_POINT('',(0.,51.5,108.6)) ;
#41896=CARTESIAN_POINT('',(-0.4,51.4984465785134,108.6)) ;
#41897=CARTESIAN_POINT('',(-0.4,0.,108.6)) ;
#41898=CARTESIAN_POINT('',(-14.,49.5605690039975,108.6)) ;
#41899=CARTESIAN_POINT('Origin',(0.,0.,108.6)) ;
#41900=CARTESIAN_POINT('',(-14.4,49.5605690039975,108.6)) ;
#41901=CARTESIAN_POINT('',(-14.,49.5605690039975,108.6)) ;
#41902=CARTESIAN_POINT('',(-14.4,49.4458289444115,108.6)) ;
#41903=CARTESIAN_POINT('',(-14.4,0.,108.6)) ;
#41904=CARTESIAN_POINT('',(-28.,43.2232576282723,108.6)) ;
#41905=CARTESIAN_POINT('Origin',(0.,0.,108.6)) ;
#41906=CARTESIAN_POINT('',(-28.4,43.2232576282723,108.6)) ;
#41907=CARTESIAN_POINT('',(-28.,43.2232576282723,108.6)) ;
#41908=CARTESIAN_POINT('',(-28.4,42.9614943874163,108.6)) ;
#41909=CARTESIAN_POINT('',(-28.4,0.,108.6)) ;
#41910=CARTESIAN_POINT('',(-29.2316609175736,42.4,108.6)) ;
#41911=CARTESIAN_POINT('Origin',(0.,0.,108.6)) ;
#41912=CARTESIAN_POINT('',(-29.8035232816525,42.4,108.6)) ;
#41913=CARTESIAN_POINT('',(0.,42.4,108.6)) ;
#41914=CARTESIAN_POINT('',(-29.8035232816525,42.,108.6)) ;
#41915=CARTESIAN_POINT('',(-29.8035232816525,42.,108.6)) ;
#41916=CARTESIAN_POINT('',(-42.,29.8035232816525,108.6)) ;
#41917=CARTESIAN_POINT('Origin',(0.,0.,108.6)) ;
#41918=CARTESIAN_POINT('',(-42.4,29.8035232816525,108.6)) ;
#41919=CARTESIAN_POINT('',(-42.,29.8035232816525,108.6)) ;
#41920=CARTESIAN_POINT('',(-42.4,29.2316609175736,108.6)) ;
#41921=CARTESIAN_POINT('',(-42.4,0.,108.6)) ;
#41922=CARTESIAN_POINT('',(-42.9614943874163,28.4,108.6)) ;
#41923=CARTESIAN_POINT('Origin',(0.,0.,108.6)) ;
#41924=CARTESIAN_POINT('',(-43.2232576282723,28.4,108.6)) ;
#41925=CARTESIAN_POINT('',(0.,28.4,108.6)) ;
#41926=CARTESIAN_POINT('',(-43.2232576282723,28.,108.6)) ;
#41927=CARTESIAN_POINT('',(-43.2232576282723,28.,108.6)) ;
#41928=CARTESIAN_POINT('',(-49.4458289444115,14.4,108.6)) ;
#41929=CARTESIAN_POINT('Origin',(0.,0.,108.6)) ;
#41930=CARTESIAN_POINT('',(-49.5605690039975,14.4,108.6)) ;
#41931=CARTESIAN_POINT('',(0.,14.4,108.6)) ;
#41932=CARTESIAN_POINT('',(-49.5605690039975,14.,108.6)) ;
#41933=CARTESIAN_POINT('',(-49.5605690039975,14.,108.6)) ;
#41934=CARTESIAN_POINT('',(-51.4984465785134,0.4,108.6)) ;
#41935=CARTESIAN_POINT('Origin',(0.,0.,108.6)) ;
#41936=CARTESIAN_POINT('',(-51.5,0.4,108.6)) ;
#41937=CARTESIAN_POINT('',(0.,0.4,108.6)) ;
#41938=CARTESIAN_POINT('',(-51.5,-0.4,108.6)) ;
#41939=CARTESIAN_POINT('',(-51.5,0.,108.6)) ;
#41940=CARTESIAN_POINT('',(-51.4984465785134,-0.4,108.6)) ;
#41941=CARTESIAN_POINT('',(0.,-0.4,108.6)) ;
#41942=CARTESIAN_POINT('',(-49.5605690039975,-14.,108.6)) ;
#41943=CARTESIAN_POINT('Origin',(0.,0.,108.6)) ;
#41944=CARTESIAN_POINT('',(-49.5605690039975,-14.4,108.6)) ;
#41945=CARTESIAN_POINT('',(-49.5605690039975,-14.,108.6)) ;
#41946=CARTESIAN_POINT('',(-49.4458289444115,-14.4,108.6)) ;
#41947=CARTESIAN_POINT('',(0.,-14.4,108.6)) ;
#41948=CARTESIAN_POINT('',(-43.2232576282723,-28.,108.6)) ;
#41949=CARTESIAN_POINT('Origin',(0.,0.,108.6)) ;
#41950=CARTESIAN_POINT('',(-43.2232576282723,-28.4,108.6)) ;
#41951=CARTESIAN_POINT('',(-43.2232576282723,-28.,108.6)) ;
#41952=CARTESIAN_POINT('',(-42.9614943874163,-28.4,108.6)) ;
#41953=CARTESIAN_POINT('',(0.,-28.4,108.6)) ;
#41954=CARTESIAN_POINT('',(-42.4,-29.2316609175736,108.6)) ;
#41955=CARTESIAN_POINT('Origin',(0.,0.,108.6)) ;
#41956=CARTESIAN_POINT('',(-42.4,-29.8035232816525,108.6)) ;
#41957=CARTESIAN_POINT('',(-42.4,0.,108.6)) ;
#41958=CARTESIAN_POINT('',(-42.,-29.8035232816525,108.6)) ;
#41959=CARTESIAN_POINT('',(-42.,-29.8035232816525,108.6)) ;
#41960=CARTESIAN_POINT('',(-29.8035232816525,-42.,108.6)) ;
#41961=CARTESIAN_POINT('Origin',(0.,0.,108.6)) ;
#41962=CARTESIAN_POINT('',(-29.8035232816525,-42.4,108.6)) ;
#41963=CARTESIAN_POINT('',(-29.8035232816525,-42.,108.6)) ;
#41964=CARTESIAN_POINT('',(-29.2316609175736,-42.4,108.6)) ;
#41965=CARTESIAN_POINT('',(0.,-42.4,108.6)) ;
#41966=CARTESIAN_POINT('',(-28.4,-42.9614943874163,108.6)) ;
#41967=CARTESIAN_POINT('Origin',(0.,0.,108.6)) ;
#41968=CARTESIAN_POINT('',(-28.4,-43.2232576282723,108.6)) ;
#41969=CARTESIAN_POINT('',(-28.4,0.,108.6)) ;
#41970=CARTESIAN_POINT('',(-28.,-43.2232576282723,108.6)) ;
#41971=CARTESIAN_POINT('',(-28.,-43.2232576282723,108.6)) ;
#41972=CARTESIAN_POINT('',(-14.4,-49.4458289444115,108.6)) ;
#41973=CARTESIAN_POINT('Origin',(0.,0.,108.6)) ;
#41974=CARTESIAN_POINT('',(-14.4,-49.5605690039975,108.6)) ;
#41975=CARTESIAN_POINT('',(-14.4,0.,108.6)) ;
#41976=CARTESIAN_POINT('',(-14.,-49.5605690039975,108.6)) ;
#41977=CARTESIAN_POINT('',(-14.,-49.5605690039975,108.6)) ;
#41978=CARTESIAN_POINT('',(-0.4,-51.4984465785134,108.6)) ;
#41979=CARTESIAN_POINT('Origin',(0.,0.,108.6)) ;
#41980=CARTESIAN_POINT('',(-0.4,-51.5,108.6)) ;
#41981=CARTESIAN_POINT('',(-0.4,0.,108.6)) ;
#41982=CARTESIAN_POINT('',(0.4,-51.5,108.6)) ;
#41983=CARTESIAN_POINT('',(0.,-51.5,108.6)) ;
#41984=CARTESIAN_POINT('',(0.4,-51.4984465785134,108.6)) ;
#41985=CARTESIAN_POINT('',(0.4,0.,108.6)) ;
#41986=CARTESIAN_POINT('',(14.,-49.5605690039975,108.6)) ;
#41987=CARTESIAN_POINT('Origin',(0.,0.,108.6)) ;
#41988=CARTESIAN_POINT('',(14.4,-49.5605690039975,108.6)) ;
#41989=CARTESIAN_POINT('',(14.,-49.5605690039975,108.6)) ;
#41990=CARTESIAN_POINT('',(14.4,-49.4458289444115,108.6)) ;
#41991=CARTESIAN_POINT('',(14.4,0.,108.6)) ;
#41992=CARTESIAN_POINT('',(28.,-43.2232576282723,108.6)) ;
#41993=CARTESIAN_POINT('Origin',(0.,0.,108.6)) ;
#41994=CARTESIAN_POINT('',(28.4,-43.2232576282723,108.6)) ;
#41995=CARTESIAN_POINT('',(28.,-43.2232576282723,108.6)) ;
#41996=CARTESIAN_POINT('',(28.4,-42.9614943874163,108.6)) ;
#41997=CARTESIAN_POINT('',(28.4,0.,108.6)) ;
#41998=CARTESIAN_POINT('',(29.2316609175736,-42.4,108.6)) ;
#41999=CARTESIAN_POINT('Origin',(0.,0.,108.6)) ;
#42000=CARTESIAN_POINT('',(29.8035232816525,-42.4,108.6)) ;
#42001=CARTESIAN_POINT('',(0.,-42.4,108.6)) ;
#42002=CARTESIAN_POINT('',(29.8035232816525,-42.,108.6)) ;
#42003=CARTESIAN_POINT('',(29.8035232816525,-42.,108.6)) ;
#42004=CARTESIAN_POINT('Origin',(0.,0.,108.6)) ;
#42005=CARTESIAN_POINT('',(42.9614943874163,-28.4,108.6)) ;
#42006=CARTESIAN_POINT('Origin',(0.,0.,108.6)) ;
#42007=CARTESIAN_POINT('',(43.2232576282723,-28.4,108.6)) ;
#42008=CARTESIAN_POINT('',(0.,-28.4,108.6)) ;
#42009=CARTESIAN_POINT('',(43.2232576282723,-28.,108.6)) ;
#42010=CARTESIAN_POINT('',(43.2232576282723,-28.,108.6)) ;
#42011=CARTESIAN_POINT('',(49.4458289444115,-14.4,108.6)) ;
#42012=CARTESIAN_POINT('Origin',(0.,0.,108.6)) ;
#42013=CARTESIAN_POINT('',(49.5605690039975,-14.4,108.6)) ;
#42014=CARTESIAN_POINT('',(0.,-14.4,108.6)) ;
#42015=CARTESIAN_POINT('',(49.5605690039975,-14.,108.6)) ;
#42016=CARTESIAN_POINT('',(49.5605690039975,-14.,108.6)) ;
#42017=CARTESIAN_POINT('',(51.4984465785134,-0.4,108.6)) ;
#42018=CARTESIAN_POINT('Origin',(0.,0.,108.6)) ;
#42019=CARTESIAN_POINT('',(51.5,-0.4,108.6)) ;
#42020=CARTESIAN_POINT('',(0.,-0.4,108.6)) ;
#42021=CARTESIAN_POINT('',(51.5,0.4,108.6)) ;
#42022=CARTESIAN_POINT('',(51.5,0.,108.6)) ;
#42023=CARTESIAN_POINT('',(51.4984465785134,0.4,108.6)) ;
#42024=CARTESIAN_POINT('',(0.,0.4,108.6)) ;
#42025=CARTESIAN_POINT('',(49.5605690039975,14.,108.6)) ;
#42026=CARTESIAN_POINT('Origin',(0.,0.,108.6)) ;
#42027=CARTESIAN_POINT('',(49.5605690039975,14.4,108.6)) ;
#42028=CARTESIAN_POINT('',(49.5605690039975,14.,108.6)) ;
#42029=CARTESIAN_POINT('',(49.4458289444115,14.4,108.6)) ;
#42030=CARTESIAN_POINT('',(0.,14.4,108.6)) ;
#42031=CARTESIAN_POINT('',(43.2232576282723,28.,108.6)) ;
#42032=CARTESIAN_POINT('Origin',(0.,0.,108.6)) ;
#42033=CARTESIAN_POINT('',(43.2232576282723,28.4,108.6)) ;
#42034=CARTESIAN_POINT('',(43.2232576282723,28.,108.6)) ;
#42035=CARTESIAN_POINT('',(0.,28.4,108.6)) ;
#42036=CARTESIAN_POINT('',(0.,14.4,108.6)) ;
#42037=CARTESIAN_POINT('',(50.4984158167363,0.4,108.6)) ;
#42038=CARTESIAN_POINT('Origin',(0.,0.,108.6)) ;
#42039=CARTESIAN_POINT('',(0.,0.4,108.6)) ;
#42040=CARTESIAN_POINT('',(48.6342471926933,-13.6,108.6)) ;
#42041=CARTESIAN_POINT('Origin',(0.,0.,108.6)) ;
#42042=CARTESIAN_POINT('',(0.,-13.6,108.6)) ;
#42043=CARTESIAN_POINT('Origin',(0.,0.,108.6)) ;
#42044=CARTESIAN_POINT('',(28.4,27.6,108.6)) ;
#42045=CARTESIAN_POINT('',(28.4,0.,108.6)) ;
#42046=CARTESIAN_POINT('',(0.,27.6,108.6)) ;
#42047=CARTESIAN_POINT('',(28.4,13.6,108.6)) ;
#42048=CARTESIAN_POINT('',(28.4,0.,108.6)) ;
#42049=CARTESIAN_POINT('',(0.,13.6,108.6)) ;
#42050=CARTESIAN_POINT('',(28.4,-0.4,108.6)) ;
#42051=CARTESIAN_POINT('',(28.4,0.,108.6)) ;
#42052=CARTESIAN_POINT('',(0.,-0.4,108.6)) ;
#42053=CARTESIAN_POINT('',(28.4,-14.4,108.6)) ;
#42054=CARTESIAN_POINT('',(28.4,0.,108.6)) ;
#42055=CARTESIAN_POINT('',(0.,-14.4,108.6)) ;
#42056=CARTESIAN_POINT('',(28.4,41.6,108.6)) ;
#42057=CARTESIAN_POINT('',(28.4,0.,108.6)) ;
#42058=CARTESIAN_POINT('',(28.6302287800849,41.6,108.6)) ;
#42059=CARTESIAN_POINT('',(0.,41.6,108.6)) ;
#42060=CARTESIAN_POINT('Origin',(0.,0.,108.6)) ;
#42061=CARTESIAN_POINT('',(14.4,42.4,108.6)) ;
#42062=CARTESIAN_POINT('',(14.4,48.4034089708566,108.6)) ;
#42063=CARTESIAN_POINT('',(14.4,0.,108.6)) ;
#42064=CARTESIAN_POINT('',(27.4315511774307,42.4,108.6)) ;
#42065=CARTESIAN_POINT('Origin',(0.,0.,108.6)) ;
#42066=CARTESIAN_POINT('',(0.,42.4,108.6)) ;
#42067=CARTESIAN_POINT('',(13.6,41.6,108.6)) ;
#42068=CARTESIAN_POINT('',(13.6,28.4,108.6)) ;
#42069=CARTESIAN_POINT('',(13.6,0.,108.6)) ;
#42070=CARTESIAN_POINT('',(0.4,28.4,108.6)) ;
#42071=CARTESIAN_POINT('',(0.,28.4,108.6)) ;
#42072=CARTESIAN_POINT('',(0.4,41.6,108.6)) ;
#42073=CARTESIAN_POINT('',(0.4,0.,108.6)) ;
#42074=CARTESIAN_POINT('',(0.,41.6,108.6)) ;
#42075=CARTESIAN_POINT('',(-0.4,41.6,108.6)) ;
#42076=CARTESIAN_POINT('',(-0.4,28.4,108.6)) ;
#42077=CARTESIAN_POINT('',(-0.4,0.,108.6)) ;
#42078=CARTESIAN_POINT('',(-13.6,28.4,108.6)) ;
#42079=CARTESIAN_POINT('',(0.,28.4,108.6)) ;
#42080=CARTESIAN_POINT('',(-13.6,41.6,108.6)) ;
#42081=CARTESIAN_POINT('',(-13.6,0.,108.6)) ;
#42082=CARTESIAN_POINT('',(0.,41.6,108.6)) ;
#42083=CARTESIAN_POINT('',(-14.4,41.6,108.6)) ;
#42084=CARTESIAN_POINT('',(-14.4,28.4,108.6)) ;
#42085=CARTESIAN_POINT('',(-14.4,0.,108.6)) ;
#42086=CARTESIAN_POINT('',(-27.6,28.4,108.6)) ;
#42087=CARTESIAN_POINT('',(0.,28.4,108.6)) ;
#42088=CARTESIAN_POINT('',(-27.6,41.6,108.6)) ;
#42089=CARTESIAN_POINT('',(-27.6,0.,108.6)) ;
#42090=CARTESIAN_POINT('',(0.,41.6,108.6)) ;
#42091=CARTESIAN_POINT('',(14.4,41.6,108.6)) ;
#42092=CARTESIAN_POINT('',(27.6,41.6,108.6)) ;
#42093=CARTESIAN_POINT('',(0.,41.6,108.6)) ;
#42094=CARTESIAN_POINT('',(27.6,28.4,108.6)) ;
#42095=CARTESIAN_POINT('',(27.6,0.,108.6)) ;
#42096=CARTESIAN_POINT('',(14.4,28.4,108.6)) ;
#42097=CARTESIAN_POINT('',(0.,28.4,108.6)) ;
#42098=CARTESIAN_POINT('',(14.4,0.,108.6)) ;
#42099=CARTESIAN_POINT('',(13.6,42.4,108.6)) ;
#42100=CARTESIAN_POINT('',(0.4,42.4,108.6)) ;
#42101=CARTESIAN_POINT('',(0.,42.4,108.6)) ;
#42102=CARTESIAN_POINT('',(0.4,50.4984158167363,108.6)) ;
#42103=CARTESIAN_POINT('',(0.4,0.,108.6)) ;
#42104=CARTESIAN_POINT('',(13.6,48.6342471926933,108.6)) ;
#42105=CARTESIAN_POINT('Origin',(0.,0.,108.6)) ;
#42106=CARTESIAN_POINT('',(13.6,0.,108.6)) ;
#42107=CARTESIAN_POINT('',(-0.4,42.4,108.6)) ;
#42108=CARTESIAN_POINT('',(-13.6,42.4,108.6)) ;
#42109=CARTESIAN_POINT('',(0.,42.4,108.6)) ;
#42110=CARTESIAN_POINT('',(-13.6,48.6342471926933,108.6)) ;
#42111=CARTESIAN_POINT('',(-13.6,0.,108.6)) ;
#42112=CARTESIAN_POINT('',(-0.4,50.4984158167363,108.6)) ;
#42113=CARTESIAN_POINT('Origin',(0.,0.,108.6)) ;
#42114=CARTESIAN_POINT('',(-0.4,0.,108.6)) ;
#42115=CARTESIAN_POINT('',(-28.4,41.6,108.6)) ;
#42116=CARTESIAN_POINT('',(-28.4,28.4,108.6)) ;
#42117=CARTESIAN_POINT('',(-28.4,0.,108.6)) ;
#42118=CARTESIAN_POINT('',(-41.6,28.4,108.6)) ;
#42119=CARTESIAN_POINT('',(0.,28.4,108.6)) ;
#42120=CARTESIAN_POINT('',(-41.6,28.6302287800849,108.6)) ;
#42121=CARTESIAN_POINT('',(-41.6,0.,108.6)) ;
#42122=CARTESIAN_POINT('',(-28.6302287800849,41.6,108.6)) ;
#42123=CARTESIAN_POINT('Origin',(0.,0.,108.6)) ;
#42124=CARTESIAN_POINT('',(0.,41.6,108.6)) ;
#42125=CARTESIAN_POINT('',(-14.4,42.4,108.6)) ;
#42126=CARTESIAN_POINT('',(-27.4315511774307,42.4,108.6)) ;
#42127=CARTESIAN_POINT('',(0.,42.4,108.6)) ;
#42128=CARTESIAN_POINT('',(-14.4,48.4034089708566,108.6)) ;
#42129=CARTESIAN_POINT('Origin',(0.,0.,108.6)) ;
#42130=CARTESIAN_POINT('',(-14.4,0.,108.6)) ;
#42131=CARTESIAN_POINT('',(-0.4,-50.4984158167363,108.6)) ;
#42132=CARTESIAN_POINT('',(-13.6,-48.6342471926933,108.6)) ;
#42133=CARTESIAN_POINT('Origin',(0.,0.,108.6)) ;
#42134=CARTESIAN_POINT('',(-13.6,-42.4,108.6)) ;
#42135=CARTESIAN_POINT('',(-13.6,0.,108.6)) ;
#42136=CARTESIAN_POINT('',(-0.4,-42.4,108.6)) ;
#42137=CARTESIAN_POINT('',(0.,-42.4,108.6)) ;
#42138=CARTESIAN_POINT('',(-0.4,0.,108.6)) ;
#42139=CARTESIAN_POINT('',(-0.4,-0.4,108.6)) ;
#42140=CARTESIAN_POINT('',(-0.4,-13.6,108.6)) ;
#42141=CARTESIAN_POINT('',(-0.4,0.,108.6)) ;
#42142=CARTESIAN_POINT('',(-13.6,-13.6,108.6)) ;
#42143=CARTESIAN_POINT('',(0.,-13.6,108.6)) ;
#42144=CARTESIAN_POINT('',(-13.6,-0.4,108.6)) ;
#42145=CARTESIAN_POINT('',(-13.6,0.,108.6)) ;
#42146=CARTESIAN_POINT('',(0.,-0.4,108.6)) ;
#42147=CARTESIAN_POINT('',(-0.4,-14.4,108.6)) ;
#42148=CARTESIAN_POINT('',(-0.4,-27.6,108.6)) ;
#42149=CARTESIAN_POINT('',(-0.4,0.,108.6)) ;
#42150=CARTESIAN_POINT('',(-13.6,-27.6,108.6)) ;
#42151=CARTESIAN_POINT('',(0.,-27.6,108.6)) ;
#42152=CARTESIAN_POINT('',(-13.6,-14.4,108.6)) ;
#42153=CARTESIAN_POINT('',(-13.6,0.,108.6)) ;
#42154=CARTESIAN_POINT('',(0.,-14.4,108.6)) ;
#42155=CARTESIAN_POINT('',(-0.4,-28.4,108.6)) ;
#42156=CARTESIAN_POINT('',(-0.4,-41.6,108.6)) ;
#42157=CARTESIAN_POINT('',(-0.4,0.,108.6)) ;
#42158=CARTESIAN_POINT('',(-13.6,-41.6,108.6)) ;
#42159=CARTESIAN_POINT('',(0.,-41.6,108.6)) ;
#42160=CARTESIAN_POINT('',(-13.6,-28.4,108.6)) ;
#42161=CARTESIAN_POINT('',(-13.6,0.,108.6)) ;
#42162=CARTESIAN_POINT('',(0.,-28.4,108.6)) ;
#42163=CARTESIAN_POINT('',(-14.4,-0.4,108.6)) ;
#42164=CARTESIAN_POINT('',(-14.4,-13.6,108.6)) ;
#42165=CARTESIAN_POINT('',(-14.4,0.,108.6)) ;
#42166=CARTESIAN_POINT('',(-27.6,-13.6,108.6)) ;
#42167=CARTESIAN_POINT('',(0.,-13.6,108.6)) ;
#42168=CARTESIAN_POINT('',(-27.6,-0.4,108.6)) ;
#42169=CARTESIAN_POINT('',(-27.6,0.,108.6)) ;
#42170=CARTESIAN_POINT('',(0.,-0.4,108.6)) ;
#42171=CARTESIAN_POINT('',(-28.4,-0.4,108.6)) ;
#42172=CARTESIAN_POINT('',(-28.4,-13.6,108.6)) ;
#42173=CARTESIAN_POINT('',(-28.4,0.,108.6)) ;
#42174=CARTESIAN_POINT('',(-41.6,-13.6,108.6)) ;
#42175=CARTESIAN_POINT('',(0.,-13.6,108.6)) ;
#42176=CARTESIAN_POINT('',(-41.6,-0.4,108.6)) ;
#42177=CARTESIAN_POINT('',(-41.6,0.,108.6)) ;
#42178=CARTESIAN_POINT('',(0.,-0.4,108.6)) ;
#42179=CARTESIAN_POINT('',(-42.4,-0.4,108.6)) ;
#42180=CARTESIAN_POINT('',(-42.4,-13.6,108.6)) ;
#42181=CARTESIAN_POINT('',(-42.4,0.,108.6)) ;
#42182=CARTESIAN_POINT('',(-48.6342471926933,-13.6,108.6)) ;
#42183=CARTESIAN_POINT('',(0.,-13.6,108.6)) ;
#42184=CARTESIAN_POINT('',(-50.4984158167363,-0.4,108.6)) ;
#42185=CARTESIAN_POINT('Origin',(0.,0.,108.6)) ;
#42186=CARTESIAN_POINT('',(0.,-0.4,108.6)) ;
#42187=CARTESIAN_POINT('',(-14.4,-28.4,108.6)) ;
#42188=CARTESIAN_POINT('',(-14.4,-41.6,108.6)) ;
#42189=CARTESIAN_POINT('',(-14.4,0.,108.6)) ;
#42190=CARTESIAN_POINT('',(-27.6,-41.6,108.6)) ;
#42191=CARTESIAN_POINT('',(0.,-41.6,108.6)) ;
#42192=CARTESIAN_POINT('',(-27.6,-28.4,108.6)) ;
#42193=CARTESIAN_POINT('',(-27.6,0.,108.6)) ;
#42194=CARTESIAN_POINT('',(0.,-28.4,108.6)) ;
#42195=CARTESIAN_POINT('',(-14.4,-14.4,108.6)) ;
#42196=CARTESIAN_POINT('',(-14.4,-27.6,108.6)) ;
#42197=CARTESIAN_POINT('',(-14.4,0.,108.6)) ;
#42198=CARTESIAN_POINT('',(-27.6,-27.6,108.6)) ;
#42199=CARTESIAN_POINT('',(0.,-27.6,108.6)) ;
#42200=CARTESIAN_POINT('',(-27.6,-14.4,108.6)) ;
#42201=CARTESIAN_POINT('',(-27.6,0.,108.6)) ;
#42202=CARTESIAN_POINT('',(0.,-14.4,108.6)) ;
#42203=CARTESIAN_POINT('',(-14.4,-42.4,108.6)) ;
#42204=CARTESIAN_POINT('',(-14.4,-48.4034089708566,108.6)) ;
#42205=CARTESIAN_POINT('',(-14.4,0.,108.6)) ;
#42206=CARTESIAN_POINT('',(-27.4315511774307,-42.4,108.6)) ;
#42207=CARTESIAN_POINT('Origin',(0.,0.,108.6)) ;
#42208=CARTESIAN_POINT('',(0.,-42.4,108.6)) ;
#42209=CARTESIAN_POINT('',(-28.4,-28.4,108.6)) ;
#42210=CARTESIAN_POINT('',(-28.4,-41.6,108.6)) ;
#42211=CARTESIAN_POINT('',(-28.4,0.,108.6)) ;
#42212=CARTESIAN_POINT('',(-28.6302287800849,-41.6,108.6)) ;
#42213=CARTESIAN_POINT('',(0.,-41.6,108.6)) ;
#42214=CARTESIAN_POINT('',(-41.6,-28.6302287800849,108.6)) ;
#42215=CARTESIAN_POINT('Origin',(0.,0.,108.6)) ;
#42216=CARTESIAN_POINT('',(-41.6,-28.4,108.6)) ;
#42217=CARTESIAN_POINT('',(-41.6,0.,108.6)) ;
#42218=CARTESIAN_POINT('',(0.,-28.4,108.6)) ;
#42219=CARTESIAN_POINT('',(-42.4,-14.4,108.6)) ;
#42220=CARTESIAN_POINT('',(-42.4,-27.4315511774307,108.6)) ;
#42221=CARTESIAN_POINT('',(-42.4,0.,108.6)) ;
#42222=CARTESIAN_POINT('',(-48.4034089708566,-14.4,108.6)) ;
#42223=CARTESIAN_POINT('Origin',(0.,0.,108.6)) ;
#42224=CARTESIAN_POINT('',(0.,-14.4,108.6)) ;
#42225=CARTESIAN_POINT('',(-28.4,-14.4,108.6)) ;
#42226=CARTESIAN_POINT('',(-28.4,-27.6,108.6)) ;
#42227=CARTESIAN_POINT('',(-28.4,0.,108.6)) ;
#42228=CARTESIAN_POINT('',(-41.6,-27.6,108.6)) ;
#42229=CARTESIAN_POINT('',(0.,-27.6,108.6)) ;
#42230=CARTESIAN_POINT('',(-41.6,-14.4,108.6)) ;
#42231=CARTESIAN_POINT('',(-41.6,0.,108.6)) ;
#42232=CARTESIAN_POINT('',(0.,-14.4,108.6)) ;
#42233=CARTESIAN_POINT('',(-42.4,14.4,108.6)) ;
#42234=CARTESIAN_POINT('',(-48.4034089708566,14.4,108.6)) ;
#42235=CARTESIAN_POINT('',(0.,14.4,108.6)) ;
#42236=CARTESIAN_POINT('',(-42.4,27.4315511774307,108.6)) ;
#42237=CARTESIAN_POINT('Origin',(0.,0.,108.6)) ;
#42238=CARTESIAN_POINT('',(-42.4,0.,108.6)) ;
#42239=CARTESIAN_POINT('',(-42.4,13.6,108.6)) ;
#42240=CARTESIAN_POINT('',(-42.4,0.4,108.6)) ;
#42241=CARTESIAN_POINT('',(-42.4,0.,108.6)) ;
#42242=CARTESIAN_POINT('',(-50.4984158167363,0.4,108.6)) ;
#42243=CARTESIAN_POINT('',(0.,0.4,108.6)) ;
#42244=CARTESIAN_POINT('',(-48.6342471926933,13.6,108.6)) ;
#42245=CARTESIAN_POINT('Origin',(0.,0.,108.6)) ;
#42246=CARTESIAN_POINT('',(0.,13.6,108.6)) ;
#42247=CARTESIAN_POINT('',(-28.4,13.6,108.6)) ;
#42248=CARTESIAN_POINT('',(-28.4,0.4,108.6)) ;
#42249=CARTESIAN_POINT('',(-28.4,0.,108.6)) ;
#42250=CARTESIAN_POINT('',(-41.6,0.4,108.6)) ;
#42251=CARTESIAN_POINT('',(0.,0.4,108.6)) ;
#42252=CARTESIAN_POINT('',(-41.6,13.6,108.6)) ;
#42253=CARTESIAN_POINT('',(-41.6,0.,108.6)) ;
#42254=CARTESIAN_POINT('',(0.,13.6,108.6)) ;
#42255=CARTESIAN_POINT('',(-14.4,13.6,108.6)) ;
#42256=CARTESIAN_POINT('',(-14.4,0.4,108.6)) ;
#42257=CARTESIAN_POINT('',(-14.4,0.,108.6)) ;
#42258=CARTESIAN_POINT('',(-27.6,0.4,108.6)) ;
#42259=CARTESIAN_POINT('',(0.,0.4,108.6)) ;
#42260=CARTESIAN_POINT('',(-27.6,13.6,108.6)) ;
#42261=CARTESIAN_POINT('',(-27.6,0.,108.6)) ;
#42262=CARTESIAN_POINT('',(0.,13.6,108.6)) ;
#42263=CARTESIAN_POINT('',(-0.4,13.6,108.6)) ;
#42264=CARTESIAN_POINT('',(-0.4,0.4,108.6)) ;
#42265=CARTESIAN_POINT('',(-0.4,0.,108.6)) ;
#42266=CARTESIAN_POINT('',(-13.6,0.4,108.6)) ;
#42267=CARTESIAN_POINT('',(0.,0.4,108.6)) ;
#42268=CARTESIAN_POINT('',(-13.6,13.6,108.6)) ;
#42269=CARTESIAN_POINT('',(-13.6,0.,108.6)) ;
#42270=CARTESIAN_POINT('',(0.,13.6,108.6)) ;
#42271=CARTESIAN_POINT('',(13.6,-28.4,108.6)) ;
#42272=CARTESIAN_POINT('',(13.6,-41.6,108.6)) ;
#42273=CARTESIAN_POINT('',(13.6,0.,108.6)) ;
#42274=CARTESIAN_POINT('',(0.4,-41.6,108.6)) ;
#42275=CARTESIAN_POINT('',(0.,-41.6,108.6)) ;
#42276=CARTESIAN_POINT('',(0.4,-28.4,108.6)) ;
#42277=CARTESIAN_POINT('',(0.4,0.,108.6)) ;
#42278=CARTESIAN_POINT('',(0.,-28.4,108.6)) ;
#42279=CARTESIAN_POINT('',(13.6,-14.4,108.6)) ;
#42280=CARTESIAN_POINT('',(13.6,-27.6,108.6)) ;
#42281=CARTESIAN_POINT('',(13.6,0.,108.6)) ;
#42282=CARTESIAN_POINT('',(0.4,-27.6,108.6)) ;
#42283=CARTESIAN_POINT('',(0.,-27.6,108.6)) ;
#42284=CARTESIAN_POINT('',(0.4,-14.4,108.6)) ;
#42285=CARTESIAN_POINT('',(0.4,0.,108.6)) ;
#42286=CARTESIAN_POINT('',(0.,-14.4,108.6)) ;
#42287=CARTESIAN_POINT('',(13.6,-0.4,108.6)) ;
#42288=CARTESIAN_POINT('',(13.6,-13.6,108.6)) ;
#42289=CARTESIAN_POINT('',(13.6,0.,108.6)) ;
#42290=CARTESIAN_POINT('',(0.4,-13.6,108.6)) ;
#42291=CARTESIAN_POINT('',(0.,-13.6,108.6)) ;
#42292=CARTESIAN_POINT('',(0.4,-0.4,108.6)) ;
#42293=CARTESIAN_POINT('',(0.4,0.,108.6)) ;
#42294=CARTESIAN_POINT('',(0.,-0.4,108.6)) ;
#42295=CARTESIAN_POINT('',(14.4,-48.4034089708566,108.6)) ;
#42296=CARTESIAN_POINT('',(14.4,-42.4,108.6)) ;
#42297=CARTESIAN_POINT('',(14.4,0.,108.6)) ;
#42298=CARTESIAN_POINT('',(27.4315511774307,-42.4,108.6)) ;
#42299=CARTESIAN_POINT('',(0.,-42.4,108.6)) ;
#42300=CARTESIAN_POINT('Origin',(0.,0.,108.6)) ;
#42301=CARTESIAN_POINT('',(13.6,13.6,108.6)) ;
#42302=CARTESIAN_POINT('',(13.6,0.4,108.6)) ;
#42303=CARTESIAN_POINT('',(13.6,0.,108.6)) ;
#42304=CARTESIAN_POINT('',(0.4,0.4,108.6)) ;
#42305=CARTESIAN_POINT('',(0.,0.4,108.6)) ;
#42306=CARTESIAN_POINT('',(0.4,13.6,108.6)) ;
#42307=CARTESIAN_POINT('',(0.4,0.,108.6)) ;
#42308=CARTESIAN_POINT('',(0.,13.6,108.6)) ;
#42309=CARTESIAN_POINT('',(13.6,-48.6342471926933,108.6)) ;
#42310=CARTESIAN_POINT('',(0.4,-50.4984158167363,108.6)) ;
#42311=CARTESIAN_POINT('Origin',(0.,0.,108.6)) ;
#42312=CARTESIAN_POINT('',(0.4,-42.4,108.6)) ;
#42313=CARTESIAN_POINT('',(0.4,0.,108.6)) ;
#42314=CARTESIAN_POINT('',(13.6,-42.4,108.6)) ;
#42315=CARTESIAN_POINT('',(0.,-42.4,108.6)) ;
#42316=CARTESIAN_POINT('',(13.6,0.,108.6)) ;
#42317=CARTESIAN_POINT('',(-41.6,27.6,108.6)) ;
#42318=CARTESIAN_POINT('',(-28.4,27.6,108.6)) ;
#42319=CARTESIAN_POINT('',(0.,27.6,108.6)) ;
#42320=CARTESIAN_POINT('',(-28.4,14.4,108.6)) ;
#42321=CARTESIAN_POINT('',(-28.4,0.,108.6)) ;
#42322=CARTESIAN_POINT('',(-41.6,14.4,108.6)) ;
#42323=CARTESIAN_POINT('',(0.,14.4,108.6)) ;
#42324=CARTESIAN_POINT('',(-41.6,0.,108.6)) ;
#42325=CARTESIAN_POINT('',(-14.4,27.6,108.6)) ;
#42326=CARTESIAN_POINT('',(-14.4,14.4,108.6)) ;
#42327=CARTESIAN_POINT('',(-14.4,0.,108.6)) ;
#42328=CARTESIAN_POINT('',(-27.6,14.4,108.6)) ;
#42329=CARTESIAN_POINT('',(0.,14.4,108.6)) ;
#42330=CARTESIAN_POINT('',(-27.6,27.6,108.6)) ;
#42331=CARTESIAN_POINT('',(-27.6,0.,108.6)) ;
#42332=CARTESIAN_POINT('',(0.,27.6,108.6)) ;
#42333=CARTESIAN_POINT('',(-0.4,27.6,108.6)) ;
#42334=CARTESIAN_POINT('',(-0.4,14.4,108.6)) ;
#42335=CARTESIAN_POINT('',(-0.4,0.,108.6)) ;
#42336=CARTESIAN_POINT('',(-13.6,14.4,108.6)) ;
#42337=CARTESIAN_POINT('',(0.,14.4,108.6)) ;
#42338=CARTESIAN_POINT('',(-13.6,27.6,108.6)) ;
#42339=CARTESIAN_POINT('',(-13.6,0.,108.6)) ;
#42340=CARTESIAN_POINT('',(0.,27.6,108.6)) ;
#42341=CARTESIAN_POINT('',(13.6,27.6,108.6)) ;
#42342=CARTESIAN_POINT('',(13.6,14.4,108.6)) ;
#42343=CARTESIAN_POINT('',(13.6,0.,108.6)) ;
#42344=CARTESIAN_POINT('',(0.4,14.4,108.6)) ;
#42345=CARTESIAN_POINT('',(0.,14.4,108.6)) ;
#42346=CARTESIAN_POINT('',(0.4,27.6,108.6)) ;
#42347=CARTESIAN_POINT('',(0.4,0.,108.6)) ;
#42348=CARTESIAN_POINT('',(0.,27.6,108.6)) ;
#42349=CARTESIAN_POINT('',(27.6,-28.4,108.6)) ;
#42350=CARTESIAN_POINT('',(27.6,-41.6,108.6)) ;
#42351=CARTESIAN_POINT('',(27.6,0.,108.6)) ;
#42352=CARTESIAN_POINT('',(14.4,-41.6,108.6)) ;
#42353=CARTESIAN_POINT('',(0.,-41.6,108.6)) ;
#42354=CARTESIAN_POINT('',(14.4,-28.4,108.6)) ;
#42355=CARTESIAN_POINT('',(14.4,0.,108.6)) ;
#42356=CARTESIAN_POINT('',(0.,-28.4,108.6)) ;
#42357=CARTESIAN_POINT('',(27.6,-14.4,108.6)) ;
#42358=CARTESIAN_POINT('',(27.6,-27.6,108.6)) ;
#42359=CARTESIAN_POINT('',(27.6,0.,108.6)) ;
#42360=CARTESIAN_POINT('',(14.4,-27.6,108.6)) ;
#42361=CARTESIAN_POINT('',(0.,-27.6,108.6)) ;
#42362=CARTESIAN_POINT('',(14.4,-14.4,108.6)) ;
#42363=CARTESIAN_POINT('',(14.4,0.,108.6)) ;
#42364=CARTESIAN_POINT('',(0.,-14.4,108.6)) ;
#42365=CARTESIAN_POINT('',(27.6,-0.4,108.6)) ;
#42366=CARTESIAN_POINT('',(27.6,-13.6,108.6)) ;
#42367=CARTESIAN_POINT('',(27.6,0.,108.6)) ;
#42368=CARTESIAN_POINT('',(14.4,-13.6,108.6)) ;
#42369=CARTESIAN_POINT('',(0.,-13.6,108.6)) ;
#42370=CARTESIAN_POINT('',(14.4,-0.4,108.6)) ;
#42371=CARTESIAN_POINT('',(14.4,0.,108.6)) ;
#42372=CARTESIAN_POINT('',(0.,-0.4,108.6)) ;
#42373=CARTESIAN_POINT('',(27.6,13.6,108.6)) ;
#42374=CARTESIAN_POINT('',(27.6,0.4,108.6)) ;
#42375=CARTESIAN_POINT('',(27.6,0.,108.6)) ;
#42376=CARTESIAN_POINT('',(14.4,0.4,108.6)) ;
#42377=CARTESIAN_POINT('',(0.,0.4,108.6)) ;
#42378=CARTESIAN_POINT('',(14.4,13.6,108.6)) ;
#42379=CARTESIAN_POINT('',(14.4,0.,108.6)) ;
#42380=CARTESIAN_POINT('',(0.,13.6,108.6)) ;
#42381=CARTESIAN_POINT('',(27.6,27.6,108.6)) ;
#42382=CARTESIAN_POINT('',(27.6,14.4,108.6)) ;
#42383=CARTESIAN_POINT('',(27.6,0.,108.6)) ;
#42384=CARTESIAN_POINT('',(14.4,14.4,108.6)) ;
#42385=CARTESIAN_POINT('',(0.,14.4,108.6)) ;
#42386=CARTESIAN_POINT('',(14.4,27.6,108.6)) ;
#42387=CARTESIAN_POINT('',(14.4,0.,108.6)) ;
#42388=CARTESIAN_POINT('',(0.,27.6,108.6)) ;
#42389=CARTESIAN_POINT('',(28.6302287800849,-41.6,108.6)) ;
#42390=CARTESIAN_POINT('Origin',(0.,0.,108.6)) ;
#42391=CARTESIAN_POINT('',(28.4,-41.6,108.6)) ;
#42392=CARTESIAN_POINT('',(0.,-41.6,108.6)) ;
#42393=CARTESIAN_POINT('',(28.4,-28.4,108.6)) ;
#42394=CARTESIAN_POINT('',(28.4,0.,108.6)) ;
#42395=CARTESIAN_POINT('',(0.,-28.4,108.6)) ;
#42396=CARTESIAN_POINT('Origin',(0.,0.,108.3)) ;
#42397=CARTESIAN_POINT('',(28.6302287800849,-41.6,108.)) ;
#42398=CARTESIAN_POINT('Origin',(0.,0.,108.)) ;
#42399=CARTESIAN_POINT('',(28.6302287800849,-41.6,108.3)) ;
#42400=CARTESIAN_POINT('Origin',(0.,0.,108.)) ;
#42401=CARTESIAN_POINT('',(43.2232576282723,28.4,108.)) ;
#42402=CARTESIAN_POINT('',(0.,28.4,108.)) ;
#42403=CARTESIAN_POINT('',(43.2232576282723,28.,108.)) ;
#42404=CARTESIAN_POINT('',(43.2232576282723,28.,108.)) ;
#42405=CARTESIAN_POINT('',(49.4458289444115,14.4,108.)) ;
#42406=CARTESIAN_POINT('Origin',(0.,0.,108.)) ;
#42407=CARTESIAN_POINT('',(49.5605690039975,14.4,108.)) ;
#42408=CARTESIAN_POINT('',(0.,14.4,108.)) ;
#42409=CARTESIAN_POINT('',(49.5605690039975,14.,108.)) ;
#42410=CARTESIAN_POINT('',(49.5605690039975,14.,108.)) ;
#42411=CARTESIAN_POINT('',(51.4984465785134,0.4,108.)) ;
#42412=CARTESIAN_POINT('Origin',(0.,0.,108.)) ;
#42413=CARTESIAN_POINT('',(51.5,0.4,108.)) ;
#42414=CARTESIAN_POINT('',(0.,0.4,108.)) ;
#42415=CARTESIAN_POINT('',(51.5,-0.4,108.)) ;
#42416=CARTESIAN_POINT('',(51.5,0.,108.)) ;
#42417=CARTESIAN_POINT('',(51.4984465785134,-0.4,108.)) ;
#42418=CARTESIAN_POINT('',(0.,-0.4,108.)) ;
#42419=CARTESIAN_POINT('',(49.5605690039975,-14.,108.)) ;
#42420=CARTESIAN_POINT('Origin',(0.,0.,108.)) ;
#42421=CARTESIAN_POINT('',(49.5605690039975,-14.4,108.)) ;
#42422=CARTESIAN_POINT('',(49.5605690039975,-14.,108.)) ;
#42423=CARTESIAN_POINT('',(49.4458289444115,-14.4,108.)) ;
#42424=CARTESIAN_POINT('',(0.,-14.4,108.)) ;
#42425=CARTESIAN_POINT('',(43.2232576282723,-28.,108.)) ;
#42426=CARTESIAN_POINT('Origin',(0.,0.,108.)) ;
#42427=CARTESIAN_POINT('',(43.2232576282723,-28.4,108.)) ;
#42428=CARTESIAN_POINT('',(43.2232576282723,-28.,108.)) ;
#42429=CARTESIAN_POINT('',(42.9614943874163,-28.4,108.)) ;
#42430=CARTESIAN_POINT('',(0.,-28.4,108.)) ;
#42431=CARTESIAN_POINT('Origin',(0.,0.,108.)) ;
#42432=CARTESIAN_POINT('',(29.8035232816525,-42.,108.)) ;
#42433=CARTESIAN_POINT('Origin',(0.,0.,108.)) ;
#42434=CARTESIAN_POINT('',(29.8035232816525,-42.4,108.)) ;
#42435=CARTESIAN_POINT('',(29.8035232816525,-42.,108.)) ;
#42436=CARTESIAN_POINT('',(29.2316609175736,-42.4,108.)) ;
#42437=CARTESIAN_POINT('',(0.,-42.4,108.)) ;
#42438=CARTESIAN_POINT('',(28.4,-42.9614943874163,108.)) ;
#42439=CARTESIAN_POINT('Origin',(0.,0.,108.)) ;
#42440=CARTESIAN_POINT('',(28.4,-43.2232576282723,108.)) ;
#42441=CARTESIAN_POINT('',(28.4,0.,108.)) ;
#42442=CARTESIAN_POINT('',(28.,-43.2232576282723,108.)) ;
#42443=CARTESIAN_POINT('',(28.,-43.2232576282723,108.)) ;
#42444=CARTESIAN_POINT('',(14.4,-49.4458289444115,108.)) ;
#42445=CARTESIAN_POINT('Origin',(0.,0.,108.)) ;
#42446=CARTESIAN_POINT('',(14.4,-49.5605690039975,108.)) ;
#42447=CARTESIAN_POINT('',(14.4,0.,108.)) ;
#42448=CARTESIAN_POINT('',(14.,-49.5605690039975,108.)) ;
#42449=CARTESIAN_POINT('',(14.,-49.5605690039975,108.)) ;
#42450=CARTESIAN_POINT('',(0.4,-51.4984465785134,108.)) ;
#42451=CARTESIAN_POINT('Origin',(0.,0.,108.)) ;
#42452=CARTESIAN_POINT('',(0.4,-51.5,108.)) ;
#42453=CARTESIAN_POINT('',(0.4,0.,108.)) ;
#42454=CARTESIAN_POINT('',(-0.4,-51.5,108.)) ;
#42455=CARTESIAN_POINT('',(0.,-51.5,108.)) ;
#42456=CARTESIAN_POINT('',(-0.4,-51.4984465785134,108.)) ;
#42457=CARTESIAN_POINT('',(-0.4,0.,108.)) ;
#42458=CARTESIAN_POINT('',(-14.,-49.5605690039975,108.)) ;
#42459=CARTESIAN_POINT('Origin',(0.,0.,108.)) ;
#42460=CARTESIAN_POINT('',(-14.4,-49.5605690039975,108.)) ;
#42461=CARTESIAN_POINT('',(-14.,-49.5605690039975,108.)) ;
#42462=CARTESIAN_POINT('',(-14.4,-49.4458289444115,108.)) ;
#42463=CARTESIAN_POINT('',(-14.4,0.,108.)) ;
#42464=CARTESIAN_POINT('',(-28.,-43.2232576282723,108.)) ;
#42465=CARTESIAN_POINT('Origin',(0.,0.,108.)) ;
#42466=CARTESIAN_POINT('',(-28.4,-43.2232576282723,108.)) ;
#42467=CARTESIAN_POINT('',(-28.,-43.2232576282723,108.)) ;
#42468=CARTESIAN_POINT('',(-28.4,-42.9614943874163,108.)) ;
#42469=CARTESIAN_POINT('',(-28.4,0.,108.)) ;
#42470=CARTESIAN_POINT('',(-29.2316609175736,-42.4,108.)) ;
#42471=CARTESIAN_POINT('Origin',(0.,0.,108.)) ;
#42472=CARTESIAN_POINT('',(-29.8035232816525,-42.4,108.)) ;
#42473=CARTESIAN_POINT('',(0.,-42.4,108.)) ;
#42474=CARTESIAN_POINT('',(-29.8035232816525,-42.,108.)) ;
#42475=CARTESIAN_POINT('',(-29.8035232816525,-42.,108.)) ;
#42476=CARTESIAN_POINT('',(-42.,-29.8035232816525,108.)) ;
#42477=CARTESIAN_POINT('Origin',(0.,0.,108.)) ;
#42478=CARTESIAN_POINT('',(-42.4,-29.8035232816525,108.)) ;
#42479=CARTESIAN_POINT('',(-42.,-29.8035232816525,108.)) ;
#42480=CARTESIAN_POINT('',(-42.4,-29.2316609175736,108.)) ;
#42481=CARTESIAN_POINT('',(-42.4,0.,108.)) ;
#42482=CARTESIAN_POINT('',(-42.9614943874163,-28.4,108.)) ;
#42483=CARTESIAN_POINT('Origin',(0.,0.,108.)) ;
#42484=CARTESIAN_POINT('',(-43.2232576282723,-28.4,108.)) ;
#42485=CARTESIAN_POINT('',(0.,-28.4,108.)) ;
#42486=CARTESIAN_POINT('',(-43.2232576282723,-28.,108.)) ;
#42487=CARTESIAN_POINT('',(-43.2232576282723,-28.,108.)) ;
#42488=CARTESIAN_POINT('',(-49.4458289444115,-14.4,108.)) ;
#42489=CARTESIAN_POINT('Origin',(0.,0.,108.)) ;
#42490=CARTESIAN_POINT('',(-49.5605690039975,-14.4,108.)) ;
#42491=CARTESIAN_POINT('',(0.,-14.4,108.)) ;
#42492=CARTESIAN_POINT('',(-49.5605690039975,-14.,108.)) ;
#42493=CARTESIAN_POINT('',(-49.5605690039975,-14.,108.)) ;
#42494=CARTESIAN_POINT('',(-51.4984465785134,-0.4,108.)) ;
#42495=CARTESIAN_POINT('Origin',(0.,0.,108.)) ;
#42496=CARTESIAN_POINT('',(-51.5,-0.4,108.)) ;
#42497=CARTESIAN_POINT('',(0.,-0.4,108.)) ;
#42498=CARTESIAN_POINT('',(-51.5,0.4,108.)) ;
#42499=CARTESIAN_POINT('',(-51.5,0.,108.)) ;
#42500=CARTESIAN_POINT('',(-51.4984465785134,0.4,108.)) ;
#42501=CARTESIAN_POINT('',(0.,0.4,108.)) ;
#42502=CARTESIAN_POINT('',(-49.5605690039975,14.,108.)) ;
#42503=CARTESIAN_POINT('Origin',(0.,0.,108.)) ;
#42504=CARTESIAN_POINT('',(-49.5605690039975,14.4,108.)) ;
#42505=CARTESIAN_POINT('',(-49.5605690039975,14.,108.)) ;
#42506=CARTESIAN_POINT('',(-49.4458289444115,14.4,108.)) ;
#42507=CARTESIAN_POINT('',(0.,14.4,108.)) ;
#42508=CARTESIAN_POINT('',(-43.2232576282723,28.,108.)) ;
#42509=CARTESIAN_POINT('Origin',(0.,0.,108.)) ;
#42510=CARTESIAN_POINT('',(-43.2232576282723,28.4,108.)) ;
#42511=CARTESIAN_POINT('',(-43.2232576282723,28.,108.)) ;
#42512=CARTESIAN_POINT('',(-42.9614943874163,28.4,108.)) ;
#42513=CARTESIAN_POINT('',(0.,28.4,108.)) ;
#42514=CARTESIAN_POINT('',(-42.4,29.2316609175736,108.)) ;
#42515=CARTESIAN_POINT('Origin',(0.,0.,108.)) ;
#42516=CARTESIAN_POINT('',(-42.4,29.8035232816525,108.)) ;
#42517=CARTESIAN_POINT('',(-42.4,0.,108.)) ;
#42518=CARTESIAN_POINT('',(-42.,29.8035232816525,108.)) ;
#42519=CARTESIAN_POINT('',(-42.,29.8035232816525,108.)) ;
#42520=CARTESIAN_POINT('',(-29.8035232816525,42.,108.)) ;
#42521=CARTESIAN_POINT('Origin',(0.,0.,108.)) ;
#42522=CARTESIAN_POINT('',(-29.8035232816525,42.4,108.)) ;
#42523=CARTESIAN_POINT('',(-29.8035232816525,42.,108.)) ;
#42524=CARTESIAN_POINT('',(-29.2316609175736,42.4,108.)) ;
#42525=CARTESIAN_POINT('',(0.,42.4,108.)) ;
#42526=CARTESIAN_POINT('',(-28.4,42.9614943874163,108.)) ;
#42527=CARTESIAN_POINT('Origin',(0.,0.,108.)) ;
#42528=CARTESIAN_POINT('',(-28.4,43.2232576282723,108.)) ;
#42529=CARTESIAN_POINT('',(-28.4,0.,108.)) ;
#42530=CARTESIAN_POINT('',(-28.,43.2232576282723,108.)) ;
#42531=CARTESIAN_POINT('',(-28.,43.2232576282723,108.)) ;
#42532=CARTESIAN_POINT('',(-14.4,49.4458289444115,108.)) ;
#42533=CARTESIAN_POINT('Origin',(0.,0.,108.)) ;
#42534=CARTESIAN_POINT('',(-14.4,49.5605690039975,108.)) ;
#42535=CARTESIAN_POINT('',(-14.4,0.,108.)) ;
#42536=CARTESIAN_POINT('',(-14.,49.5605690039975,108.)) ;
#42537=CARTESIAN_POINT('',(-14.,49.5605690039975,108.)) ;
#42538=CARTESIAN_POINT('',(-0.4,51.4984465785134,108.)) ;
#42539=CARTESIAN_POINT('Origin',(0.,0.,108.)) ;
#42540=CARTESIAN_POINT('',(-0.4,51.5,108.)) ;
#42541=CARTESIAN_POINT('',(-0.4,0.,108.)) ;
#42542=CARTESIAN_POINT('',(0.4,51.5,108.)) ;
#42543=CARTESIAN_POINT('',(0.,51.5,108.)) ;
#42544=CARTESIAN_POINT('',(0.4,51.4984465785134,108.)) ;
#42545=CARTESIAN_POINT('',(0.4,0.,108.)) ;
#42546=CARTESIAN_POINT('',(14.,49.5605690039975,108.)) ;
#42547=CARTESIAN_POINT('Origin',(0.,0.,108.)) ;
#42548=CARTESIAN_POINT('',(14.4,49.5605690039975,108.)) ;
#42549=CARTESIAN_POINT('',(14.,49.5605690039975,108.)) ;
#42550=CARTESIAN_POINT('',(14.4,49.4458289444115,108.)) ;
#42551=CARTESIAN_POINT('',(14.4,0.,108.)) ;
#42552=CARTESIAN_POINT('',(28.,43.2232576282723,108.)) ;
#42553=CARTESIAN_POINT('Origin',(0.,0.,108.)) ;
#42554=CARTESIAN_POINT('',(28.4,43.2232576282723,108.)) ;
#42555=CARTESIAN_POINT('',(28.,43.2232576282723,108.)) ;
#42556=CARTESIAN_POINT('',(28.4,42.9614943874163,108.)) ;
#42557=CARTESIAN_POINT('',(28.4,0.,108.)) ;
#42558=CARTESIAN_POINT('',(29.2316609175736,42.4,108.)) ;
#42559=CARTESIAN_POINT('Origin',(0.,0.,108.)) ;
#42560=CARTESIAN_POINT('',(29.8035232816525,42.4,108.)) ;
#42561=CARTESIAN_POINT('',(0.,42.4,108.)) ;
#42562=CARTESIAN_POINT('',(29.8035232816525,42.,108.)) ;
#42563=CARTESIAN_POINT('',(28.4,27.6,108.)) ;
#42564=CARTESIAN_POINT('',(0.,27.6,108.)) ;
#42565=CARTESIAN_POINT('',(28.4,0.,108.)) ;
#42566=CARTESIAN_POINT('',(28.4,13.6,108.)) ;
#42567=CARTESIAN_POINT('',(0.,13.6,108.)) ;
#42568=CARTESIAN_POINT('',(28.4,0.,108.)) ;
#42569=CARTESIAN_POINT('',(28.4,-0.4,108.)) ;
#42570=CARTESIAN_POINT('',(0.,-0.4,108.)) ;
#42571=CARTESIAN_POINT('',(28.4,0.,108.)) ;
#42572=CARTESIAN_POINT('',(28.4,-14.4,108.)) ;
#42573=CARTESIAN_POINT('',(0.,-14.4,108.)) ;
#42574=CARTESIAN_POINT('',(28.4,0.,108.)) ;
#42575=CARTESIAN_POINT('',(28.6302287800849,41.6,108.)) ;
#42576=CARTESIAN_POINT('Origin',(0.,0.,108.)) ;
#42577=CARTESIAN_POINT('',(28.4,41.6,108.)) ;
#42578=CARTESIAN_POINT('',(0.,41.6,108.)) ;
#42579=CARTESIAN_POINT('',(28.4,0.,108.)) ;
#42580=CARTESIAN_POINT('',(50.4984158167363,0.4,108.)) ;
#42581=CARTESIAN_POINT('',(0.,0.4,108.)) ;
#42582=CARTESIAN_POINT('Origin',(0.,0.,108.)) ;
#42583=CARTESIAN_POINT('',(48.6342471926933,-13.6,108.)) ;
#42584=CARTESIAN_POINT('',(0.,-13.6,108.)) ;
#42585=CARTESIAN_POINT('Origin',(0.,0.,108.)) ;
#42586=CARTESIAN_POINT('Origin',(0.,0.,108.)) ;
#42587=CARTESIAN_POINT('',(28.4,-28.4,108.)) ;
#42588=CARTESIAN_POINT('',(0.,-28.4,108.)) ;
#42589=CARTESIAN_POINT('',(28.4,-41.6,108.)) ;
#42590=CARTESIAN_POINT('',(28.4,0.,108.)) ;
#42591=CARTESIAN_POINT('',(0.,-41.6,108.)) ;
#42592=CARTESIAN_POINT('',(0.,14.4,108.)) ;
#42593=CARTESIAN_POINT('',(-28.4,41.6,108.)) ;
#42594=CARTESIAN_POINT('',(-28.6302287800849,41.6,108.)) ;
#42595=CARTESIAN_POINT('',(0.,41.6,108.)) ;
#42596=CARTESIAN_POINT('',(-41.6,28.6302287800849,108.)) ;
#42597=CARTESIAN_POINT('Origin',(0.,0.,108.)) ;
#42598=CARTESIAN_POINT('',(-41.6,28.4,108.)) ;
#42599=CARTESIAN_POINT('',(-41.6,0.,108.)) ;
#42600=CARTESIAN_POINT('',(-28.4,28.4,108.)) ;
#42601=CARTESIAN_POINT('',(0.,28.4,108.)) ;
#42602=CARTESIAN_POINT('',(-28.4,0.,108.)) ;
#42603=CARTESIAN_POINT('',(-41.6,27.6,108.)) ;
#42604=CARTESIAN_POINT('',(-41.6,14.4,108.)) ;
#42605=CARTESIAN_POINT('',(-41.6,0.,108.)) ;
#42606=CARTESIAN_POINT('',(-28.4,14.4,108.)) ;
#42607=CARTESIAN_POINT('',(0.,14.4,108.)) ;
#42608=CARTESIAN_POINT('',(-28.4,27.6,108.)) ;
#42609=CARTESIAN_POINT('',(-28.4,0.,108.)) ;
#42610=CARTESIAN_POINT('',(0.,27.6,108.)) ;
#42611=CARTESIAN_POINT('',(13.6,27.6,108.)) ;
#42612=CARTESIAN_POINT('',(0.4,27.6,108.)) ;
#42613=CARTESIAN_POINT('',(0.,27.6,108.)) ;
#42614=CARTESIAN_POINT('',(0.4,14.4,108.)) ;
#42615=CARTESIAN_POINT('',(0.4,0.,108.)) ;
#42616=CARTESIAN_POINT('',(13.6,14.4,108.)) ;
#42617=CARTESIAN_POINT('',(0.,14.4,108.)) ;
#42618=CARTESIAN_POINT('',(13.6,0.,108.)) ;
#42619=CARTESIAN_POINT('',(-0.4,27.6,108.)) ;
#42620=CARTESIAN_POINT('',(-13.6,27.6,108.)) ;
#42621=CARTESIAN_POINT('',(0.,27.6,108.)) ;
#42622=CARTESIAN_POINT('',(-13.6,14.4,108.)) ;
#42623=CARTESIAN_POINT('',(-13.6,0.,108.)) ;
#42624=CARTESIAN_POINT('',(-0.4,14.4,108.)) ;
#42625=CARTESIAN_POINT('',(0.,14.4,108.)) ;
#42626=CARTESIAN_POINT('',(-0.4,0.,108.)) ;
#42627=CARTESIAN_POINT('',(-14.4,27.6,108.)) ;
#42628=CARTESIAN_POINT('',(-27.6,27.6,108.)) ;
#42629=CARTESIAN_POINT('',(0.,27.6,108.)) ;
#42630=CARTESIAN_POINT('',(-27.6,14.4,108.)) ;
#42631=CARTESIAN_POINT('',(-27.6,0.,108.)) ;
#42632=CARTESIAN_POINT('',(-14.4,14.4,108.)) ;
#42633=CARTESIAN_POINT('',(0.,14.4,108.)) ;
#42634=CARTESIAN_POINT('',(-14.4,0.,108.)) ;
#42635=CARTESIAN_POINT('',(-42.4,14.4,108.)) ;
#42636=CARTESIAN_POINT('',(-42.4,27.4315511774307,108.)) ;
#42637=CARTESIAN_POINT('',(-42.4,0.,108.)) ;
#42638=CARTESIAN_POINT('',(-48.4034089708566,14.4,108.)) ;
#42639=CARTESIAN_POINT('Origin',(0.,0.,108.)) ;
#42640=CARTESIAN_POINT('',(0.,14.4,108.)) ;
#42641=CARTESIAN_POINT('',(-0.4,13.6,108.)) ;
#42642=CARTESIAN_POINT('',(-13.6,13.6,108.)) ;
#42643=CARTESIAN_POINT('',(0.,13.6,108.)) ;
#42644=CARTESIAN_POINT('',(-13.6,0.4,108.)) ;
#42645=CARTESIAN_POINT('',(-13.6,0.,108.)) ;
#42646=CARTESIAN_POINT('',(-0.4,0.4,108.)) ;
#42647=CARTESIAN_POINT('',(0.,0.4,108.)) ;
#42648=CARTESIAN_POINT('',(-0.4,0.,108.)) ;
#42649=CARTESIAN_POINT('',(-14.4,13.6,108.)) ;
#42650=CARTESIAN_POINT('',(-27.6,13.6,108.)) ;
#42651=CARTESIAN_POINT('',(0.,13.6,108.)) ;
#42652=CARTESIAN_POINT('',(-27.6,0.4,108.)) ;
#42653=CARTESIAN_POINT('',(-27.6,0.,108.)) ;
#42654=CARTESIAN_POINT('',(-14.4,0.4,108.)) ;
#42655=CARTESIAN_POINT('',(0.,0.4,108.)) ;
#42656=CARTESIAN_POINT('',(-14.4,0.,108.)) ;
#42657=CARTESIAN_POINT('',(-28.4,13.6,108.)) ;
#42658=CARTESIAN_POINT('',(-41.6,13.6,108.)) ;
#42659=CARTESIAN_POINT('',(0.,13.6,108.)) ;
#42660=CARTESIAN_POINT('',(-41.6,0.4,108.)) ;
#42661=CARTESIAN_POINT('',(-41.6,0.,108.)) ;
#42662=CARTESIAN_POINT('',(-28.4,0.4,108.)) ;
#42663=CARTESIAN_POINT('',(0.,0.4,108.)) ;
#42664=CARTESIAN_POINT('',(-28.4,0.,108.)) ;
#42665=CARTESIAN_POINT('',(-0.4,-0.4,108.)) ;
#42666=CARTESIAN_POINT('',(-13.6,-0.4,108.)) ;
#42667=CARTESIAN_POINT('',(0.,-0.4,108.)) ;
#42668=CARTESIAN_POINT('',(-13.6,-13.6,108.)) ;
#42669=CARTESIAN_POINT('',(-13.6,0.,108.)) ;
#42670=CARTESIAN_POINT('',(-0.4,-13.6,108.)) ;
#42671=CARTESIAN_POINT('',(0.,-13.6,108.)) ;
#42672=CARTESIAN_POINT('',(-0.4,0.,108.)) ;
#42673=CARTESIAN_POINT('',(-0.4,-14.4,108.)) ;
#42674=CARTESIAN_POINT('',(-13.6,-14.4,108.)) ;
#42675=CARTESIAN_POINT('',(0.,-14.4,108.)) ;
#42676=CARTESIAN_POINT('',(-13.6,-27.6,108.)) ;
#42677=CARTESIAN_POINT('',(-13.6,0.,108.)) ;
#42678=CARTESIAN_POINT('',(-0.4,-27.6,108.)) ;
#42679=CARTESIAN_POINT('',(0.,-27.6,108.)) ;
#42680=CARTESIAN_POINT('',(-0.4,0.,108.)) ;
#42681=CARTESIAN_POINT('',(-0.4,-28.4,108.)) ;
#42682=CARTESIAN_POINT('',(-13.6,-28.4,108.)) ;
#42683=CARTESIAN_POINT('',(0.,-28.4,108.)) ;
#42684=CARTESIAN_POINT('',(-13.6,-41.6,108.)) ;
#42685=CARTESIAN_POINT('',(-13.6,0.,108.)) ;
#42686=CARTESIAN_POINT('',(-0.4,-41.6,108.)) ;
#42687=CARTESIAN_POINT('',(0.,-41.6,108.)) ;
#42688=CARTESIAN_POINT('',(-0.4,0.,108.)) ;
#42689=CARTESIAN_POINT('',(-0.4,-50.4984158167363,108.)) ;
#42690=CARTESIAN_POINT('',(-0.4,-42.4,108.)) ;
#42691=CARTESIAN_POINT('',(-0.4,0.,108.)) ;
#42692=CARTESIAN_POINT('',(-13.6,-42.4,108.)) ;
#42693=CARTESIAN_POINT('',(0.,-42.4,108.)) ;
#42694=CARTESIAN_POINT('',(-13.6,-48.6342471926933,108.)) ;
#42695=CARTESIAN_POINT('',(-13.6,0.,108.)) ;
#42696=CARTESIAN_POINT('Origin',(0.,0.,108.)) ;
#42697=CARTESIAN_POINT('',(-42.4,-0.4,108.)) ;
#42698=CARTESIAN_POINT('',(-50.4984158167363,-0.4,108.)) ;
#42699=CARTESIAN_POINT('',(0.,-0.4,108.)) ;
#42700=CARTESIAN_POINT('',(-48.6342471926933,-13.6,108.)) ;
#42701=CARTESIAN_POINT('Origin',(0.,0.,108.)) ;
#42702=CARTESIAN_POINT('',(-42.4,-13.6,108.)) ;
#42703=CARTESIAN_POINT('',(0.,-13.6,108.)) ;
#42704=CARTESIAN_POINT('',(-42.4,0.,108.)) ;
#42705=CARTESIAN_POINT('',(-28.4,-28.4,108.)) ;
#42706=CARTESIAN_POINT('',(-41.6,-28.4,108.)) ;
#42707=CARTESIAN_POINT('',(0.,-28.4,108.)) ;
#42708=CARTESIAN_POINT('',(-41.6,-28.6302287800849,108.)) ;
#42709=CARTESIAN_POINT('',(-41.6,0.,108.)) ;
#42710=CARTESIAN_POINT('',(-28.6302287800849,-41.6,108.)) ;
#42711=CARTESIAN_POINT('Origin',(0.,0.,108.)) ;
#42712=CARTESIAN_POINT('',(-28.4,-41.6,108.)) ;
#42713=CARTESIAN_POINT('',(0.,-41.6,108.)) ;
#42714=CARTESIAN_POINT('',(-28.4,0.,108.)) ;
#42715=CARTESIAN_POINT('',(-42.4,-14.4,108.)) ;
#42716=CARTESIAN_POINT('',(-48.4034089708566,-14.4,108.)) ;
#42717=CARTESIAN_POINT('',(0.,-14.4,108.)) ;
#42718=CARTESIAN_POINT('',(-42.4,-27.4315511774307,108.)) ;
#42719=CARTESIAN_POINT('Origin',(0.,0.,108.)) ;
#42720=CARTESIAN_POINT('',(-42.4,0.,108.)) ;
#42721=CARTESIAN_POINT('',(-28.4,-14.4,108.)) ;
#42722=CARTESIAN_POINT('',(-41.6,-14.4,108.)) ;
#42723=CARTESIAN_POINT('',(0.,-14.4,108.)) ;
#42724=CARTESIAN_POINT('',(-41.6,-27.6,108.)) ;
#42725=CARTESIAN_POINT('',(-41.6,0.,108.)) ;
#42726=CARTESIAN_POINT('',(-28.4,-27.6,108.)) ;
#42727=CARTESIAN_POINT('',(0.,-27.6,108.)) ;
#42728=CARTESIAN_POINT('',(-28.4,0.,108.)) ;
#42729=CARTESIAN_POINT('',(-14.4,-42.4,108.)) ;
#42730=CARTESIAN_POINT('',(-27.4315511774307,-42.4,108.)) ;
#42731=CARTESIAN_POINT('',(0.,-42.4,108.)) ;
#42732=CARTESIAN_POINT('',(-14.4,-48.4034089708566,108.)) ;
#42733=CARTESIAN_POINT('Origin',(0.,0.,108.)) ;
#42734=CARTESIAN_POINT('',(-14.4,0.,108.)) ;
#42735=CARTESIAN_POINT('',(-14.4,-28.4,108.)) ;
#42736=CARTESIAN_POINT('',(-27.6,-28.4,108.)) ;
#42737=CARTESIAN_POINT('',(0.,-28.4,108.)) ;
#42738=CARTESIAN_POINT('',(-27.6,-41.6,108.)) ;
#42739=CARTESIAN_POINT('',(-27.6,0.,108.)) ;
#42740=CARTESIAN_POINT('',(-14.4,-41.6,108.)) ;
#42741=CARTESIAN_POINT('',(0.,-41.6,108.)) ;
#42742=CARTESIAN_POINT('',(-14.4,0.,108.)) ;
#42743=CARTESIAN_POINT('',(-14.4,-14.4,108.)) ;
#42744=CARTESIAN_POINT('',(-27.6,-14.4,108.)) ;
#42745=CARTESIAN_POINT('',(0.,-14.4,108.)) ;
#42746=CARTESIAN_POINT('',(-27.6,-27.6,108.)) ;
#42747=CARTESIAN_POINT('',(-27.6,0.,108.)) ;
#42748=CARTESIAN_POINT('',(-14.4,-27.6,108.)) ;
#42749=CARTESIAN_POINT('',(0.,-27.6,108.)) ;
#42750=CARTESIAN_POINT('',(-14.4,0.,108.)) ;
#42751=CARTESIAN_POINT('',(-28.4,-0.4,108.)) ;
#42752=CARTESIAN_POINT('',(-41.6,-0.4,108.)) ;
#42753=CARTESIAN_POINT('',(0.,-0.4,108.)) ;
#42754=CARTESIAN_POINT('',(-41.6,-13.6,108.)) ;
#42755=CARTESIAN_POINT('',(-41.6,0.,108.)) ;
#42756=CARTESIAN_POINT('',(-28.4,-13.6,108.)) ;
#42757=CARTESIAN_POINT('',(0.,-13.6,108.)) ;
#42758=CARTESIAN_POINT('',(-28.4,0.,108.)) ;
#42759=CARTESIAN_POINT('',(-14.4,-0.4,108.)) ;
#42760=CARTESIAN_POINT('',(-27.6,-0.4,108.)) ;
#42761=CARTESIAN_POINT('',(0.,-0.4,108.)) ;
#42762=CARTESIAN_POINT('',(-27.6,-13.6,108.)) ;
#42763=CARTESIAN_POINT('',(-27.6,0.,108.)) ;
#42764=CARTESIAN_POINT('',(-14.4,-13.6,108.)) ;
#42765=CARTESIAN_POINT('',(0.,-13.6,108.)) ;
#42766=CARTESIAN_POINT('',(-14.4,0.,108.)) ;
#42767=CARTESIAN_POINT('',(-42.4,13.6,108.)) ;
#42768=CARTESIAN_POINT('',(-48.6342471926933,13.6,108.)) ;
#42769=CARTESIAN_POINT('',(0.,13.6,108.)) ;
#42770=CARTESIAN_POINT('',(-50.4984158167363,0.4,108.)) ;
#42771=CARTESIAN_POINT('Origin',(0.,0.,108.)) ;
#42772=CARTESIAN_POINT('',(-42.4,0.4,108.)) ;
#42773=CARTESIAN_POINT('',(0.,0.4,108.)) ;
#42774=CARTESIAN_POINT('',(-42.4,0.,108.)) ;
#42775=CARTESIAN_POINT('',(13.6,-48.6342471926933,108.)) ;
#42776=CARTESIAN_POINT('',(13.6,-42.4,108.)) ;
#42777=CARTESIAN_POINT('',(13.6,0.,108.)) ;
#42778=CARTESIAN_POINT('',(0.4,-42.4,108.)) ;
#42779=CARTESIAN_POINT('',(0.,-42.4,108.)) ;
#42780=CARTESIAN_POINT('',(0.4,-50.4984158167363,108.)) ;
#42781=CARTESIAN_POINT('',(0.4,0.,108.)) ;
#42782=CARTESIAN_POINT('Origin',(0.,0.,108.)) ;
#42783=CARTESIAN_POINT('',(13.6,-28.4,108.)) ;
#42784=CARTESIAN_POINT('',(0.4,-28.4,108.)) ;
#42785=CARTESIAN_POINT('',(0.,-28.4,108.)) ;
#42786=CARTESIAN_POINT('',(0.4,-41.6,108.)) ;
#42787=CARTESIAN_POINT('',(0.4,0.,108.)) ;
#42788=CARTESIAN_POINT('',(13.6,-41.6,108.)) ;
#42789=CARTESIAN_POINT('',(0.,-41.6,108.)) ;
#42790=CARTESIAN_POINT('',(13.6,0.,108.)) ;
#42791=CARTESIAN_POINT('',(13.6,-14.4,108.)) ;
#42792=CARTESIAN_POINT('',(0.4,-14.4,108.)) ;
#42793=CARTESIAN_POINT('',(0.,-14.4,108.)) ;
#42794=CARTESIAN_POINT('',(0.4,-27.6,108.)) ;
#42795=CARTESIAN_POINT('',(0.4,0.,108.)) ;
#42796=CARTESIAN_POINT('',(13.6,-27.6,108.)) ;
#42797=CARTESIAN_POINT('',(0.,-27.6,108.)) ;
#42798=CARTESIAN_POINT('',(13.6,0.,108.)) ;
#42799=CARTESIAN_POINT('',(13.6,-0.4,108.)) ;
#42800=CARTESIAN_POINT('',(0.4,-0.4,108.)) ;
#42801=CARTESIAN_POINT('',(0.,-0.4,108.)) ;
#42802=CARTESIAN_POINT('',(0.4,-13.6,108.)) ;
#42803=CARTESIAN_POINT('',(0.4,0.,108.)) ;
#42804=CARTESIAN_POINT('',(13.6,-13.6,108.)) ;
#42805=CARTESIAN_POINT('',(0.,-13.6,108.)) ;
#42806=CARTESIAN_POINT('',(13.6,0.,108.)) ;
#42807=CARTESIAN_POINT('',(14.4,-48.4034089708566,108.)) ;
#42808=CARTESIAN_POINT('',(27.4315511774307,-42.4,108.)) ;
#42809=CARTESIAN_POINT('Origin',(0.,0.,108.)) ;
#42810=CARTESIAN_POINT('',(14.4,-42.4,108.)) ;
#42811=CARTESIAN_POINT('',(0.,-42.4,108.)) ;
#42812=CARTESIAN_POINT('',(14.4,0.,108.)) ;
#42813=CARTESIAN_POINT('',(13.6,13.6,108.)) ;
#42814=CARTESIAN_POINT('',(0.4,13.6,108.)) ;
#42815=CARTESIAN_POINT('',(0.,13.6,108.)) ;
#42816=CARTESIAN_POINT('',(0.4,0.4,108.)) ;
#42817=CARTESIAN_POINT('',(0.4,0.,108.)) ;
#42818=CARTESIAN_POINT('',(13.6,0.4,108.)) ;
#42819=CARTESIAN_POINT('',(0.,0.4,108.)) ;
#42820=CARTESIAN_POINT('',(13.6,0.,108.)) ;
#42821=CARTESIAN_POINT('',(27.6,-28.4,108.)) ;
#42822=CARTESIAN_POINT('',(14.4,-28.4,108.)) ;
#42823=CARTESIAN_POINT('',(0.,-28.4,108.)) ;
#42824=CARTESIAN_POINT('',(14.4,-41.6,108.)) ;
#42825=CARTESIAN_POINT('',(14.4,0.,108.)) ;
#42826=CARTESIAN_POINT('',(27.6,-41.6,108.)) ;
#42827=CARTESIAN_POINT('',(0.,-41.6,108.)) ;
#42828=CARTESIAN_POINT('',(27.6,0.,108.)) ;
#42829=CARTESIAN_POINT('',(27.6,-14.4,108.)) ;
#42830=CARTESIAN_POINT('',(14.4,-14.4,108.)) ;
#42831=CARTESIAN_POINT('',(0.,-14.4,108.)) ;
#42832=CARTESIAN_POINT('',(14.4,-27.6,108.)) ;
#42833=CARTESIAN_POINT('',(14.4,0.,108.)) ;
#42834=CARTESIAN_POINT('',(27.6,-27.6,108.)) ;
#42835=CARTESIAN_POINT('',(0.,-27.6,108.)) ;
#42836=CARTESIAN_POINT('',(27.6,0.,108.)) ;
#42837=CARTESIAN_POINT('',(27.6,-0.4,108.)) ;
#42838=CARTESIAN_POINT('',(14.4,-0.4,108.)) ;
#42839=CARTESIAN_POINT('',(0.,-0.4,108.)) ;
#42840=CARTESIAN_POINT('',(14.4,-13.6,108.)) ;
#42841=CARTESIAN_POINT('',(14.4,0.,108.)) ;
#42842=CARTESIAN_POINT('',(27.6,-13.6,108.)) ;
#42843=CARTESIAN_POINT('',(0.,-13.6,108.)) ;
#42844=CARTESIAN_POINT('',(27.6,0.,108.)) ;
#42845=CARTESIAN_POINT('',(27.6,13.6,108.)) ;
#42846=CARTESIAN_POINT('',(14.4,13.6,108.)) ;
#42847=CARTESIAN_POINT('',(0.,13.6,108.)) ;
#42848=CARTESIAN_POINT('',(14.4,0.4,108.)) ;
#42849=CARTESIAN_POINT('',(14.4,0.,108.)) ;
#42850=CARTESIAN_POINT('',(27.6,0.4,108.)) ;
#42851=CARTESIAN_POINT('',(0.,0.4,108.)) ;
#42852=CARTESIAN_POINT('',(27.6,0.,108.)) ;
#42853=CARTESIAN_POINT('',(27.6,27.6,108.)) ;
#42854=CARTESIAN_POINT('',(14.4,27.6,108.)) ;
#42855=CARTESIAN_POINT('',(0.,27.6,108.)) ;
#42856=CARTESIAN_POINT('',(14.4,14.4,108.)) ;
#42857=CARTESIAN_POINT('',(14.4,0.,108.)) ;
#42858=CARTESIAN_POINT('',(27.6,14.4,108.)) ;
#42859=CARTESIAN_POINT('',(0.,14.4,108.)) ;
#42860=CARTESIAN_POINT('',(27.6,0.,108.)) ;
#42861=CARTESIAN_POINT('',(-14.4,41.6,108.)) ;
#42862=CARTESIAN_POINT('',(-27.6,41.6,108.)) ;
#42863=CARTESIAN_POINT('',(0.,41.6,108.)) ;
#42864=CARTESIAN_POINT('',(-27.6,28.4,108.)) ;
#42865=CARTESIAN_POINT('',(-27.6,0.,108.)) ;
#42866=CARTESIAN_POINT('',(-14.4,28.4,108.)) ;
#42867=CARTESIAN_POINT('',(0.,28.4,108.)) ;
#42868=CARTESIAN_POINT('',(-14.4,0.,108.)) ;
#42869=CARTESIAN_POINT('',(-0.4,41.6,108.)) ;
#42870=CARTESIAN_POINT('',(-13.6,41.6,108.)) ;
#42871=CARTESIAN_POINT('',(0.,41.6,108.)) ;
#42872=CARTESIAN_POINT('',(-13.6,28.4,108.)) ;
#42873=CARTESIAN_POINT('',(-13.6,0.,108.)) ;
#42874=CARTESIAN_POINT('',(-0.4,28.4,108.)) ;
#42875=CARTESIAN_POINT('',(0.,28.4,108.)) ;
#42876=CARTESIAN_POINT('',(-0.4,0.,108.)) ;
#42877=CARTESIAN_POINT('',(13.6,41.6,108.)) ;
#42878=CARTESIAN_POINT('',(0.4,41.6,108.)) ;
#42879=CARTESIAN_POINT('',(0.,41.6,108.)) ;
#42880=CARTESIAN_POINT('',(0.4,28.4,108.)) ;
#42881=CARTESIAN_POINT('',(0.4,0.,108.)) ;
#42882=CARTESIAN_POINT('',(13.6,28.4,108.)) ;
#42883=CARTESIAN_POINT('',(0.,28.4,108.)) ;
#42884=CARTESIAN_POINT('',(13.6,0.,108.)) ;
#42885=CARTESIAN_POINT('',(14.4,42.4,108.)) ;
#42886=CARTESIAN_POINT('',(27.4315511774307,42.4,108.)) ;
#42887=CARTESIAN_POINT('',(0.,42.4,108.)) ;
#42888=CARTESIAN_POINT('',(14.4,48.4034089708566,108.)) ;
#42889=CARTESIAN_POINT('Origin',(0.,0.,108.)) ;
#42890=CARTESIAN_POINT('',(14.4,0.,108.)) ;
#42891=CARTESIAN_POINT('',(-14.4,42.4,108.)) ;
#42892=CARTESIAN_POINT('',(-14.4,48.4034089708566,108.)) ;
#42893=CARTESIAN_POINT('',(-14.4,0.,108.)) ;
#42894=CARTESIAN_POINT('',(-27.4315511774307,42.4,108.)) ;
#42895=CARTESIAN_POINT('Origin',(0.,0.,108.)) ;
#42896=CARTESIAN_POINT('',(0.,42.4,108.)) ;
#42897=CARTESIAN_POINT('',(-0.4,42.4,108.)) ;
#42898=CARTESIAN_POINT('',(-0.4,50.4984158167363,108.)) ;
#42899=CARTESIAN_POINT('',(-0.4,0.,108.)) ;
#42900=CARTESIAN_POINT('',(-13.6,48.6342471926933,108.)) ;
#42901=CARTESIAN_POINT('Origin',(0.,0.,108.)) ;
#42902=CARTESIAN_POINT('',(-13.6,42.4,108.)) ;
#42903=CARTESIAN_POINT('',(-13.6,0.,108.)) ;
#42904=CARTESIAN_POINT('',(0.,42.4,108.)) ;
#42905=CARTESIAN_POINT('',(13.6,42.4,108.)) ;
#42906=CARTESIAN_POINT('',(13.6,48.6342471926933,108.)) ;
#42907=CARTESIAN_POINT('',(13.6,0.,108.)) ;
#42908=CARTESIAN_POINT('',(0.4,50.4984158167363,108.)) ;
#42909=CARTESIAN_POINT('Origin',(0.,0.,108.)) ;
#42910=CARTESIAN_POINT('',(0.4,42.4,108.)) ;
#42911=CARTESIAN_POINT('',(0.4,0.,108.)) ;
#42912=CARTESIAN_POINT('',(0.,42.4,108.)) ;
#42913=CARTESIAN_POINT('',(14.4,41.6,108.)) ;
#42914=CARTESIAN_POINT('',(14.4,28.4,108.)) ;
#42915=CARTESIAN_POINT('',(14.4,0.,108.)) ;
#42916=CARTESIAN_POINT('',(27.6,28.4,108.)) ;
#42917=CARTESIAN_POINT('',(0.,28.4,108.)) ;
#42918=CARTESIAN_POINT('',(27.6,41.6,108.)) ;
#42919=CARTESIAN_POINT('',(27.6,0.,108.)) ;
#42920=CARTESIAN_POINT('',(0.,41.6,108.)) ;
#42921=CARTESIAN_POINT('Origin',(0.,0.,108.3)) ;
#42922=CARTESIAN_POINT('',(29.8035232816525,-42.,108.3)) ;
#42923=CARTESIAN_POINT('Origin',(0.,0.,108.3)) ;
#42924=CARTESIAN_POINT('',(42.9614943874163,-28.4,108.3)) ;
#42925=CARTESIAN_POINT('Origin',(29.8035232816525,42.,108.3)) ;
#42926=CARTESIAN_POINT('',(29.8035232816525,42.4,108.3)) ;
#42927=CARTESIAN_POINT('Origin',(0.,41.6,108.3)) ;
#42928=CARTESIAN_POINT('',(-28.4,41.6,108.3)) ;
#42929=CARTESIAN_POINT('',(-28.6302287800849,41.6,108.3)) ;
#42930=CARTESIAN_POINT('Origin',(0.,41.6,108.3)) ;
#42931=CARTESIAN_POINT('',(-14.4,41.6,108.3)) ;
#42932=CARTESIAN_POINT('',(-27.6,41.6,108.3)) ;
#42933=CARTESIAN_POINT('Origin',(0.,41.6,108.3)) ;
#42934=CARTESIAN_POINT('',(-0.4,41.6,108.3)) ;
#42935=CARTESIAN_POINT('',(-13.6,41.6,108.3)) ;
#42936=CARTESIAN_POINT('Origin',(0.,41.6,108.3)) ;
#42937=CARTESIAN_POINT('',(28.4,41.6,108.3)) ;
#42938=CARTESIAN_POINT('',(28.6302287800849,41.6,108.3)) ;
#42939=CARTESIAN_POINT('Origin',(0.,41.6,108.3)) ;
#42940=CARTESIAN_POINT('',(14.4,41.6,108.3)) ;
#42941=CARTESIAN_POINT('',(27.6,41.6,108.3)) ;
#42942=CARTESIAN_POINT('Origin',(0.,41.6,108.3)) ;
#42943=CARTESIAN_POINT('',(13.6,41.6,108.3)) ;
#42944=CARTESIAN_POINT('',(0.4,41.6,108.3)) ;
#42945=CARTESIAN_POINT('Origin',(0.,42.4,108.3)) ;
#42946=CARTESIAN_POINT('',(-29.2316609175736,42.4,108.3)) ;
#42947=CARTESIAN_POINT('',(-29.8035232816525,42.4,108.3)) ;
#42948=CARTESIAN_POINT('Origin',(0.,42.4,108.3)) ;
#42949=CARTESIAN_POINT('',(-14.4,42.4,108.3)) ;
#42950=CARTESIAN_POINT('',(-27.4315511774307,42.4,108.3)) ;
#42951=CARTESIAN_POINT('Origin',(0.,42.4,108.3)) ;
#42952=CARTESIAN_POINT('',(-0.4,42.4,108.3)) ;
#42953=CARTESIAN_POINT('',(-13.6,42.4,108.3)) ;
#42954=CARTESIAN_POINT('Origin',(0.,42.4,108.3)) ;
#42955=CARTESIAN_POINT('',(13.6,42.4,108.3)) ;
#42956=CARTESIAN_POINT('',(0.4,42.4,108.3)) ;
#42957=CARTESIAN_POINT('Origin',(0.,42.4,108.3)) ;
#42958=CARTESIAN_POINT('',(29.2316609175736,42.4,108.3)) ;
#42959=CARTESIAN_POINT('Origin',(-29.8035232816525,42.,108.3)) ;
#42960=CARTESIAN_POINT('',(-29.8035232816525,42.,108.3)) ;
#42961=CARTESIAN_POINT('Origin',(0.,42.4,108.3)) ;
#42962=CARTESIAN_POINT('',(14.4,42.4,108.3)) ;
#42963=CARTESIAN_POINT('',(27.4315511774307,42.4,108.3)) ;
#42964=CARTESIAN_POINT('Origin',(14.4,0.,108.3)) ;
#42965=CARTESIAN_POINT('',(14.4,48.4034089708566,108.3)) ;
#42966=CARTESIAN_POINT('Origin',(13.6,0.,108.3)) ;
#42967=CARTESIAN_POINT('',(13.6,28.4,108.3)) ;
#42968=CARTESIAN_POINT('Origin',(27.6,0.,108.3)) ;
#42969=CARTESIAN_POINT('',(27.6,28.4,108.3)) ;
#42970=CARTESIAN_POINT('Origin',(0.,0.,108.3)) ;
#42971=CARTESIAN_POINT('Origin',(0.,0.,108.3)) ;
#42972=CARTESIAN_POINT('',(28.4,42.9614943874163,108.3)) ;
#42973=CARTESIAN_POINT('Origin',(0.4,0.,108.3)) ;
#42974=CARTESIAN_POINT('',(0.4,50.4984158167363,108.3)) ;
#42975=CARTESIAN_POINT('Origin',(-0.4,0.,108.3)) ;
#42976=CARTESIAN_POINT('',(-0.4,28.4,108.3)) ;
#42977=CARTESIAN_POINT('Origin',(-13.6,0.,108.3)) ;
#42978=CARTESIAN_POINT('',(-13.6,48.6342471926933,108.3)) ;
#42979=CARTESIAN_POINT('Origin',(-14.4,0.,108.3)) ;
#42980=CARTESIAN_POINT('',(-14.4,28.4,108.3)) ;
#42981=CARTESIAN_POINT('Origin',(-28.4,0.,108.3)) ;
#42982=CARTESIAN_POINT('',(-28.4,28.4,108.3)) ;
#42983=CARTESIAN_POINT('Origin',(0.,0.,108.3)) ;
#42984=CARTESIAN_POINT('',(-14.4,48.4034089708566,108.3)) ;
#42985=CARTESIAN_POINT('Origin',(0.,0.,108.3)) ;
#42986=CARTESIAN_POINT('',(-28.4,42.9614943874163,108.3)) ;
#42987=CARTESIAN_POINT('Origin',(0.,0.,108.3)) ;
#42988=CARTESIAN_POINT('',(-42.,29.8035232816525,108.3)) ;
#42989=CARTESIAN_POINT('Origin',(28.,-43.2232576282723,108.3)) ;
#42990=CARTESIAN_POINT('',(28.,-43.2232576282723,108.3)) ;
#42991=CARTESIAN_POINT('',(28.4,-43.2232576282723,108.3)) ;
#42992=CARTESIAN_POINT('Origin',(28.4,0.,108.3)) ;
#42993=CARTESIAN_POINT('',(28.4,43.2232576282723,108.3)) ;
#42994=CARTESIAN_POINT('Origin',(28.4,0.,108.3)) ;
#42995=CARTESIAN_POINT('',(28.4,-42.9614943874163,108.3)) ;
#42996=CARTESIAN_POINT('Origin',(28.4,0.,108.3)) ;
#42997=CARTESIAN_POINT('',(28.4,-28.4,108.3)) ;
#42998=CARTESIAN_POINT('',(28.4,-41.6,108.3)) ;
#42999=CARTESIAN_POINT('Origin',(28.4,0.,108.3)) ;
#43000=CARTESIAN_POINT('',(28.4,-14.4,108.3)) ;
#43001=CARTESIAN_POINT('Origin',(28.4,0.,108.3)) ;
#43002=CARTESIAN_POINT('',(28.4,-0.4,108.3)) ;
#43003=CARTESIAN_POINT('Origin',(28.4,0.,108.3)) ;
#43004=CARTESIAN_POINT('',(28.4,13.6,108.3)) ;
#43005=CARTESIAN_POINT('Origin',(28.4,0.,108.3)) ;
#43006=CARTESIAN_POINT('Origin',(27.6,0.,108.3)) ;
#43007=CARTESIAN_POINT('',(27.6,-28.4,108.3)) ;
#43008=CARTESIAN_POINT('',(27.6,-41.6,108.3)) ;
#43009=CARTESIAN_POINT('Origin',(27.6,0.,108.3)) ;
#43010=CARTESIAN_POINT('',(27.6,-14.4,108.3)) ;
#43011=CARTESIAN_POINT('',(27.6,-27.6,108.3)) ;
#43012=CARTESIAN_POINT('Origin',(27.6,0.,108.3)) ;
#43013=CARTESIAN_POINT('',(27.6,-0.4,108.3)) ;
#43014=CARTESIAN_POINT('',(27.6,-13.6,108.3)) ;
#43015=CARTESIAN_POINT('Origin',(27.6,0.,108.3)) ;
#43016=CARTESIAN_POINT('',(27.6,13.6,108.3)) ;
#43017=CARTESIAN_POINT('',(27.6,0.4,108.3)) ;
#43018=CARTESIAN_POINT('Origin',(27.6,0.,108.3)) ;
#43019=CARTESIAN_POINT('',(27.6,27.6,108.3)) ;
#43020=CARTESIAN_POINT('',(27.6,14.4,108.3)) ;
#43021=CARTESIAN_POINT('Origin',(28.,43.2232576282723,108.3)) ;
#43022=CARTESIAN_POINT('',(28.,43.2232576282723,108.3)) ;
#43023=CARTESIAN_POINT('Origin',(28.4,0.,108.3)) ;
#43024=CARTESIAN_POINT('',(28.4,27.6,108.3)) ;
#43025=CARTESIAN_POINT('Origin',(0.,27.6,108.3)) ;
#43026=CARTESIAN_POINT('Origin',(0.,28.4,108.3)) ;
#43027=CARTESIAN_POINT('',(14.4,28.4,108.3)) ;
#43028=CARTESIAN_POINT('Origin',(0.,0.,108.3)) ;
#43029=CARTESIAN_POINT('',(14.4,49.4458289444115,108.3)) ;
#43030=CARTESIAN_POINT('Origin',(0.,13.6,108.3)) ;
#43031=CARTESIAN_POINT('Origin',(0.,14.4,108.3)) ;
#43032=CARTESIAN_POINT('',(14.4,14.4,108.3)) ;
#43033=CARTESIAN_POINT('Origin',(0.,-0.4,108.3)) ;
#43034=CARTESIAN_POINT('Origin',(0.,0.4,108.3)) ;
#43035=CARTESIAN_POINT('',(14.4,0.4,108.3)) ;
#43036=CARTESIAN_POINT('Origin',(0.,-14.4,108.3)) ;
#43037=CARTESIAN_POINT('Origin',(0.,-13.6,108.3)) ;
#43038=CARTESIAN_POINT('',(14.4,-13.6,108.3)) ;
#43039=CARTESIAN_POINT('Origin',(0.,-28.4,108.3)) ;
#43040=CARTESIAN_POINT('Origin',(0.,-27.6,108.3)) ;
#43041=CARTESIAN_POINT('',(14.4,-27.6,108.3)) ;
#43042=CARTESIAN_POINT('Origin',(0.,0.,108.3)) ;
#43043=CARTESIAN_POINT('',(29.2316609175736,-42.4,108.3)) ;
#43044=CARTESIAN_POINT('Origin',(0.,-41.6,108.3)) ;
#43045=CARTESIAN_POINT('',(14.4,-41.6,108.3)) ;
#43046=CARTESIAN_POINT('Origin',(43.2232576282723,28.,108.3)) ;
#43047=CARTESIAN_POINT('',(43.2232576282723,28.,108.3)) ;
#43048=CARTESIAN_POINT('',(43.2232576282723,28.4,108.3)) ;
#43049=CARTESIAN_POINT('Origin',(0.,28.4,108.3)) ;
#43050=CARTESIAN_POINT('',(-42.9614943874163,28.4,108.3)) ;
#43051=CARTESIAN_POINT('',(-43.2232576282723,28.4,108.3)) ;
#43052=CARTESIAN_POINT('Origin',(0.,28.4,108.3)) ;
#43053=CARTESIAN_POINT('',(-27.6,28.4,108.3)) ;
#43054=CARTESIAN_POINT('Origin',(0.,28.4,108.3)) ;
#43055=CARTESIAN_POINT('',(-13.6,28.4,108.3)) ;
#43056=CARTESIAN_POINT('Origin',(0.,28.4,108.3)) ;
#43057=CARTESIAN_POINT('',(-41.6,28.4,108.3)) ;
#43058=CARTESIAN_POINT('Origin',(0.,28.4,108.3)) ;
#43059=CARTESIAN_POINT('Origin',(0.,28.4,108.3)) ;
#43060=CARTESIAN_POINT('',(0.4,28.4,108.3)) ;
#43061=CARTESIAN_POINT('Origin',(0.,27.6,108.3)) ;
#43062=CARTESIAN_POINT('',(-41.6,27.6,108.3)) ;
#43063=CARTESIAN_POINT('',(-28.4,27.6,108.3)) ;
#43064=CARTESIAN_POINT('Origin',(0.,27.6,108.3)) ;
#43065=CARTESIAN_POINT('',(-14.4,27.6,108.3)) ;
#43066=CARTESIAN_POINT('',(-27.6,27.6,108.3)) ;
#43067=CARTESIAN_POINT('Origin',(0.,27.6,108.3)) ;
#43068=CARTESIAN_POINT('',(14.4,27.6,108.3)) ;
#43069=CARTESIAN_POINT('Origin',(0.,27.6,108.3)) ;
#43070=CARTESIAN_POINT('',(-0.4,27.6,108.3)) ;
#43071=CARTESIAN_POINT('',(-13.6,27.6,108.3)) ;
#43072=CARTESIAN_POINT('Origin',(0.,27.6,108.3)) ;
#43073=CARTESIAN_POINT('',(13.6,27.6,108.3)) ;
#43074=CARTESIAN_POINT('',(0.4,27.6,108.3)) ;
#43075=CARTESIAN_POINT('Origin',(-43.2232576282723,28.,108.3)) ;
#43076=CARTESIAN_POINT('',(-43.2232576282723,28.,108.3)) ;
#43077=CARTESIAN_POINT('Origin',(14.4,0.,108.3)) ;
#43078=CARTESIAN_POINT('Origin',(13.6,0.,108.3)) ;
#43079=CARTESIAN_POINT('',(13.6,48.6342471926933,108.3)) ;
#43080=CARTESIAN_POINT('Origin',(13.6,0.,108.3)) ;
#43081=CARTESIAN_POINT('',(13.6,14.4,108.3)) ;
#43082=CARTESIAN_POINT('Origin',(0.4,0.,108.3)) ;
#43083=CARTESIAN_POINT('Origin',(-0.4,0.,108.3)) ;
#43084=CARTESIAN_POINT('',(-0.4,14.4,108.3)) ;
#43085=CARTESIAN_POINT('Origin',(0.,0.,108.3)) ;
#43086=CARTESIAN_POINT('Origin',(0.,0.,108.3)) ;
#43087=CARTESIAN_POINT('',(49.4458289444115,14.4,108.3)) ;
#43088=CARTESIAN_POINT('Origin',(-41.6,0.,108.3)) ;
#43089=CARTESIAN_POINT('',(-41.6,28.6302287800849,108.3)) ;
#43090=CARTESIAN_POINT('Origin',(0.,0.,108.3)) ;
#43091=CARTESIAN_POINT('',(-42.4,29.2316609175736,108.3)) ;
#43092=CARTESIAN_POINT('Origin',(0.,0.,108.3)) ;
#43093=CARTESIAN_POINT('',(-49.4458289444115,14.4,108.3)) ;
#43094=CARTESIAN_POINT('Origin',(-13.6,0.,108.3)) ;
#43095=CARTESIAN_POINT('Origin',(-14.4,0.,108.3)) ;
#43096=CARTESIAN_POINT('',(-14.4,14.4,108.3)) ;
#43097=CARTESIAN_POINT('Origin',(-27.6,0.,108.3)) ;
#43098=CARTESIAN_POINT('Origin',(-28.4,0.,108.3)) ;
#43099=CARTESIAN_POINT('',(-28.4,14.4,108.3)) ;
#43100=CARTESIAN_POINT('Origin',(14.,-49.5605690039975,108.3)) ;
#43101=CARTESIAN_POINT('',(14.,-49.5605690039975,108.3)) ;
#43102=CARTESIAN_POINT('',(14.4,-49.5605690039975,108.3)) ;
#43103=CARTESIAN_POINT('Origin',(14.4,0.,108.3)) ;
#43104=CARTESIAN_POINT('',(14.4,49.5605690039975,108.3)) ;
#43105=CARTESIAN_POINT('Origin',(14.4,0.,108.3)) ;
#43106=CARTESIAN_POINT('',(14.4,-48.4034089708566,108.3)) ;
#43107=CARTESIAN_POINT('',(14.4,-42.4,108.3)) ;
#43108=CARTESIAN_POINT('Origin',(14.4,0.,108.3)) ;
#43109=CARTESIAN_POINT('',(14.4,-28.4,108.3)) ;
#43110=CARTESIAN_POINT('Origin',(14.4,0.,108.3)) ;
#43111=CARTESIAN_POINT('',(14.4,-14.4,108.3)) ;
#43112=CARTESIAN_POINT('Origin',(14.4,0.,108.3)) ;
#43113=CARTESIAN_POINT('',(14.4,-0.4,108.3)) ;
#43114=CARTESIAN_POINT('Origin',(14.4,0.,108.3)) ;
#43115=CARTESIAN_POINT('',(14.4,-49.4458289444115,108.3)) ;
#43116=CARTESIAN_POINT('Origin',(14.4,0.,108.3)) ;
#43117=CARTESIAN_POINT('Origin',(13.6,0.,108.3)) ;
#43118=CARTESIAN_POINT('',(13.6,-28.4,108.3)) ;
#43119=CARTESIAN_POINT('',(13.6,-41.6,108.3)) ;
#43120=CARTESIAN_POINT('Origin',(13.6,0.,108.3)) ;
#43121=CARTESIAN_POINT('',(13.6,-14.4,108.3)) ;
#43122=CARTESIAN_POINT('',(13.6,-27.6,108.3)) ;
#43123=CARTESIAN_POINT('Origin',(13.6,0.,108.3)) ;
#43124=CARTESIAN_POINT('',(13.6,-0.4,108.3)) ;
#43125=CARTESIAN_POINT('',(13.6,-13.6,108.3)) ;
#43126=CARTESIAN_POINT('Origin',(13.6,0.,108.3)) ;
#43127=CARTESIAN_POINT('',(13.6,13.6,108.3)) ;
#43128=CARTESIAN_POINT('',(13.6,0.4,108.3)) ;
#43129=CARTESIAN_POINT('Origin',(13.6,0.,108.3)) ;
#43130=CARTESIAN_POINT('',(13.6,-48.6342471926933,108.3)) ;
#43131=CARTESIAN_POINT('',(13.6,-42.4,108.3)) ;
#43132=CARTESIAN_POINT('Origin',(14.,49.5605690039975,108.3)) ;
#43133=CARTESIAN_POINT('',(14.,49.5605690039975,108.3)) ;
#43134=CARTESIAN_POINT('Origin',(14.4,0.,108.3)) ;
#43135=CARTESIAN_POINT('',(14.4,13.6,108.3)) ;
#43136=CARTESIAN_POINT('Origin',(0.,13.6,108.3)) ;
#43137=CARTESIAN_POINT('Origin',(0.,14.4,108.3)) ;
#43138=CARTESIAN_POINT('Origin',(0.,14.4,108.3)) ;
#43139=CARTESIAN_POINT('',(0.4,14.4,108.3)) ;
#43140=CARTESIAN_POINT('Origin',(0.,0.,108.3)) ;
#43141=CARTESIAN_POINT('',(0.4,51.4984465785134,108.3)) ;
#43142=CARTESIAN_POINT('Origin',(0.,0.,108.3)) ;
#43143=CARTESIAN_POINT('Origin',(0.,0.,108.3)) ;
#43144=CARTESIAN_POINT('',(27.4315511774307,-42.4,108.3)) ;
#43145=CARTESIAN_POINT('Origin',(0.,0.,108.3)) ;
#43146=CARTESIAN_POINT('',(0.4,-50.4984158167363,108.3)) ;
#43147=CARTESIAN_POINT('Origin',(0.,-0.4,108.3)) ;
#43148=CARTESIAN_POINT('Origin',(0.,0.4,108.3)) ;
#43149=CARTESIAN_POINT('',(0.4,0.4,108.3)) ;
#43150=CARTESIAN_POINT('Origin',(0.,-14.4,108.3)) ;
#43151=CARTESIAN_POINT('Origin',(0.,-13.6,108.3)) ;
#43152=CARTESIAN_POINT('',(0.4,-13.6,108.3)) ;
#43153=CARTESIAN_POINT('Origin',(0.,-28.4,108.3)) ;
#43154=CARTESIAN_POINT('Origin',(0.,-27.6,108.3)) ;
#43155=CARTESIAN_POINT('',(0.4,-27.6,108.3)) ;
#43156=CARTESIAN_POINT('Origin',(0.,-42.4,108.3)) ;
#43157=CARTESIAN_POINT('Origin',(0.,-41.6,108.3)) ;
#43158=CARTESIAN_POINT('',(0.4,-41.6,108.3)) ;
#43159=CARTESIAN_POINT('Origin',(49.5605690039975,14.,108.3)) ;
#43160=CARTESIAN_POINT('',(49.5605690039975,14.,108.3)) ;
#43161=CARTESIAN_POINT('',(49.5605690039975,14.4,108.3)) ;
#43162=CARTESIAN_POINT('Origin',(0.,13.6,108.3)) ;
#43163=CARTESIAN_POINT('',(-42.4,13.6,108.3)) ;
#43164=CARTESIAN_POINT('',(-48.6342471926933,13.6,108.3)) ;
#43165=CARTESIAN_POINT('Origin',(0.,13.6,108.3)) ;
#43166=CARTESIAN_POINT('',(-28.4,13.6,108.3)) ;
#43167=CARTESIAN_POINT('',(-41.6,13.6,108.3)) ;
#43168=CARTESIAN_POINT('Origin',(0.,13.6,108.3)) ;
#43169=CARTESIAN_POINT('',(-14.4,13.6,108.3)) ;
#43170=CARTESIAN_POINT('',(-27.6,13.6,108.3)) ;
#43171=CARTESIAN_POINT('Origin',(0.,13.6,108.3)) ;
#43172=CARTESIAN_POINT('',(0.4,13.6,108.3)) ;
#43173=CARTESIAN_POINT('Origin',(0.,13.6,108.3)) ;
#43174=CARTESIAN_POINT('',(-0.4,13.6,108.3)) ;
#43175=CARTESIAN_POINT('',(-13.6,13.6,108.3)) ;
#43176=CARTESIAN_POINT('Origin',(0.,14.4,108.3)) ;
#43177=CARTESIAN_POINT('',(-49.5605690039975,14.4,108.3)) ;
#43178=CARTESIAN_POINT('Origin',(0.,14.4,108.3)) ;
#43179=CARTESIAN_POINT('',(-42.4,14.4,108.3)) ;
#43180=CARTESIAN_POINT('',(-48.4034089708566,14.4,108.3)) ;
#43181=CARTESIAN_POINT('Origin',(0.,14.4,108.3)) ;
#43182=CARTESIAN_POINT('',(-41.6,14.4,108.3)) ;
#43183=CARTESIAN_POINT('Origin',(0.,14.4,108.3)) ;
#43184=CARTESIAN_POINT('',(-27.6,14.4,108.3)) ;
#43185=CARTESIAN_POINT('Origin',(0.,14.4,108.3)) ;
#43186=CARTESIAN_POINT('',(-13.6,14.4,108.3)) ;
#43187=CARTESIAN_POINT('Origin',(0.,14.4,108.3)) ;
#43188=CARTESIAN_POINT('Origin',(-49.5605690039975,14.,108.3)) ;
#43189=CARTESIAN_POINT('',(-49.5605690039975,14.,108.3)) ;
#43190=CARTESIAN_POINT('Origin',(0.4,0.,108.3)) ;
#43191=CARTESIAN_POINT('Origin',(-0.4,0.,108.3)) ;
#43192=CARTESIAN_POINT('',(-0.4,50.4984158167363,108.3)) ;
#43193=CARTESIAN_POINT('Origin',(-0.4,0.,108.3)) ;
#43194=CARTESIAN_POINT('',(-0.4,0.4,108.3)) ;
#43195=CARTESIAN_POINT('Origin',(0.,0.,108.3)) ;
#43196=CARTESIAN_POINT('Origin',(0.,0.,108.3)) ;
#43197=CARTESIAN_POINT('',(50.4984158167363,0.4,108.3)) ;
#43198=CARTESIAN_POINT('Origin',(0.,0.,108.3)) ;
#43199=CARTESIAN_POINT('',(51.4984465785134,0.4,108.3)) ;
#43200=CARTESIAN_POINT('Origin',(-13.6,0.,108.3)) ;
#43201=CARTESIAN_POINT('Origin',(-14.4,0.,108.3)) ;
#43202=CARTESIAN_POINT('',(-14.4,0.4,108.3)) ;
#43203=CARTESIAN_POINT('Origin',(-27.6,0.,108.3)) ;
#43204=CARTESIAN_POINT('Origin',(-28.4,0.,108.3)) ;
#43205=CARTESIAN_POINT('',(-28.4,0.4,108.3)) ;
#43206=CARTESIAN_POINT('Origin',(-41.6,0.,108.3)) ;
#43207=CARTESIAN_POINT('Origin',(-42.4,0.,108.3)) ;
#43208=CARTESIAN_POINT('',(-42.4,0.4,108.3)) ;
#43209=CARTESIAN_POINT('Origin',(0.,0.,108.3)) ;
#43210=CARTESIAN_POINT('',(-42.4,27.4315511774307,108.3)) ;
#43211=CARTESIAN_POINT('Origin',(0.,0.,108.3)) ;
#43212=CARTESIAN_POINT('',(-51.4984465785134,0.4,108.3)) ;
#43213=CARTESIAN_POINT('Origin',(0.4,0.,108.3)) ;
#43214=CARTESIAN_POINT('',(0.4,51.5,108.3)) ;
#43215=CARTESIAN_POINT('Origin',(0.4,0.,108.3)) ;
#43216=CARTESIAN_POINT('',(0.4,-42.4,108.3)) ;
#43217=CARTESIAN_POINT('Origin',(0.4,0.,108.3)) ;
#43218=CARTESIAN_POINT('',(0.4,-28.4,108.3)) ;
#43219=CARTESIAN_POINT('Origin',(0.4,0.,108.3)) ;
#43220=CARTESIAN_POINT('',(0.4,-51.4984465785134,108.3)) ;
#43221=CARTESIAN_POINT('',(0.4,-51.5,108.3)) ;
#43222=CARTESIAN_POINT('Origin',(0.4,0.,108.3)) ;
#43223=CARTESIAN_POINT('',(0.4,-14.4,108.3)) ;
#43224=CARTESIAN_POINT('Origin',(0.4,0.,108.3)) ;
#43225=CARTESIAN_POINT('Origin',(0.4,0.,108.3)) ;
#43226=CARTESIAN_POINT('',(0.4,-0.4,108.3)) ;
#43227=CARTESIAN_POINT('Origin',(-0.4,0.,108.3)) ;
#43228=CARTESIAN_POINT('',(-0.4,-51.4984465785134,108.3)) ;
#43229=CARTESIAN_POINT('',(-0.4,-51.5,108.3)) ;
#43230=CARTESIAN_POINT('Origin',(-0.4,0.,108.3)) ;
#43231=CARTESIAN_POINT('',(-0.4,-28.4,108.3)) ;
#43232=CARTESIAN_POINT('',(-0.4,-41.6,108.3)) ;
#43233=CARTESIAN_POINT('Origin',(-0.4,0.,108.3)) ;
#43234=CARTESIAN_POINT('',(-0.4,-14.4,108.3)) ;
#43235=CARTESIAN_POINT('',(-0.4,-27.6,108.3)) ;
#43236=CARTESIAN_POINT('Origin',(-0.4,0.,108.3)) ;
#43237=CARTESIAN_POINT('',(-0.4,-50.4984158167363,108.3)) ;
#43238=CARTESIAN_POINT('',(-0.4,-42.4,108.3)) ;
#43239=CARTESIAN_POINT('Origin',(-0.4,0.,108.3)) ;
#43240=CARTESIAN_POINT('',(-0.4,-0.4,108.3)) ;
#43241=CARTESIAN_POINT('',(-0.4,-13.6,108.3)) ;
#43242=CARTESIAN_POINT('Origin',(-0.4,0.,108.3)) ;
#43243=CARTESIAN_POINT('',(-0.4,51.4984465785134,108.3)) ;
#43244=CARTESIAN_POINT('',(-0.4,51.5,108.3)) ;
#43245=CARTESIAN_POINT('Origin',(0.,-51.5,108.3)) ;
#43246=CARTESIAN_POINT('Origin',(0.,51.5,108.3)) ;
#43247=CARTESIAN_POINT('Origin',(0.,0.4,108.3)) ;
#43248=CARTESIAN_POINT('',(-13.6,0.4,108.3)) ;
#43249=CARTESIAN_POINT('Origin',(0.,-0.4,108.3)) ;
#43250=CARTESIAN_POINT('',(-13.6,-0.4,108.3)) ;
#43251=CARTESIAN_POINT('Origin',(0.,-0.4,108.3)) ;
#43252=CARTESIAN_POINT('Origin',(0.,0.,108.3)) ;
#43253=CARTESIAN_POINT('Origin',(0.,0.,108.3)) ;
#43254=CARTESIAN_POINT('',(-14.,49.5605690039975,108.3)) ;
#43255=CARTESIAN_POINT('Origin',(0.,-14.4,108.3)) ;
#43256=CARTESIAN_POINT('Origin',(0.,-13.6,108.3)) ;
#43257=CARTESIAN_POINT('',(-13.6,-13.6,108.3)) ;
#43258=CARTESIAN_POINT('Origin',(0.,0.,108.3)) ;
#43259=CARTESIAN_POINT('Origin',(0.,0.,108.3)) ;
#43260=CARTESIAN_POINT('',(-14.,-49.5605690039975,108.3)) ;
#43261=CARTESIAN_POINT('Origin',(0.,0.,108.3)) ;
#43262=CARTESIAN_POINT('',(-13.6,-48.6342471926933,108.3)) ;
#43263=CARTESIAN_POINT('Origin',(0.,-28.4,108.3)) ;
#43264=CARTESIAN_POINT('Origin',(0.,-27.6,108.3)) ;
#43265=CARTESIAN_POINT('',(-13.6,-27.6,108.3)) ;
#43266=CARTESIAN_POINT('Origin',(0.,-42.4,108.3)) ;
#43267=CARTESIAN_POINT('Origin',(0.,-41.6,108.3)) ;
#43268=CARTESIAN_POINT('',(-13.6,-41.6,108.3)) ;
#43269=CARTESIAN_POINT('Origin',(0.,0.4,108.3)) ;
#43270=CARTESIAN_POINT('',(-51.5,0.4,108.3)) ;
#43271=CARTESIAN_POINT('Origin',(0.,0.4,108.3)) ;
#43272=CARTESIAN_POINT('',(-50.4984158167363,0.4,108.3)) ;
#43273=CARTESIAN_POINT('Origin',(0.,0.4,108.3)) ;
#43274=CARTESIAN_POINT('',(-41.6,0.4,108.3)) ;
#43275=CARTESIAN_POINT('Origin',(0.,0.4,108.3)) ;
#43276=CARTESIAN_POINT('',(51.5,0.4,108.3)) ;
#43277=CARTESIAN_POINT('Origin',(0.,0.4,108.3)) ;
#43278=CARTESIAN_POINT('',(-27.6,0.4,108.3)) ;
#43279=CARTESIAN_POINT('Origin',(0.,0.4,108.3)) ;
#43280=CARTESIAN_POINT('Origin',(0.,-0.4,108.3)) ;
#43281=CARTESIAN_POINT('',(51.4984465785134,-0.4,108.3)) ;
#43282=CARTESIAN_POINT('',(51.5,-0.4,108.3)) ;
#43283=CARTESIAN_POINT('Origin',(0.,-0.4,108.3)) ;
#43284=CARTESIAN_POINT('',(-51.4984465785134,-0.4,108.3)) ;
#43285=CARTESIAN_POINT('',(-51.5,-0.4,108.3)) ;
#43286=CARTESIAN_POINT('Origin',(0.,-0.4,108.3)) ;
#43287=CARTESIAN_POINT('',(-42.4,-0.4,108.3)) ;
#43288=CARTESIAN_POINT('',(-50.4984158167363,-0.4,108.3)) ;
#43289=CARTESIAN_POINT('Origin',(0.,-0.4,108.3)) ;
#43290=CARTESIAN_POINT('',(-28.4,-0.4,108.3)) ;
#43291=CARTESIAN_POINT('',(-41.6,-0.4,108.3)) ;
#43292=CARTESIAN_POINT('Origin',(0.,-0.4,108.3)) ;
#43293=CARTESIAN_POINT('',(-14.4,-0.4,108.3)) ;
#43294=CARTESIAN_POINT('',(-27.6,-0.4,108.3)) ;
#43295=CARTESIAN_POINT('Origin',(-51.5,0.,108.3)) ;
#43296=CARTESIAN_POINT('Origin',(51.5,0.,108.3)) ;
#43297=CARTESIAN_POINT('Origin',(-14.4,0.,108.3)) ;
#43298=CARTESIAN_POINT('',(-14.4,-13.6,108.3)) ;
#43299=CARTESIAN_POINT('Origin',(-13.6,0.,108.3)) ;
#43300=CARTESIAN_POINT('Origin',(-13.6,0.,108.3)) ;
#43301=CARTESIAN_POINT('Origin',(-27.6,0.,108.3)) ;
#43302=CARTESIAN_POINT('Origin',(-28.4,0.,108.3)) ;
#43303=CARTESIAN_POINT('',(-28.4,-13.6,108.3)) ;
#43304=CARTESIAN_POINT('Origin',(0.,0.,108.3)) ;
#43305=CARTESIAN_POINT('',(48.6342471926933,-13.6,108.3)) ;
#43306=CARTESIAN_POINT('Origin',(-41.6,0.,108.3)) ;
#43307=CARTESIAN_POINT('Origin',(-42.4,0.,108.3)) ;
#43308=CARTESIAN_POINT('',(-42.4,-13.6,108.3)) ;
#43309=CARTESIAN_POINT('Origin',(0.,0.,108.3)) ;
#43310=CARTESIAN_POINT('',(-48.6342471926933,-13.6,108.3)) ;
#43311=CARTESIAN_POINT('Origin',(0.,0.,108.3)) ;
#43312=CARTESIAN_POINT('Origin',(0.,0.,108.3)) ;
#43313=CARTESIAN_POINT('',(-49.5605690039975,-14.,108.3)) ;
#43314=CARTESIAN_POINT('Origin',(-14.,49.5605690039975,108.3)) ;
#43315=CARTESIAN_POINT('',(-14.4,49.5605690039975,108.3)) ;
#43316=CARTESIAN_POINT('Origin',(-14.4,0.,108.3)) ;
#43317=CARTESIAN_POINT('',(-14.4,-49.4458289444115,108.3)) ;
#43318=CARTESIAN_POINT('',(-14.4,-49.5605690039975,108.3)) ;
#43319=CARTESIAN_POINT('Origin',(-14.4,0.,108.3)) ;
#43320=CARTESIAN_POINT('',(-14.4,-42.4,108.3)) ;
#43321=CARTESIAN_POINT('',(-14.4,-48.4034089708566,108.3)) ;
#43322=CARTESIAN_POINT('Origin',(-14.4,0.,108.3)) ;
#43323=CARTESIAN_POINT('',(-14.4,-28.4,108.3)) ;
#43324=CARTESIAN_POINT('',(-14.4,-41.6,108.3)) ;
#43325=CARTESIAN_POINT('Origin',(-14.4,0.,108.3)) ;
#43326=CARTESIAN_POINT('',(-14.4,49.4458289444115,108.3)) ;
#43327=CARTESIAN_POINT('Origin',(-14.4,0.,108.3)) ;
#43328=CARTESIAN_POINT('',(-14.4,-14.4,108.3)) ;
#43329=CARTESIAN_POINT('',(-14.4,-27.6,108.3)) ;
#43330=CARTESIAN_POINT('Origin',(-14.4,0.,108.3)) ;
#43331=CARTESIAN_POINT('Origin',(-13.6,0.,108.3)) ;
#43332=CARTESIAN_POINT('',(-13.6,-42.4,108.3)) ;
#43333=CARTESIAN_POINT('Origin',(-13.6,0.,108.3)) ;
#43334=CARTESIAN_POINT('',(-13.6,-28.4,108.3)) ;
#43335=CARTESIAN_POINT('Origin',(-14.,-49.5605690039975,108.3)) ;
#43336=CARTESIAN_POINT('Origin',(-13.6,0.,108.3)) ;
#43337=CARTESIAN_POINT('',(-13.6,-14.4,108.3)) ;
#43338=CARTESIAN_POINT('Origin',(0.,-14.4,108.3)) ;
#43339=CARTESIAN_POINT('Origin',(0.,-13.6,108.3)) ;
#43340=CARTESIAN_POINT('Origin',(0.,-13.6,108.3)) ;
#43341=CARTESIAN_POINT('',(-27.6,-13.6,108.3)) ;
#43342=CARTESIAN_POINT('Origin',(0.,-28.4,108.3)) ;
#43343=CARTESIAN_POINT('Origin',(0.,-27.6,108.3)) ;
#43344=CARTESIAN_POINT('',(-27.6,-27.6,108.3)) ;
#43345=CARTESIAN_POINT('Origin',(0.,0.,108.3)) ;
#43346=CARTESIAN_POINT('',(-28.,43.2232576282723,108.3)) ;
#43347=CARTESIAN_POINT('Origin',(0.,-41.6,108.3)) ;
#43348=CARTESIAN_POINT('',(-27.6,-41.6,108.3)) ;
#43349=CARTESIAN_POINT('Origin',(0.,-42.4,108.3)) ;
#43350=CARTESIAN_POINT('Origin',(0.,0.,108.3)) ;
#43351=CARTESIAN_POINT('',(-28.,-43.2232576282723,108.3)) ;
#43352=CARTESIAN_POINT('Origin',(0.,0.,108.3)) ;
#43353=CARTESIAN_POINT('',(-27.4315511774307,-42.4,108.3)) ;
#43354=CARTESIAN_POINT('Origin',(-49.5605690039975,-14.,108.3)) ;
#43355=CARTESIAN_POINT('',(-49.5605690039975,-14.4,108.3)) ;
#43356=CARTESIAN_POINT('Origin',(0.,-13.6,108.3)) ;
#43357=CARTESIAN_POINT('Origin',(0.,-13.6,108.3)) ;
#43358=CARTESIAN_POINT('',(-41.6,-13.6,108.3)) ;
#43359=CARTESIAN_POINT('Origin',(0.,-14.4,108.3)) ;
#43360=CARTESIAN_POINT('',(-49.4458289444115,-14.4,108.3)) ;
#43361=CARTESIAN_POINT('Origin',(0.,-14.4,108.3)) ;
#43362=CARTESIAN_POINT('',(-42.4,-14.4,108.3)) ;
#43363=CARTESIAN_POINT('',(-48.4034089708566,-14.4,108.3)) ;
#43364=CARTESIAN_POINT('Origin',(0.,-14.4,108.3)) ;
#43365=CARTESIAN_POINT('',(49.4458289444115,-14.4,108.3)) ;
#43366=CARTESIAN_POINT('',(49.5605690039975,-14.4,108.3)) ;
#43367=CARTESIAN_POINT('Origin',(0.,-14.4,108.3)) ;
#43368=CARTESIAN_POINT('',(-28.4,-14.4,108.3)) ;
#43369=CARTESIAN_POINT('',(-41.6,-14.4,108.3)) ;
#43370=CARTESIAN_POINT('Origin',(0.,-14.4,108.3)) ;
#43371=CARTESIAN_POINT('',(-27.6,-14.4,108.3)) ;
#43372=CARTESIAN_POINT('Origin',(49.5605690039975,-14.,108.3)) ;
#43373=CARTESIAN_POINT('',(49.5605690039975,-14.,108.3)) ;
#43374=CARTESIAN_POINT('Origin',(-27.6,0.,108.3)) ;
#43375=CARTESIAN_POINT('Origin',(-28.4,0.,108.3)) ;
#43376=CARTESIAN_POINT('',(-28.4,-27.6,108.3)) ;
#43377=CARTESIAN_POINT('Origin',(0.,0.,108.3)) ;
#43378=CARTESIAN_POINT('Origin',(0.,0.,108.3)) ;
#43379=CARTESIAN_POINT('',(43.2232576282723,-28.,108.3)) ;
#43380=CARTESIAN_POINT('Origin',(0.,0.,108.3)) ;
#43381=CARTESIAN_POINT('Origin',(-41.6,0.,108.3)) ;
#43382=CARTESIAN_POINT('Origin',(-42.4,0.,108.3)) ;
#43383=CARTESIAN_POINT('',(-42.4,-27.4315511774307,108.3)) ;
#43384=CARTESIAN_POINT('Origin',(0.,0.,108.3)) ;
#43385=CARTESIAN_POINT('',(-43.2232576282723,-28.,108.3)) ;
#43386=CARTESIAN_POINT('Origin',(0.,0.,108.3)) ;
#43387=CARTESIAN_POINT('Origin',(-28.,43.2232576282723,108.3)) ;
#43388=CARTESIAN_POINT('',(-28.4,43.2232576282723,108.3)) ;
#43389=CARTESIAN_POINT('Origin',(-27.6,0.,108.3)) ;
#43390=CARTESIAN_POINT('Origin',(-28.4,0.,108.3)) ;
#43391=CARTESIAN_POINT('',(-28.4,-42.9614943874163,108.3)) ;
#43392=CARTESIAN_POINT('',(-28.4,-43.2232576282723,108.3)) ;
#43393=CARTESIAN_POINT('Origin',(-28.4,0.,108.3)) ;
#43394=CARTESIAN_POINT('Origin',(-28.4,0.,108.3)) ;
#43395=CARTESIAN_POINT('',(-28.4,-28.4,108.3)) ;
#43396=CARTESIAN_POINT('',(-28.4,-41.6,108.3)) ;
#43397=CARTESIAN_POINT('Origin',(-28.,-43.2232576282723,108.3)) ;
#43398=CARTESIAN_POINT('Origin',(-27.6,0.,108.3)) ;
#43399=CARTESIAN_POINT('',(-27.6,-28.4,108.3)) ;
#43400=CARTESIAN_POINT('Origin',(0.,-28.4,108.3)) ;
#43401=CARTESIAN_POINT('Origin',(0.,-27.6,108.3)) ;
#43402=CARTESIAN_POINT('',(-41.6,-27.6,108.3)) ;
#43403=CARTESIAN_POINT('Origin',(0.,0.,108.3)) ;
#43404=CARTESIAN_POINT('Origin',(0.,-41.6,108.3)) ;
#43405=CARTESIAN_POINT('',(-28.6302287800849,-41.6,108.3)) ;
#43406=CARTESIAN_POINT('Origin',(0.,0.,108.3)) ;
#43407=CARTESIAN_POINT('',(-29.2316609175736,-42.4,108.3)) ;
#43408=CARTESIAN_POINT('Origin',(-43.2232576282723,-28.,108.3)) ;
#43409=CARTESIAN_POINT('',(-43.2232576282723,-28.4,108.3)) ;
#43410=CARTESIAN_POINT('Origin',(0.,-28.4,108.3)) ;
#43411=CARTESIAN_POINT('',(43.2232576282723,-28.4,108.3)) ;
#43412=CARTESIAN_POINT('Origin',(0.,-28.4,108.3)) ;
#43413=CARTESIAN_POINT('',(-42.9614943874163,-28.4,108.3)) ;
#43414=CARTESIAN_POINT('Origin',(0.,-28.4,108.3)) ;
#43415=CARTESIAN_POINT('',(-41.6,-28.4,108.3)) ;
#43416=CARTESIAN_POINT('Origin',(43.2232576282723,-28.,108.3)) ;
#43417=CARTESIAN_POINT('Origin',(-41.6,0.,108.3)) ;
#43418=CARTESIAN_POINT('',(-41.6,-28.6302287800849,108.3)) ;
#43419=CARTESIAN_POINT('Origin',(-41.6,0.,108.3)) ;
#43420=CARTESIAN_POINT('Origin',(0.,0.,108.3)) ;
#43421=CARTESIAN_POINT('',(-42.4,-29.2316609175736,108.3)) ;
#43422=CARTESIAN_POINT('Origin',(-42.,29.8035232816525,108.3)) ;
#43423=CARTESIAN_POINT('',(-42.4,29.8035232816525,108.3)) ;
#43424=CARTESIAN_POINT('Origin',(-42.4,0.,108.3)) ;
#43425=CARTESIAN_POINT('Origin',(-42.4,0.,108.3)) ;
#43426=CARTESIAN_POINT('Origin',(-42.4,0.,108.3)) ;
#43427=CARTESIAN_POINT('',(-42.4,-29.8035232816525,108.3)) ;
#43428=CARTESIAN_POINT('Origin',(-42.,-29.8035232816525,108.3)) ;
#43429=CARTESIAN_POINT('',(-42.,-29.8035232816525,108.3)) ;
#43430=CARTESIAN_POINT('Origin',(0.,0.,108.3)) ;
#43431=CARTESIAN_POINT('',(-29.8035232816525,-42.,108.3)) ;
#43432=CARTESIAN_POINT('Origin',(0.,0.,108.3)) ;
#43433=CARTESIAN_POINT('Origin',(0.,-41.6,108.3)) ;
#43434=CARTESIAN_POINT('Origin',(-29.8035232816525,-42.,108.3)) ;
#43435=CARTESIAN_POINT('',(-29.8035232816525,-42.4,108.3)) ;
#43436=CARTESIAN_POINT('Origin',(0.,-42.4,108.3)) ;
#43437=CARTESIAN_POINT('',(29.8035232816525,-42.4,108.3)) ;
#43438=CARTESIAN_POINT('Origin',(0.,-42.4,108.3)) ;
#43439=CARTESIAN_POINT('Origin',(0.,-42.4,108.3)) ;
#43440=CARTESIAN_POINT('Origin',(29.8035232816525,-42.,108.3)) ;
#50340=UNCERTAINTY_MEASURE_WITH_UNIT(LENGTH_MEASURE(0.001),#50441,
'DISTANCE_ACCURACY_VALUE',
'Maximum model space distance between geometric entities at asserted c
onnectivities') ;
#50387=UNCERTAINTY_MEASURE_WITH_UNIT(LENGTH_MEASURE(0.001),#50441,
'DISTANCE_ACCURACY_VALUE',
'Maximum model space distance between geometric entities at asserted c
onnectivities') ;
#50393=(
GEOMETRIC_REPRESENTATION_CONTEXT(3)
GLOBAL_UNCERTAINTY_ASSIGNED_CONTEXT((#50340))
GLOBAL_UNIT_ASSIGNED_CONTEXT((#50441,#50443,#50444))
REPRESENTATION_CONTEXT('','3D')
) ;
#50440=(
GEOMETRIC_REPRESENTATION_CONTEXT(3)
GLOBAL_UNCERTAINTY_ASSIGNED_CONTEXT((#50387))
GLOBAL_UNIT_ASSIGNED_CONTEXT((#50441,#50443,#50444))
REPRESENTATION_CONTEXT('','3D')
) ;
#50441=(
LENGTH_UNIT()
NAMED_UNIT(*)
SI_UNIT(.CENTI.,.METRE.)
) ;
#50443=(
NAMED_UNIT(*)
PLANE_ANGLE_UNIT()
SI_UNIT($,.RADIAN.)
) ;
#50444=(
NAMED_UNIT(*)
SI_UNIT($,.STERADIAN.)
SOLID_ANGLE_UNIT()
) ;
#50450=SHAPE_DEFINITION_REPRESENTATION(#50502,#50624) ;
#50502=PRODUCT_DEFINITION_SHAPE('',$,#50677) ;
#50624=SHAPE_REPRESENTATION('',(#29339),#50393) ;
#50671=PRODUCT_DEFINITION_CONTEXT('part definition',#50829,'design') ;
#50677=PRODUCT_DEFINITION('HOPPER_SIEVE_GRID','HOPPER_SIEVE_GRID',
#50729,#50671) ;
#50729=PRODUCT_DEFINITION_FORMATION('',$,#50836) ;
#50829=APPLICATION_CONTEXT(
'Core Data for Automotive Mechanical Design Process') ;
#50830=PRODUCT_CONTEXT('part definition',#50829,'mechanical') ;
#50836=PRODUCT('HOPPER_SIEVE_GRID','HOPPER_SIEVE_GRID',$,(#50830)) ;
#50885=PRESENTATION_STYLE_ASSIGNMENT((#50892)) ;
#50892=SURFACE_STYLE_USAGE(.BOTH.,#50899) ;
#50899=SURFACE_SIDE_STYLE('',(#50906)) ;
#50906=SURFACE_STYLE_FILL_AREA(#50913) ;
#50913=FILL_AREA_STYLE('Steel - Galvanized (Small)',(#50920)) ;
#50920=FILL_AREA_STYLE_COLOUR('Steel - Galvanized (Small)',#50927) ;
#50927=COLOUR_RGB('Steel - Galvanized (Small)', 0.09019608, 0.27058824, 0.51372549) ;
ENDSEC;
END-ISO-10303-21;
